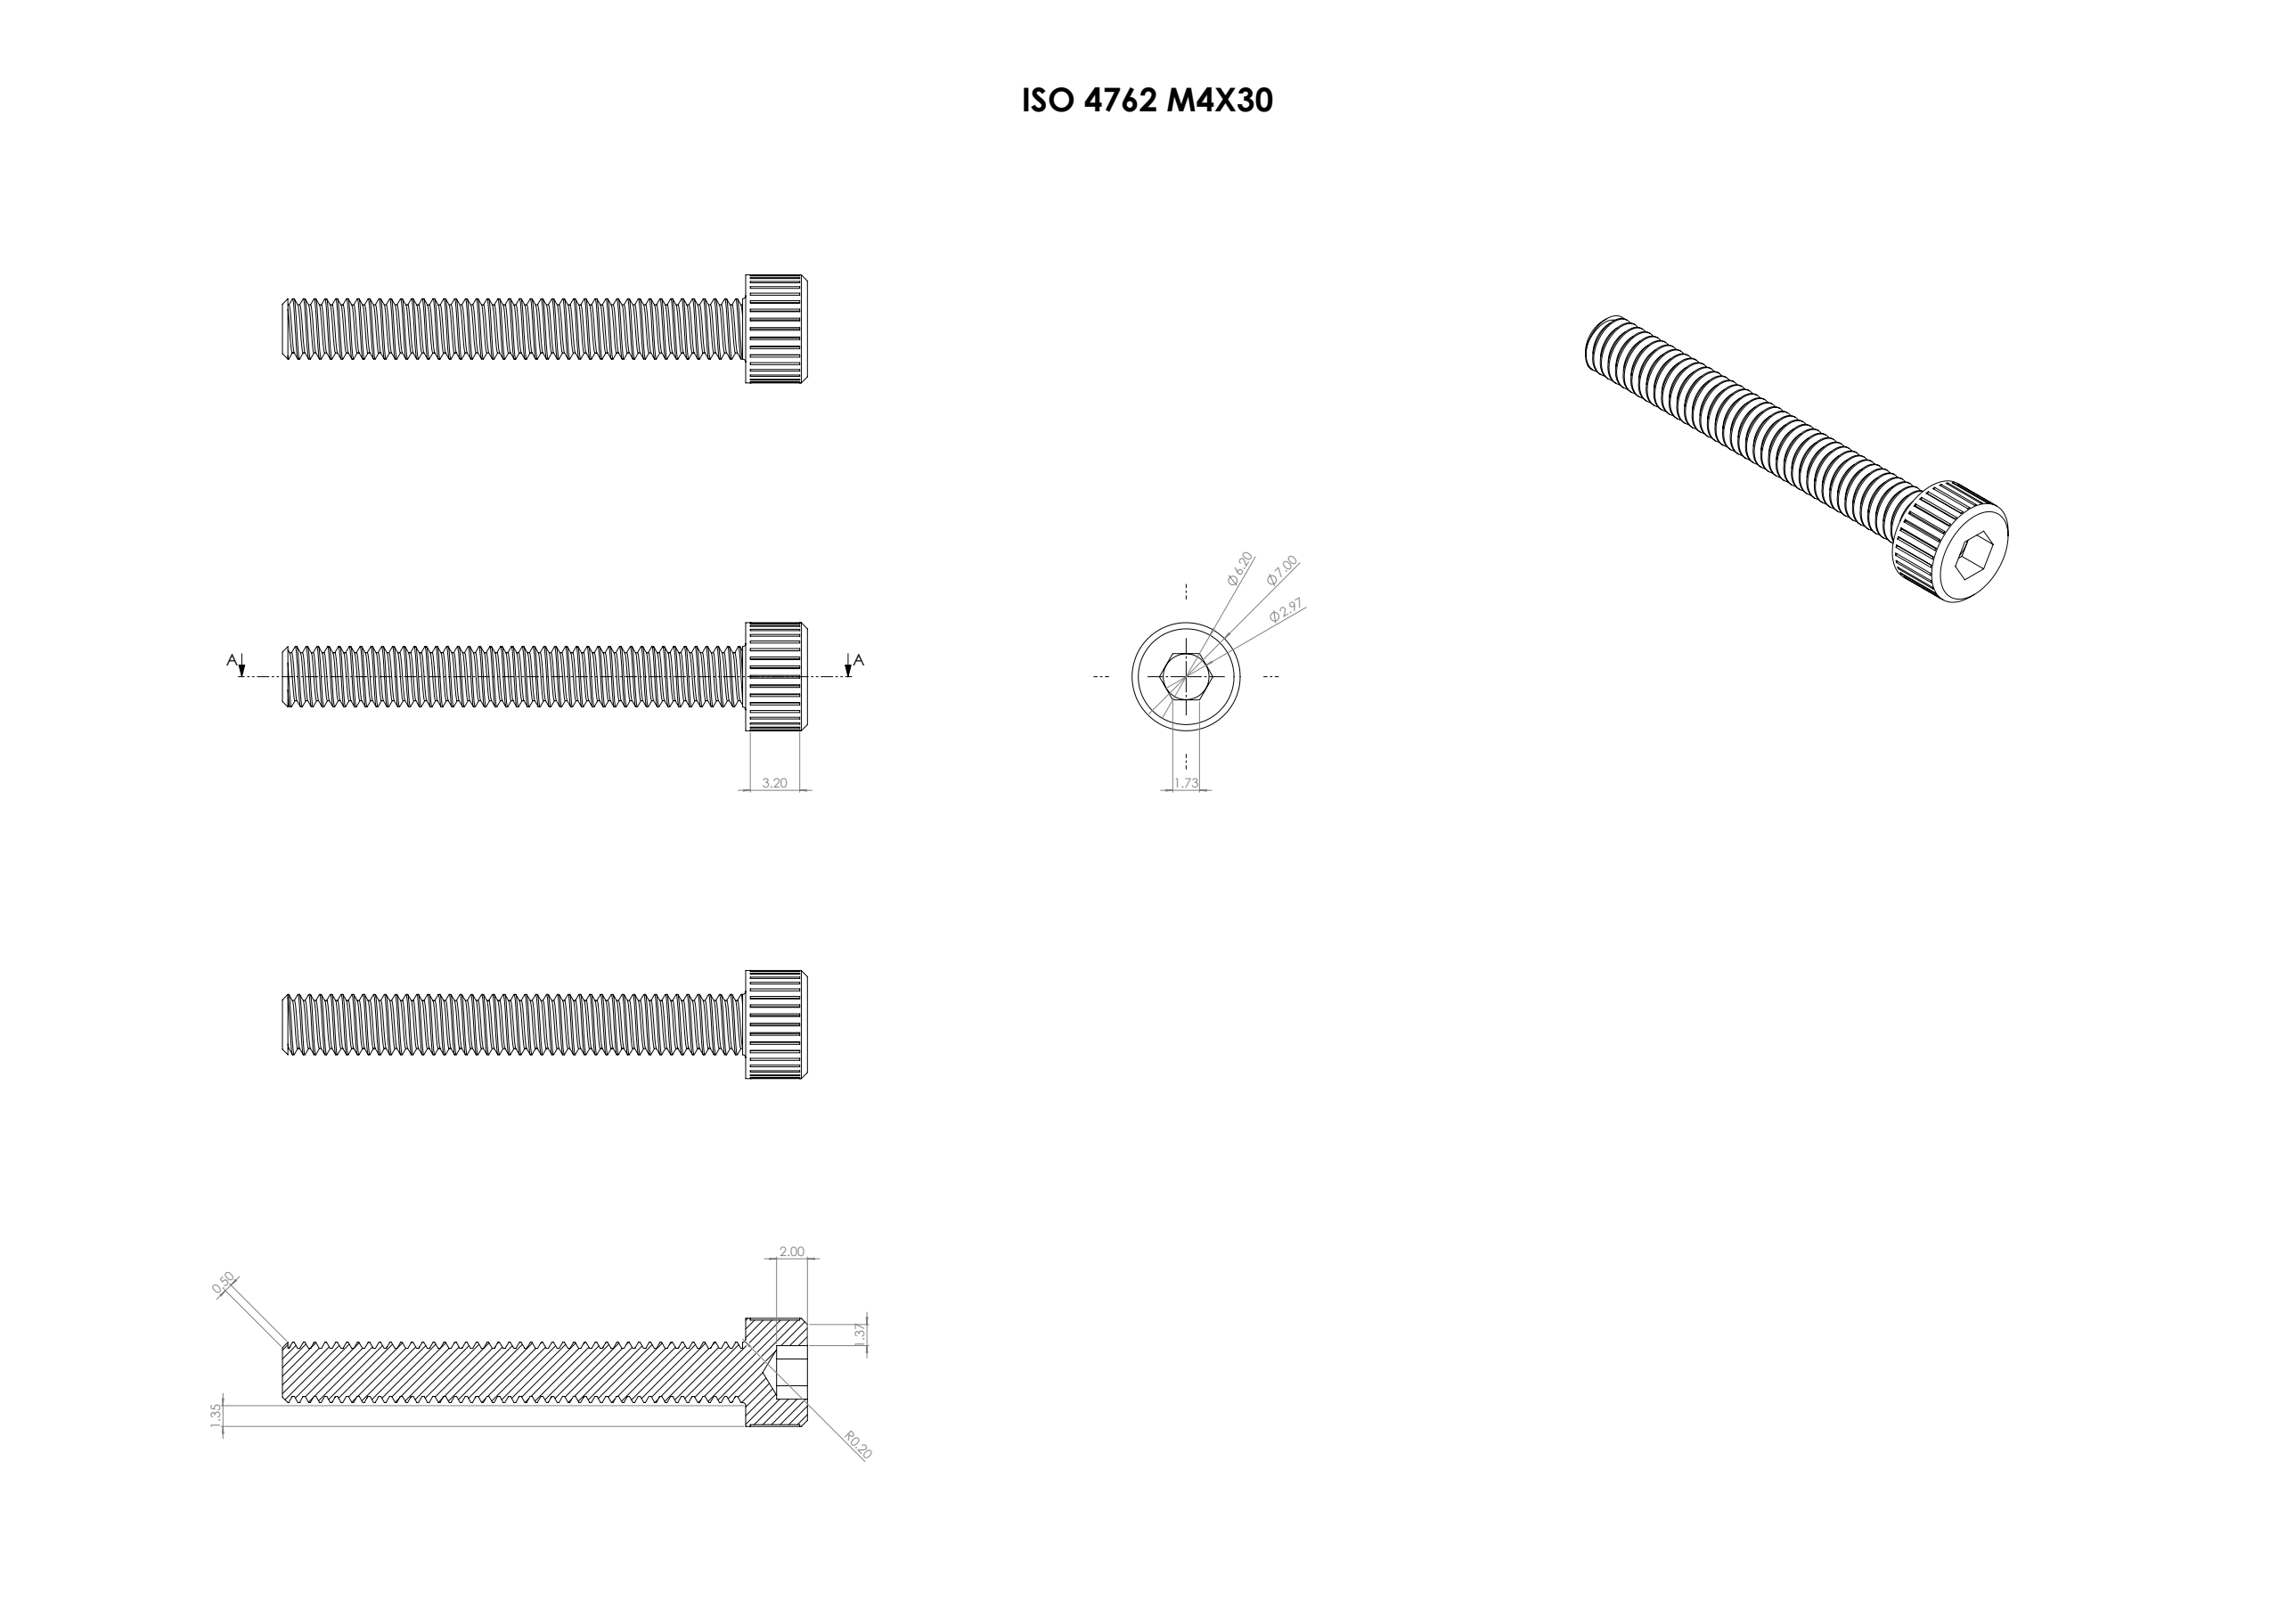
ISO-10303-21;
HEADER;
/* Generated by software containing ST-Developer
 * from STEP Tools, Inc. (www.steptools.com) 
 */

FILE_DESCRIPTION(
/* description */ (''),
/* implementation_level */ '2;1');

FILE_NAME(
/* name */ '14_ISO_4762_M4x30.step',
/* time_stamp */ '2026-10-21T01:56:51-07:00',
/* author */ (''),
/* organization */ (''),
/* preprocessor_version */ 'ST-DEVELOPER v20.2',
/* originating_system */ 'Autodesk Translation Framework v15.15.0.0',
/* authorisation */ '');

FILE_SCHEMA (('AUTOMOTIVE_DESIGN { 1 0 10303 214 3 1 1 }'));
ENDSEC;

DATA;
#10=MECHANICAL_DESIGN_GEOMETRIC_PRESENTATION_REPRESENTATION('',(#281),#82384);
#160=TOROIDAL_SURFACE('',#32201,2.154,0.2);
#243=SHAPE_REPRESENTATION_RELATIONSHIP('SRR','None',#82477,#262);
#262=ADVANCED_BREP_SHAPE_REPRESENTATION('',(#300),#82376);
#281=STYLED_ITEM('',(#82638),#300);
#300=MANIFOLD_SOLID_BREP('Body1',#30672);
#422=B_SPLINE_SURFACE_WITH_KNOTS('',3,3,((#52834,#52835,#52836,#52837,#52838,
#52839,#52840,#52841,#52842,#52843,#52844,#52845,#52846,#52847,#52848,#52849,
#52850,#52851,#52852,#52853,#52854,#52855,#52856,#52857,#52858,#52859,#52860,
#52861,#52862,#52863,#52864,#52865,#52866,#52867,#52868,#52869,#52870,#52871,
#52872,#52873,#52874,#52875,#52876,#52877,#52878,#52879,#52880,#52881,#52882,
#52883,#52884,#52885,#52886,#52887,#52888,#52889,#52890,#52891,#52892,#52893,
#52894,#52895,#52896,#52897,#52898,#52899,#52900,#52901,#52902,#52903,#52904,
#52905,#52906,#52907,#52908,#52909,#52910,#52911,#52912,#52913,#52914,#52915,
#52916,#52917,#52918,#52919,#52920,#52921,#52922,#52923,#52924,#52925,#52926,
#52927,#52928,#52929,#52930,#52931,#52932,#52933,#52934,#52935,#52936,#52937,
#52938,#52939,#52940,#52941,#52942,#52943,#52944,#52945,#52946,#52947,#52948,
#52949,#52950,#52951,#52952,#52953,#52954,#52955,#52956,#52957,#52958,#52959,
#52960,#52961,#52962,#52963,#52964,#52965,#52966,#52967,#52968,#52969,#52970,
#52971,#52972,#52973,#52974,#52975,#52976,#52977,#52978,#52979,#52980,#52981,
#52982,#52983,#52984,#52985,#52986,#52987,#52988,#52989,#52990,#52991,#52992,
#52993,#52994,#52995,#52996,#52997,#52998,#52999,#53000,#53001,#53002,#53003,
#53004,#53005,#53006,#53007,#53008,#53009,#53010,#53011,#53012,#53013,#53014,
#53015,#53016,#53017,#53018,#53019,#53020,#53021,#53022,#53023,#53024,#53025,
#53026,#53027,#53028,#53029,#53030,#53031,#53032,#53033,#53034,#53035,#53036,
#53037,#53038,#53039,#53040,#53041,#53042,#53043,#53044,#53045,#53046,#53047,
#53048,#53049,#53050,#53051,#53052,#53053,#53054,#53055,#53056,#53057,#53058,
#53059,#53060,#53061,#53062,#53063,#53064,#53065,#53066,#53067,#53068,#53069,
#53070,#53071,#53072,#53073,#53074,#53075,#53076,#53077,#53078,#53079,#53080,
#53081,#53082,#53083,#53084,#53085,#53086,#53087,#53088,#53089,#53090,#53091,
#53092,#53093,#53094,#53095,#53096,#53097,#53098,#53099,#53100,#53101,#53102,
#53103),(#53104,#53105,#53106,#53107,#53108,#53109,#53110,#53111,#53112,
#53113,#53114,#53115,#53116,#53117,#53118,#53119,#53120,#53121,#53122,#53123,
#53124,#53125,#53126,#53127,#53128,#53129,#53130,#53131,#53132,#53133,#53134,
#53135,#53136,#53137,#53138,#53139,#53140,#53141,#53142,#53143,#53144,#53145,
#53146,#53147,#53148,#53149,#53150,#53151,#53152,#53153,#53154,#53155,#53156,
#53157,#53158,#53159,#53160,#53161,#53162,#53163,#53164,#53165,#53166,#53167,
#53168,#53169,#53170,#53171,#53172,#53173,#53174,#53175,#53176,#53177,#53178,
#53179,#53180,#53181,#53182,#53183,#53184,#53185,#53186,#53187,#53188,#53189,
#53190,#53191,#53192,#53193,#53194,#53195,#53196,#53197,#53198,#53199,#53200,
#53201,#53202,#53203,#53204,#53205,#53206,#53207,#53208,#53209,#53210,#53211,
#53212,#53213,#53214,#53215,#53216,#53217,#53218,#53219,#53220,#53221,#53222,
#53223,#53224,#53225,#53226,#53227,#53228,#53229,#53230,#53231,#53232,#53233,
#53234,#53235,#53236,#53237,#53238,#53239,#53240,#53241,#53242,#53243,#53244,
#53245,#53246,#53247,#53248,#53249,#53250,#53251,#53252,#53253,#53254,#53255,
#53256,#53257,#53258,#53259,#53260,#53261,#53262,#53263,#53264,#53265,#53266,
#53267,#53268,#53269,#53270,#53271,#53272,#53273,#53274,#53275,#53276,#53277,
#53278,#53279,#53280,#53281,#53282,#53283,#53284,#53285,#53286,#53287,#53288,
#53289,#53290,#53291,#53292,#53293,#53294,#53295,#53296,#53297,#53298,#53299,
#53300,#53301,#53302,#53303,#53304,#53305,#53306,#53307,#53308,#53309,#53310,
#53311,#53312,#53313,#53314,#53315,#53316,#53317,#53318,#53319,#53320,#53321,
#53322,#53323,#53324,#53325,#53326,#53327,#53328,#53329,#53330,#53331,#53332,
#53333,#53334,#53335,#53336,#53337,#53338,#53339,#53340,#53341,#53342,#53343,
#53344,#53345,#53346,#53347,#53348,#53349,#53350,#53351,#53352,#53353,#53354,
#53355,#53356,#53357,#53358,#53359,#53360,#53361,#53362,#53363,#53364,#53365,
#53366,#53367,#53368,#53369,#53370,#53371,#53372,#53373),(#53374,#53375,
#53376,#53377,#53378,#53379,#53380,#53381,#53382,#53383,#53384,#53385,#53386,
#53387,#53388,#53389,#53390,#53391,#53392,#53393,#53394,#53395,#53396,#53397,
#53398,#53399,#53400,#53401,#53402,#53403,#53404,#53405,#53406,#53407,#53408,
#53409,#53410,#53411,#53412,#53413,#53414,#53415,#53416,#53417,#53418,#53419,
#53420,#53421,#53422,#53423,#53424,#53425,#53426,#53427,#53428,#53429,#53430,
#53431,#53432,#53433,#53434,#53435,#53436,#53437,#53438,#53439,#53440,#53441,
#53442,#53443,#53444,#53445,#53446,#53447,#53448,#53449,#53450,#53451,#53452,
#53453,#53454,#53455,#53456,#53457,#53458,#53459,#53460,#53461,#53462,#53463,
#53464,#53465,#53466,#53467,#53468,#53469,#53470,#53471,#53472,#53473,#53474,
#53475,#53476,#53477,#53478,#53479,#53480,#53481,#53482,#53483,#53484,#53485,
#53486,#53487,#53488,#53489,#53490,#53491,#53492,#53493,#53494,#53495,#53496,
#53497,#53498,#53499,#53500,#53501,#53502,#53503,#53504,#53505,#53506,#53507,
#53508,#53509,#53510,#53511,#53512,#53513,#53514,#53515,#53516,#53517,#53518,
#53519,#53520,#53521,#53522,#53523,#53524,#53525,#53526,#53527,#53528,#53529,
#53530,#53531,#53532,#53533,#53534,#53535,#53536,#53537,#53538,#53539,#53540,
#53541,#53542,#53543,#53544,#53545,#53546,#53547,#53548,#53549,#53550,#53551,
#53552,#53553,#53554,#53555,#53556,#53557,#53558,#53559,#53560,#53561,#53562,
#53563,#53564,#53565,#53566,#53567,#53568,#53569,#53570,#53571,#53572,#53573,
#53574,#53575,#53576,#53577,#53578,#53579,#53580,#53581,#53582,#53583,#53584,
#53585,#53586,#53587,#53588,#53589,#53590,#53591,#53592,#53593,#53594,#53595,
#53596,#53597,#53598,#53599,#53600,#53601,#53602,#53603,#53604,#53605,#53606,
#53607,#53608,#53609,#53610,#53611,#53612,#53613,#53614,#53615,#53616,#53617,
#53618,#53619,#53620,#53621,#53622,#53623,#53624,#53625,#53626,#53627,#53628,
#53629,#53630,#53631,#53632,#53633,#53634,#53635,#53636,#53637,#53638,#53639,
#53640,#53641,#53642,#53643),(#53644,#53645,#53646,#53647,#53648,#53649,
#53650,#53651,#53652,#53653,#53654,#53655,#53656,#53657,#53658,#53659,#53660,
#53661,#53662,#53663,#53664,#53665,#53666,#53667,#53668,#53669,#53670,#53671,
#53672,#53673,#53674,#53675,#53676,#53677,#53678,#53679,#53680,#53681,#53682,
#53683,#53684,#53685,#53686,#53687,#53688,#53689,#53690,#53691,#53692,#53693,
#53694,#53695,#53696,#53697,#53698,#53699,#53700,#53701,#53702,#53703,#53704,
#53705,#53706,#53707,#53708,#53709,#53710,#53711,#53712,#53713,#53714,#53715,
#53716,#53717,#53718,#53719,#53720,#53721,#53722,#53723,#53724,#53725,#53726,
#53727,#53728,#53729,#53730,#53731,#53732,#53733,#53734,#53735,#53736,#53737,
#53738,#53739,#53740,#53741,#53742,#53743,#53744,#53745,#53746,#53747,#53748,
#53749,#53750,#53751,#53752,#53753,#53754,#53755,#53756,#53757,#53758,#53759,
#53760,#53761,#53762,#53763,#53764,#53765,#53766,#53767,#53768,#53769,#53770,
#53771,#53772,#53773,#53774,#53775,#53776,#53777,#53778,#53779,#53780,#53781,
#53782,#53783,#53784,#53785,#53786,#53787,#53788,#53789,#53790,#53791,#53792,
#53793,#53794,#53795,#53796,#53797,#53798,#53799,#53800,#53801,#53802,#53803,
#53804,#53805,#53806,#53807,#53808,#53809,#53810,#53811,#53812,#53813,#53814,
#53815,#53816,#53817,#53818,#53819,#53820,#53821,#53822,#53823,#53824,#53825,
#53826,#53827,#53828,#53829,#53830,#53831,#53832,#53833,#53834,#53835,#53836,
#53837,#53838,#53839,#53840,#53841,#53842,#53843,#53844,#53845,#53846,#53847,
#53848,#53849,#53850,#53851,#53852,#53853,#53854,#53855,#53856,#53857,#53858,
#53859,#53860,#53861,#53862,#53863,#53864,#53865,#53866,#53867,#53868,#53869,
#53870,#53871,#53872,#53873,#53874,#53875,#53876,#53877,#53878,#53879,#53880,
#53881,#53882,#53883,#53884,#53885,#53886,#53887,#53888,#53889,#53890,#53891,
#53892,#53893,#53894,#53895,#53896,#53897,#53898,#53899,#53900,#53901,#53902,
#53903,#53904,#53905,#53906,#53907,#53908,#53909,#53910,#53911,#53912,#53913)),
 .UNSPECIFIED.,.F.,.F.,.F.,(4,4),(4,1,1,1,1,1,1,1,1,1,1,1,1,1,1,1,1,1,1,
1,1,1,1,1,1,1,1,1,1,1,1,1,1,1,1,1,1,1,1,1,1,1,1,1,1,1,1,1,1,1,1,1,1,1,1,
1,1,1,1,1,1,1,1,1,1,1,1,1,1,1,1,1,1,1,1,1,1,1,1,1,1,1,1,1,1,1,1,1,1,1,1,
1,1,1,1,1,1,1,1,1,1,1,1,1,1,1,1,1,1,1,1,1,1,1,1,1,1,1,1,1,1,1,1,1,1,1,1,
1,1,1,1,1,1,1,1,1,1,1,1,1,1,1,1,1,1,1,1,1,1,1,1,1,1,1,1,1,1,1,1,1,1,1,1,
1,1,1,1,1,1,1,1,1,1,1,1,1,1,1,1,1,1,1,1,1,1,1,1,1,1,1,1,1,1,1,1,1,1,1,1,
1,1,1,1,1,1,1,1,1,1,1,1,1,1,1,1,1,1,1,1,1,1,1,1,1,1,1,1,1,1,1,1,1,1,1,1,
1,1,1,1,1,1,1,1,1,1,1,1,1,1,1,1,1,1,1,1,1,1,1,1,1,1,1,1,1,1,1,1,4),(0.,
0.0460148164544131),(8.31058692274005,9.30823418142654,10.305881440113,
11.3035286987995,12.301175957486,13.2988232161725,14.296470474859,15.2941177335455,
16.291764992232,17.2894122509185,18.2870595096049,19.2847067682914,20.2823540269779,
21.2800012856644,22.2776485443509,23.2752958030374,24.2729430617239,25.2705903204104,
26.2682375790969,27.2658848377834,28.2635320964698,29.2611793551563,30.2588266138428,
31.2564738725293,32.2541211312158,33.2517683899023,34.2494156485888,35.2470629072753,
36.2447101659618,37.2423574246482,38.2400046833347,39.2376519420212,40.2352992007077,
41.2329464593942,42.2305937180807,43.2282409767672,44.2258882354537,45.2235354941402,
46.2211827528266,47.2188300115131,48.2164772701996,49.2141245288861,50.2117717875726,
51.2094190462591,52.2070663049456,53.2047135636321,54.2023608223186,55.2000080810051,
56.1976553396915,57.195302598378,58.1929498570645,59.190597115751,60.1882443744375,
61.185891633124,62.1835388918105,63.181186150497,64.1788334091835,65.17648066787,
66.1741279265564,67.1717751852429,68.1694224439294,69.1670697026159,70.1647169613024,
71.1623642199889,72.1600114786754,73.1576587373619,74.1553059960484,75.1529532547349,
76.1506005134213,77.1482477721078,78.1458950307943,79.1435422894808,80.1411895481673,
81.1388368068538,82.1364840655403,83.1341313242268,84.1317785829133,85.1294258415997,
86.1270731002862,87.1247203589727,88.1223676176592,89.1200148763457,90.1176621350322,
91.1153093937187,92.1129566524052,93.1106039110917,94.1082511697781,95.1058984284646,
96.1035456871511,97.1011929458376,98.0988402045241,99.0964874632106,100.094134721897,
101.091781980584,102.08942923927,103.087076497957,104.084723756643,105.08237101533,
106.080018274016,107.077665532703,108.075312791389,109.072960050075,110.070607308762,
111.068254567448,112.065901826135,113.063549084821,114.061196343508,115.058843602194,
116.056490860881,117.054138119567,118.051785378254,119.04943263694,120.047079895627,
121.044727154313,122.042374413,123.040021671686,124.037668930373,125.035316189059,
126.032963447746,127.030610706432,128.028257965119,129.025905223805,130.023552482492,
131.021199741178,132.018846999865,133.016494258551,134.014141517238,135.011788775924,
136.009436034611,137.007083293297,138.004730551984,139.00237781067,140.000025069357,
140.997672328043,141.99531958673,142.992966845416,143.990614104103,144.988261362789,
145.985908621476,146.983555880162,147.981203138849,148.978850397535,149.976497656222,
150.974144914908,151.971792173595,152.969439432281,153.967086690968,154.964733949654,
155.96238120834,156.960028467027,157.957675725713,158.9553229844,159.952970243086,
160.950617501773,161.948264760459,162.945912019146,163.943559277832,164.941206536519,
165.938853795205,166.936501053892,167.934148312578,168.931795571265,169.929442829951,
170.927090088638,171.924737347324,172.922384606011,173.920031864697,174.917679123384,
175.91532638207,176.912973640757,177.910620899443,178.90826815813,179.905915416816,
180.903562675503,181.901209934189,182.898857192876,183.896504451562,184.894151710249,
185.891798968935,186.889446227622,187.887093486308,188.884740744995,189.882388003681,
190.880035262368,191.877682521054,192.875329779741,193.872977038427,194.870624297114,
195.8682715558,196.865918814487,197.863566073173,198.86121333186,199.858860590546,
200.856507849232,201.854155107919,202.851802366605,203.849449625292,204.847096883978,
205.844744142665,206.842391401351,207.840038660038,208.837685918724,209.835333177411,
210.832980436097,211.830627694784,212.82827495347,213.825922212157,214.823569470843,
215.82121672953,216.818863988216,217.816511246903,218.814158505589,219.811805764276,
220.809453022962,221.807100281649,222.804747540335,223.802394799022,224.800042057708,
225.797689316395,226.795336575081,227.792983833768,228.790631092454,229.788278351141,
230.785925609827,231.783572868514,232.7812201272,233.778867385887,234.776514644573,
235.77416190326,236.771809161946,237.769456420633,238.767103679319,239.764750938006,
240.762398196692,241.760045455379,242.757692714065,243.755339972752,244.752987231438,
245.750634490125,246.748281748811,247.745929007497,248.743576266184,249.74122352487,
250.738870783557,251.736518042243,252.73416530093,253.731812559616,254.729459818303,
255.727107076989,256.724754335676,257.722401594362,258.720048853049,259.717696111735,
260.715343370422,261.712990629108,262.710637887795,263.708285146481,264.705932405168,
265.703579663854,266.701226922541,267.698874181227,268.696521439914,269.6941686986,
270.691815957287,271.689463215973,272.68711047466,273.684757733346,274.682404992033),
 .UNSPECIFIED.);
#423=B_SPLINE_SURFACE_WITH_KNOTS('',3,3,((#54128,#54129,#54130,#54131,#54132,
#54133,#54134,#54135,#54136,#54137,#54138,#54139,#54140,#54141,#54142,#54143,
#54144,#54145,#54146,#54147,#54148,#54149,#54150,#54151,#54152,#54153,#54154,
#54155,#54156,#54157,#54158,#54159,#54160,#54161,#54162,#54163,#54164,#54165,
#54166,#54167,#54168,#54169,#54170,#54171,#54172,#54173,#54174,#54175,#54176,
#54177,#54178,#54179,#54180,#54181,#54182,#54183,#54184,#54185,#54186,#54187,
#54188,#54189,#54190,#54191,#54192,#54193,#54194,#54195,#54196,#54197,#54198,
#54199,#54200,#54201,#54202,#54203,#54204,#54205,#54206,#54207,#54208,#54209,
#54210,#54211,#54212,#54213,#54214,#54215,#54216,#54217,#54218,#54219,#54220,
#54221,#54222,#54223,#54224,#54225,#54226,#54227,#54228,#54229,#54230,#54231,
#54232,#54233,#54234,#54235,#54236,#54237,#54238,#54239,#54240,#54241,#54242,
#54243,#54244,#54245,#54246,#54247,#54248,#54249,#54250,#54251,#54252,#54253,
#54254,#54255,#54256,#54257,#54258,#54259,#54260,#54261,#54262,#54263,#54264,
#54265,#54266,#54267,#54268,#54269,#54270,#54271,#54272,#54273,#54274,#54275,
#54276,#54277,#54278,#54279,#54280,#54281,#54282,#54283,#54284,#54285,#54286,
#54287,#54288,#54289,#54290,#54291,#54292,#54293,#54294,#54295,#54296,#54297,
#54298,#54299,#54300,#54301,#54302,#54303,#54304,#54305,#54306,#54307,#54308,
#54309,#54310,#54311,#54312,#54313,#54314,#54315,#54316,#54317,#54318,#54319,
#54320,#54321,#54322,#54323,#54324,#54325,#54326,#54327,#54328,#54329,#54330,
#54331,#54332,#54333,#54334,#54335,#54336,#54337,#54338,#54339,#54340,#54341,
#54342,#54343,#54344,#54345,#54346,#54347,#54348,#54349,#54350,#54351,#54352,
#54353,#54354,#54355,#54356,#54357,#54358,#54359,#54360,#54361,#54362,#54363,
#54364,#54365,#54366,#54367,#54368,#54369,#54370,#54371,#54372,#54373,#54374,
#54375,#54376,#54377,#54378,#54379,#54380,#54381,#54382,#54383,#54384,#54385,
#54386,#54387,#54388,#54389,#54390,#54391,#54392,#54393,#54394,#54395,#54396,
#54397),(#54398,#54399,#54400,#54401,#54402,#54403,#54404,#54405,#54406,
#54407,#54408,#54409,#54410,#54411,#54412,#54413,#54414,#54415,#54416,#54417,
#54418,#54419,#54420,#54421,#54422,#54423,#54424,#54425,#54426,#54427,#54428,
#54429,#54430,#54431,#54432,#54433,#54434,#54435,#54436,#54437,#54438,#54439,
#54440,#54441,#54442,#54443,#54444,#54445,#54446,#54447,#54448,#54449,#54450,
#54451,#54452,#54453,#54454,#54455,#54456,#54457,#54458,#54459,#54460,#54461,
#54462,#54463,#54464,#54465,#54466,#54467,#54468,#54469,#54470,#54471,#54472,
#54473,#54474,#54475,#54476,#54477,#54478,#54479,#54480,#54481,#54482,#54483,
#54484,#54485,#54486,#54487,#54488,#54489,#54490,#54491,#54492,#54493,#54494,
#54495,#54496,#54497,#54498,#54499,#54500,#54501,#54502,#54503,#54504,#54505,
#54506,#54507,#54508,#54509,#54510,#54511,#54512,#54513,#54514,#54515,#54516,
#54517,#54518,#54519,#54520,#54521,#54522,#54523,#54524,#54525,#54526,#54527,
#54528,#54529,#54530,#54531,#54532,#54533,#54534,#54535,#54536,#54537,#54538,
#54539,#54540,#54541,#54542,#54543,#54544,#54545,#54546,#54547,#54548,#54549,
#54550,#54551,#54552,#54553,#54554,#54555,#54556,#54557,#54558,#54559,#54560,
#54561,#54562,#54563,#54564,#54565,#54566,#54567,#54568,#54569,#54570,#54571,
#54572,#54573,#54574,#54575,#54576,#54577,#54578,#54579,#54580,#54581,#54582,
#54583,#54584,#54585,#54586,#54587,#54588,#54589,#54590,#54591,#54592,#54593,
#54594,#54595,#54596,#54597,#54598,#54599,#54600,#54601,#54602,#54603,#54604,
#54605,#54606,#54607,#54608,#54609,#54610,#54611,#54612,#54613,#54614,#54615,
#54616,#54617,#54618,#54619,#54620,#54621,#54622,#54623,#54624,#54625,#54626,
#54627,#54628,#54629,#54630,#54631,#54632,#54633,#54634,#54635,#54636,#54637,
#54638,#54639,#54640,#54641,#54642,#54643,#54644,#54645,#54646,#54647,#54648,
#54649,#54650,#54651,#54652,#54653,#54654,#54655,#54656,#54657,#54658,#54659,
#54660,#54661,#54662,#54663,#54664,#54665,#54666,#54667),(#54668,#54669,
#54670,#54671,#54672,#54673,#54674,#54675,#54676,#54677,#54678,#54679,#54680,
#54681,#54682,#54683,#54684,#54685,#54686,#54687,#54688,#54689,#54690,#54691,
#54692,#54693,#54694,#54695,#54696,#54697,#54698,#54699,#54700,#54701,#54702,
#54703,#54704,#54705,#54706,#54707,#54708,#54709,#54710,#54711,#54712,#54713,
#54714,#54715,#54716,#54717,#54718,#54719,#54720,#54721,#54722,#54723,#54724,
#54725,#54726,#54727,#54728,#54729,#54730,#54731,#54732,#54733,#54734,#54735,
#54736,#54737,#54738,#54739,#54740,#54741,#54742,#54743,#54744,#54745,#54746,
#54747,#54748,#54749,#54750,#54751,#54752,#54753,#54754,#54755,#54756,#54757,
#54758,#54759,#54760,#54761,#54762,#54763,#54764,#54765,#54766,#54767,#54768,
#54769,#54770,#54771,#54772,#54773,#54774,#54775,#54776,#54777,#54778,#54779,
#54780,#54781,#54782,#54783,#54784,#54785,#54786,#54787,#54788,#54789,#54790,
#54791,#54792,#54793,#54794,#54795,#54796,#54797,#54798,#54799,#54800,#54801,
#54802,#54803,#54804,#54805,#54806,#54807,#54808,#54809,#54810,#54811,#54812,
#54813,#54814,#54815,#54816,#54817,#54818,#54819,#54820,#54821,#54822,#54823,
#54824,#54825,#54826,#54827,#54828,#54829,#54830,#54831,#54832,#54833,#54834,
#54835,#54836,#54837,#54838,#54839,#54840,#54841,#54842,#54843,#54844,#54845,
#54846,#54847,#54848,#54849,#54850,#54851,#54852,#54853,#54854,#54855,#54856,
#54857,#54858,#54859,#54860,#54861,#54862,#54863,#54864,#54865,#54866,#54867,
#54868,#54869,#54870,#54871,#54872,#54873,#54874,#54875,#54876,#54877,#54878,
#54879,#54880,#54881,#54882,#54883,#54884,#54885,#54886,#54887,#54888,#54889,
#54890,#54891,#54892,#54893,#54894,#54895,#54896,#54897,#54898,#54899,#54900,
#54901,#54902,#54903,#54904,#54905,#54906,#54907,#54908,#54909,#54910,#54911,
#54912,#54913,#54914,#54915,#54916,#54917,#54918,#54919,#54920,#54921,#54922,
#54923,#54924,#54925,#54926,#54927,#54928,#54929,#54930,#54931,#54932,#54933,
#54934,#54935,#54936,#54937),(#54938,#54939,#54940,#54941,#54942,#54943,
#54944,#54945,#54946,#54947,#54948,#54949,#54950,#54951,#54952,#54953,#54954,
#54955,#54956,#54957,#54958,#54959,#54960,#54961,#54962,#54963,#54964,#54965,
#54966,#54967,#54968,#54969,#54970,#54971,#54972,#54973,#54974,#54975,#54976,
#54977,#54978,#54979,#54980,#54981,#54982,#54983,#54984,#54985,#54986,#54987,
#54988,#54989,#54990,#54991,#54992,#54993,#54994,#54995,#54996,#54997,#54998,
#54999,#55000,#55001,#55002,#55003,#55004,#55005,#55006,#55007,#55008,#55009,
#55010,#55011,#55012,#55013,#55014,#55015,#55016,#55017,#55018,#55019,#55020,
#55021,#55022,#55023,#55024,#55025,#55026,#55027,#55028,#55029,#55030,#55031,
#55032,#55033,#55034,#55035,#55036,#55037,#55038,#55039,#55040,#55041,#55042,
#55043,#55044,#55045,#55046,#55047,#55048,#55049,#55050,#55051,#55052,#55053,
#55054,#55055,#55056,#55057,#55058,#55059,#55060,#55061,#55062,#55063,#55064,
#55065,#55066,#55067,#55068,#55069,#55070,#55071,#55072,#55073,#55074,#55075,
#55076,#55077,#55078,#55079,#55080,#55081,#55082,#55083,#55084,#55085,#55086,
#55087,#55088,#55089,#55090,#55091,#55092,#55093,#55094,#55095,#55096,#55097,
#55098,#55099,#55100,#55101,#55102,#55103,#55104,#55105,#55106,#55107,#55108,
#55109,#55110,#55111,#55112,#55113,#55114,#55115,#55116,#55117,#55118,#55119,
#55120,#55121,#55122,#55123,#55124,#55125,#55126,#55127,#55128,#55129,#55130,
#55131,#55132,#55133,#55134,#55135,#55136,#55137,#55138,#55139,#55140,#55141,
#55142,#55143,#55144,#55145,#55146,#55147,#55148,#55149,#55150,#55151,#55152,
#55153,#55154,#55155,#55156,#55157,#55158,#55159,#55160,#55161,#55162,#55163,
#55164,#55165,#55166,#55167,#55168,#55169,#55170,#55171,#55172,#55173,#55174,
#55175,#55176,#55177,#55178,#55179,#55180,#55181,#55182,#55183,#55184,#55185,
#55186,#55187,#55188,#55189,#55190,#55191,#55192,#55193,#55194,#55195,#55196,
#55197,#55198,#55199,#55200,#55201,#55202,#55203,#55204,#55205,#55206,#55207)),
 .UNSPECIFIED.,.F.,.F.,.F.,(4,4),(4,1,1,1,1,1,1,1,1,1,1,1,1,1,1,1,1,1,1,
1,1,1,1,1,1,1,1,1,1,1,1,1,1,1,1,1,1,1,1,1,1,1,1,1,1,1,1,1,1,1,1,1,1,1,1,
1,1,1,1,1,1,1,1,1,1,1,1,1,1,1,1,1,1,1,1,1,1,1,1,1,1,1,1,1,1,1,1,1,1,1,1,
1,1,1,1,1,1,1,1,1,1,1,1,1,1,1,1,1,1,1,1,1,1,1,1,1,1,1,1,1,1,1,1,1,1,1,1,
1,1,1,1,1,1,1,1,1,1,1,1,1,1,1,1,1,1,1,1,1,1,1,1,1,1,1,1,1,1,1,1,1,1,1,1,
1,1,1,1,1,1,1,1,1,1,1,1,1,1,1,1,1,1,1,1,1,1,1,1,1,1,1,1,1,1,1,1,1,1,1,1,
1,1,1,1,1,1,1,1,1,1,1,1,1,1,1,1,1,1,1,1,1,1,1,1,1,1,1,1,1,1,1,1,1,1,1,1,
1,1,1,1,1,1,1,1,1,1,1,1,1,1,1,1,1,1,1,1,1,1,1,1,1,1,1,1,1,1,1,1,4),(0.,
0.0460148164544131),(11.615421519111,12.6130687777975,13.610716036484,14.6083632951705,
15.606010553857,16.6036578125435,17.60130507123,18.5989523299165,19.596599588603,
20.5942468472894,21.5918941059759,22.5895413646624,23.5871886233489,24.5848358820354,
25.5824831407219,26.5801303994084,27.5777776580949,28.5754249167814,29.5730721754678,
30.5707194341543,31.5683666928408,32.5660139515273,33.5636612102138,34.5613084689003,
35.5589557275868,36.5566029862733,37.5542502449598,38.5518975036462,39.5495447623327,
40.5471920210192,41.5448392797057,42.5424865383922,43.5401337970787,44.5377810557652,
45.5354283144517,46.5330755731381,47.5307228318246,48.5283700905111,49.5260173491976,
50.5236646078841,51.5213118665706,52.5189591252571,53.5166063839436,54.5142536426301,
55.5119009013166,56.509548160003,57.5071954186895,58.504842677376,59.5024899360625,
60.500137194749,61.4977844534355,62.495431712122,63.4930789708085,64.490726229495,
65.4883734881815,66.4860207468679,67.4836680055544,68.4813152642409,69.4789625229274,
70.4766097816139,71.4742570403004,72.4719042989869,73.4695515576734,74.4671988163598,
75.4648460750463,76.4624933337328,77.4601405924193,78.4577878511058,79.4554351097923,
80.4530823684788,81.4507296271653,82.4483768858518,83.4460241445382,84.4436714032247,
85.4413186619112,86.4389659205977,87.4366131792842,88.4342604379707,89.4319076966572,
90.4295549553437,91.4272022140302,92.4248494727166,93.4224967314031,94.4201439900896,
95.4177912487761,96.4154385074626,97.4130857661491,98.4107330248356,99.4083802835221,
100.406027542209,101.403674800895,102.401322059582,103.398969318268,104.396616576955,
105.394263835641,106.391911094327,107.389558353014,108.3872056117,109.384852870387,
110.382500129073,111.38014738776,112.377794646446,113.375441905133,114.373089163819,
115.370736422506,116.368383681192,117.366030939879,118.363678198565,119.361325457252,
120.358972715938,121.356619974625,122.354267233311,123.351914491998,124.349561750684,
125.347209009371,126.344856268057,127.342503526744,128.34015078543,129.337798044117,
130.335445302803,131.33309256149,132.330739820176,133.328387078863,134.326034337549,
135.323681596236,136.321328854922,137.318976113609,138.316623372295,139.314270630982,
140.311917889668,141.309565148355,142.307212407041,143.304859665728,144.302506924414,
145.300154183101,146.297801441787,147.295448700474,148.29309595916,149.290743217847,
150.288390476533,151.286037735219,152.283684993906,153.281332252592,154.278979511279,
155.276626769965,156.274274028652,157.271921287338,158.269568546025,159.267215804711,
160.264863063398,161.262510322084,162.260157580771,163.257804839457,164.255452098144,
165.25309935683,166.250746615517,167.248393874203,168.24604113289,169.243688391576,
170.241335650263,171.238982908949,172.236630167636,173.234277426322,174.231924685009,
175.229571943695,176.227219202382,177.224866461068,178.222513719755,179.220160978441,
180.217808237128,181.215455495814,182.213102754501,183.210750013187,184.208397271874,
185.20604453056,186.203691789247,187.201339047933,188.19898630662,189.196633565306,
190.194280823993,191.191928082679,192.189575341366,193.187222600052,194.184869858739,
195.182517117425,196.180164376111,197.177811634798,198.175458893484,199.173106152171,
200.170753410857,201.168400669544,202.16604792823,203.163695186917,204.161342445603,
205.15898970429,206.156636962976,207.154284221663,208.151931480349,209.149578739036,
210.147225997722,211.144873256409,212.142520515095,213.140167773782,214.137815032468,
215.135462291155,216.133109549841,217.130756808528,218.128404067214,219.126051325901,
220.123698584587,221.121345843274,222.11899310196,223.116640360647,224.114287619333,
225.11193487802,226.109582136706,227.107229395393,228.104876654079,229.102523912766,
230.100171171452,231.097818430139,232.095465688825,233.093112947512,234.090760206198,
235.088407464885,236.086054723571,237.083701982258,238.081349240944,239.078996499631,
240.076643758317,241.074291017004,242.07193827569,243.069585534376,244.067232793063,
245.064880051749,246.062527310436,247.060174569122,248.057821827809,249.055469086495,
250.053116345182,251.050763603868,252.048410862555,253.046058121241,254.043705379928,
255.041352638614,256.038999897301,257.036647155987,258.034294414674,259.03194167336,
260.029588932047,261.027236190733,262.02488344942,263.022530708106,264.020177966793,
265.017825225479,266.015472484166,267.013119742852,268.010767001539,269.008414260225,
270.006061518912,271.003708777598,272.001356036285,272.999003294971,273.996650553658,
274.994297812344,275.991945071031,276.989592329717,277.987239588404),
 .UNSPECIFIED.);
#578=CYLINDRICAL_SURFACE('',#32108,1.954);
#579=CYLINDRICAL_SURFACE('',#32110,1.954);
#580=CYLINDRICAL_SURFACE('',#32111,1.954);
#581=CYLINDRICAL_SURFACE('',#32112,1.954);
#582=CYLINDRICAL_SURFACE('',#32113,1.954);
#583=CYLINDRICAL_SURFACE('',#32114,1.954);
#584=CYLINDRICAL_SURFACE('',#32115,1.954);
#585=CYLINDRICAL_SURFACE('',#32116,1.954);
#586=CYLINDRICAL_SURFACE('',#32117,1.954);
#587=CYLINDRICAL_SURFACE('',#32118,1.954);
#588=CYLINDRICAL_SURFACE('',#32119,1.954);
#589=CYLINDRICAL_SURFACE('',#32120,1.954);
#590=CYLINDRICAL_SURFACE('',#32121,1.954);
#591=CYLINDRICAL_SURFACE('',#32122,1.954);
#592=CYLINDRICAL_SURFACE('',#32123,1.954);
#593=CYLINDRICAL_SURFACE('',#32124,1.954);
#594=CYLINDRICAL_SURFACE('',#32125,1.954);
#595=CYLINDRICAL_SURFACE('',#32126,1.954);
#596=CYLINDRICAL_SURFACE('',#32127,1.954);
#597=CYLINDRICAL_SURFACE('',#32128,1.954);
#598=CYLINDRICAL_SURFACE('',#32129,1.954);
#599=CYLINDRICAL_SURFACE('',#32130,1.954);
#600=CYLINDRICAL_SURFACE('',#32131,1.954);
#601=CYLINDRICAL_SURFACE('',#32132,1.954);
#602=CYLINDRICAL_SURFACE('',#32133,1.954);
#603=CYLINDRICAL_SURFACE('',#32134,1.954);
#604=CYLINDRICAL_SURFACE('',#32135,1.954);
#605=CYLINDRICAL_SURFACE('',#32136,1.954);
#606=CYLINDRICAL_SURFACE('',#32137,1.954);
#607=CYLINDRICAL_SURFACE('',#32138,1.954);
#608=CYLINDRICAL_SURFACE('',#32139,1.954);
#609=CYLINDRICAL_SURFACE('',#32140,1.954);
#610=CYLINDRICAL_SURFACE('',#32141,1.954);
#611=CYLINDRICAL_SURFACE('',#32142,1.954);
#612=CYLINDRICAL_SURFACE('',#32143,1.954);
#613=CYLINDRICAL_SURFACE('',#32144,1.954);
#614=CYLINDRICAL_SURFACE('',#32145,1.954);
#615=CYLINDRICAL_SURFACE('',#32146,1.954);
#616=CYLINDRICAL_SURFACE('',#32147,1.954);
#617=CYLINDRICAL_SURFACE('',#32148,1.954);
#618=CYLINDRICAL_SURFACE('',#32149,1.954);
#619=CYLINDRICAL_SURFACE('',#32150,1.954);
#620=CYLINDRICAL_SURFACE('',#32151,1.5555);
#621=CYLINDRICAL_SURFACE('',#32153,1.5555);
#622=CYLINDRICAL_SURFACE('',#32154,1.5555);
#623=CYLINDRICAL_SURFACE('',#32155,1.5555);
#624=CYLINDRICAL_SURFACE('',#32156,1.5555);
#625=CYLINDRICAL_SURFACE('',#32157,1.5555);
#626=CYLINDRICAL_SURFACE('',#32158,1.5555);
#627=CYLINDRICAL_SURFACE('',#32159,1.5555);
#628=CYLINDRICAL_SURFACE('',#32160,1.5555);
#629=CYLINDRICAL_SURFACE('',#32161,1.5555);
#630=CYLINDRICAL_SURFACE('',#32162,1.5555);
#631=CYLINDRICAL_SURFACE('',#32163,1.5555);
#632=CYLINDRICAL_SURFACE('',#32164,1.5555);
#633=CYLINDRICAL_SURFACE('',#32165,1.5555);
#634=CYLINDRICAL_SURFACE('',#32166,1.5555);
#635=CYLINDRICAL_SURFACE('',#32167,1.5555);
#636=CYLINDRICAL_SURFACE('',#32168,1.5555);
#637=CYLINDRICAL_SURFACE('',#32169,1.5555);
#638=CYLINDRICAL_SURFACE('',#32170,1.5555);
#639=CYLINDRICAL_SURFACE('',#32171,1.5555);
#640=CYLINDRICAL_SURFACE('',#32172,1.5555);
#641=CYLINDRICAL_SURFACE('',#32173,1.5555);
#642=CYLINDRICAL_SURFACE('',#32174,1.5555);
#643=CYLINDRICAL_SURFACE('',#32175,1.5555);
#644=CYLINDRICAL_SURFACE('',#32176,1.5555);
#645=CYLINDRICAL_SURFACE('',#32177,1.5555);
#646=CYLINDRICAL_SURFACE('',#32178,1.5555);
#647=CYLINDRICAL_SURFACE('',#32179,1.5555);
#648=CYLINDRICAL_SURFACE('',#32180,1.5555);
#649=CYLINDRICAL_SURFACE('',#32181,1.5555);
#650=CYLINDRICAL_SURFACE('',#32182,1.5555);
#651=CYLINDRICAL_SURFACE('',#32183,1.5555);
#652=CYLINDRICAL_SURFACE('',#32184,1.5555);
#653=CYLINDRICAL_SURFACE('',#32185,1.5555);
#654=CYLINDRICAL_SURFACE('',#32186,1.5555);
#655=CYLINDRICAL_SURFACE('',#32187,1.5555);
#656=CYLINDRICAL_SURFACE('',#32188,1.5555);
#657=CYLINDRICAL_SURFACE('',#32189,1.5555);
#658=CYLINDRICAL_SURFACE('',#32190,1.5555);
#659=CYLINDRICAL_SURFACE('',#32191,1.5555);
#660=CYLINDRICAL_SURFACE('',#32192,1.5555);
#661=CYLINDRICAL_SURFACE('',#32193,1.5555);
#662=CYLINDRICAL_SURFACE('',#32200,1.5555);
#663=CYLINDRICAL_SURFACE('',#32206,1.954);
#664=CYLINDRICAL_SURFACE('',#32439,3.5);
#1542=CIRCLE('',#32109,1.954);
#1543=CIRCLE('',#32152,1.5555);
#1544=CIRCLE('',#32195,1.954);
#1545=CIRCLE('',#32197,1.954);
#1546=CIRCLE('',#32198,1.954);
#1547=CIRCLE('',#32199,1.5555);
#1548=CIRCLE('',#32202,1.954);
#1549=CIRCLE('',#32203,0.2);
#1550=CIRCLE('',#32204,2.154);
#1551=CIRCLE('',#32205,1.954);
#1552=CIRCLE('',#32208,3.5);
#1553=CIRCLE('',#32211,3.5);
#1554=CIRCLE('',#32214,3.5);
#1555=CIRCLE('',#32217,3.5);
#1556=CIRCLE('',#32220,3.5);
#1557=CIRCLE('',#32223,3.5);
#1558=CIRCLE('',#32226,3.5);
#1559=CIRCLE('',#32229,3.5);
#1560=CIRCLE('',#32232,3.5);
#1561=CIRCLE('',#32235,3.5);
#1562=CIRCLE('',#32238,3.5);
#1563=CIRCLE('',#32241,3.5);
#1564=CIRCLE('',#32244,3.5);
#1565=CIRCLE('',#32247,3.5);
#1566=CIRCLE('',#32250,3.5);
#1567=CIRCLE('',#32253,3.5);
#1568=CIRCLE('',#32256,3.5);
#1569=CIRCLE('',#32259,3.5);
#1570=CIRCLE('',#32262,3.5);
#1571=CIRCLE('',#32265,3.5);
#1572=CIRCLE('',#32268,3.5);
#1573=CIRCLE('',#32271,3.5);
#1574=CIRCLE('',#32274,3.5);
#1575=CIRCLE('',#32277,3.5);
#1576=CIRCLE('',#32280,3.5);
#1577=CIRCLE('',#32283,3.5);
#1578=CIRCLE('',#32286,3.5);
#1579=CIRCLE('',#32289,3.5);
#1580=CIRCLE('',#32292,3.5);
#1581=CIRCLE('',#32295,3.5);
#1582=CIRCLE('',#32298,3.5);
#1583=CIRCLE('',#32301,3.5);
#1584=CIRCLE('',#32304,3.5);
#1585=CIRCLE('',#32307,3.5);
#1586=CIRCLE('',#32310,3.5);
#1587=CIRCLE('',#32313,3.5);
#1588=CIRCLE('',#32314,3.5);
#1589=CIRCLE('',#32317,3.5);
#1590=CIRCLE('',#32318,3.5);
#1591=CIRCLE('',#32321,3.5);
#1592=CIRCLE('',#32324,3.5);
#1593=CIRCLE('',#32327,3.5);
#1594=CIRCLE('',#32330,3.5);
#1595=CIRCLE('',#32333,3.5);
#1596=CIRCLE('',#32336,3.5);
#1597=CIRCLE('',#32339,3.5);
#1598=CIRCLE('',#32342,3.5);
#1599=CIRCLE('',#32345,3.5);
#1600=CIRCLE('',#32348,3.5);
#1601=CIRCLE('',#32351,3.5);
#1602=CIRCLE('',#32354,3.5);
#1603=CIRCLE('',#32357,3.5);
#1604=CIRCLE('',#32360,3.5);
#1605=CIRCLE('',#32363,3.5);
#1606=CIRCLE('',#32366,3.5);
#1607=CIRCLE('',#32369,3.5);
#1608=CIRCLE('',#32372,3.5);
#1609=CIRCLE('',#32375,3.5);
#1610=CIRCLE('',#32378,3.5);
#1611=CIRCLE('',#32381,3.5);
#1612=CIRCLE('',#32384,3.5);
#1613=CIRCLE('',#32387,3.5);
#1614=CIRCLE('',#32390,3.5);
#1615=CIRCLE('',#32393,3.5);
#1616=CIRCLE('',#32396,3.5);
#1617=CIRCLE('',#32399,3.5);
#1618=CIRCLE('',#32402,3.5);
#1619=CIRCLE('',#32405,3.5);
#1620=CIRCLE('',#32408,3.5);
#1621=CIRCLE('',#32411,3.5);
#1622=CIRCLE('',#32414,3.5);
#1623=CIRCLE('',#32417,3.5);
#1624=CIRCLE('',#32420,3.5);
#1625=CIRCLE('',#32423,3.5);
#1626=CIRCLE('',#32426,3.5);
#1627=CIRCLE('',#32428,1.483539833954);
#1628=CIRCLE('',#32437,1.6);
#1629=CIRCLE('',#32440,3.5);
#1630=CIRCLE('',#32442,3.1);
#2039=CONICAL_SURFACE('',#32427,0.75,1.02486043295185);
#2040=CONICAL_SURFACE('',#32438,1.8,0.785398163397448);
#2041=CONICAL_SURFACE('',#32441,3.3,0.785398163397448);
#2375=B_SPLINE_CURVE_WITH_KNOTS('',3,(#49575,#49576,#49577,#49578,#49579,
#49580,#49581,#49582,#49583,#49584),.UNSPECIFIED.,.F.,.F.,(4,3,3,4),(-4.09254174883831,
-3.99058903474596,-2.99294177605947,-2.06514013327809),.UNSPECIFIED.);
#2376=B_SPLINE_CURVE_WITH_KNOTS('',3,(#49587,#49588,#49589,#49590,#49591,
#49592,#49593),.UNSPECIFIED.,.F.,.F.,(4,3,4),(0.,0.997647258686503,1.11419103803015),
 .UNSPECIFIED.);
#2377=B_SPLINE_CURVE_WITH_KNOTS('',3,(#49598,#49599,#49600,#49601,#49602,
#49603,#49604,#49605,#49606,#49607,#49608,#49609,#49610,#49611,#49612,#49613,
#49614,#49615,#49616,#49617,#49618,#49619),.UNSPECIFIED.,.F.,.F.,(4,3,3,
3,3,3,3,4),(-10.3757270560179,-9.97647258686489,-8.9788253281784,-7.98117806949191,
-6.98353081080542,-5.98588355211893,-4.98823629343245,-4.09254174883831),
 .UNSPECIFIED.);
#2378=B_SPLINE_CURVE_WITH_KNOTS('',3,(#49620,#49621,#49622,#49623,#49624,
#49625,#49626,#49627,#49628,#49629,#49630,#49631,#49632,#49633,#49634,#49635,
#49636,#49637,#49638,#49639,#49640,#49641),.UNSPECIFIED.,.F.,.F.,(4,3,3,
3,3,3,3,4),(1.11419103803015,1.99529451737299,2.99294177605948,3.99058903474597,
4.98823629343246,5.98588355211895,6.98353081080544,7.39737634520972),
 .UNSPECIFIED.);
#2379=B_SPLINE_CURVE_WITH_KNOTS('',3,(#49646,#49647,#49648,#49649,#49650,
#49651,#49652,#49653,#49654,#49655,#49656,#49657,#49658,#49659,#49660,#49661,
#49662,#49663,#49664,#49665,#49666,#49667),.UNSPECIFIED.,.F.,.F.,(4,3,3,
3,3,3,3,4),(-16.6589123631975,-15.9623561389838,-14.9647088802973,-13.9670616216108,
-12.9694143629244,-11.9717671042379,-10.9741198455514,-10.3757270560179),
 .UNSPECIFIED.);
#2380=B_SPLINE_CURVE_WITH_KNOTS('',3,(#49668,#49669,#49670,#49671,#49672,
#49673,#49674,#49675,#49676,#49677,#49678,#49679,#49680,#49681,#49682,#49683,
#49684,#49685,#49686,#49687,#49688,#49689),.UNSPECIFIED.,.F.,.F.,(4,3,3,
3,3,3,3,4),(7.39737634520972,7.98117806949192,8.97882532817841,9.97647258686489,
10.9741198455514,11.9717671042379,12.9694143629243,13.6805616523893),
 .UNSPECIFIED.);
#2381=B_SPLINE_CURVE_WITH_KNOTS('',3,(#49694,#49695,#49696,#49697,#49698,
#49699,#49700,#49701,#49702,#49703,#49704,#49705,#49706,#49707,#49708,#49709,
#49710,#49711,#49712,#49713,#49714,#49715),.UNSPECIFIED.,.F.,.F.,(4,3,3,
3,3,3,3,4),(-22.9420976703771,-21.9482396911028,-20.9505924324163,-19.9529451737298,
-18.9552979150433,-17.9576506563568,-16.9600033976703,-16.6589123631975),
 .UNSPECIFIED.);
#2382=B_SPLINE_CURVE_WITH_KNOTS('',3,(#49716,#49717,#49718,#49719,#49720,
#49721,#49722,#49723,#49724,#49725,#49726,#49727,#49728,#49729,#49730,#49731,
#49732,#49733,#49734,#49735,#49736,#49737,#49738,#49739,#49740),
 .UNSPECIFIED.,.F.,.F.,(4,3,3,3,3,3,3,3,4),(13.6805616523893,13.9670616216108,
14.9647088802973,15.9623561389838,16.9600033976703,17.9576506563568,18.9552979150433,
19.9529451737298,19.9637469595689),.UNSPECIFIED.);
#2383=B_SPLINE_CURVE_WITH_KNOTS('',3,(#49745,#49746,#49747,#49748,#49749,
#49750,#49751,#49752,#49753,#49754,#49755,#49756,#49757,#49758,#49759,#49760,
#49761,#49762,#49763,#49764,#49765,#49766,#49767,#49768,#49769),
 .UNSPECIFIED.,.F.,.F.,(4,3,3,3,3,3,3,3,4),(-29.2252829775566,-28.9317705019082,
-27.9341232432217,-26.9364759845352,-25.9388287258487,-24.9411814671622,
-23.9435342084757,-22.9458869497892,-22.9420976703771),.UNSPECIFIED.);
#2384=B_SPLINE_CURVE_WITH_KNOTS('',3,(#49770,#49771,#49772,#49773,#49774,
#49775,#49776,#49777,#49778,#49779,#49780,#49781,#49782,#49783,#49784,#49785,
#49786,#49787,#49788,#49789,#49790,#49791),.UNSPECIFIED.,.F.,.F.,(4,3,3,
3,3,3,3,4),(19.9637469595689,20.9505924324163,21.9482396911028,22.9458869497892,
23.9435342084757,24.9411814671622,25.9388287258487,26.2469322667485),
 .UNSPECIFIED.);
#2385=B_SPLINE_CURVE_WITH_KNOTS('',3,(#49796,#49797,#49798,#49799,#49800,
#49801,#49802,#49803,#49804,#49805,#49806,#49807,#49808,#49809,#49810,#49811,
#49812,#49813,#49814,#49815,#49816,#49817),.UNSPECIFIED.,.F.,.F.,(4,3,3,
3,3,3,3,4),(-35.5084682847363,-34.9176540540271,-33.9200067953406,-32.9223595366541,
-31.9247122779677,-30.9270650192812,-29.9294177605947,-29.2252829775566),
 .UNSPECIFIED.);
#2386=B_SPLINE_CURVE_WITH_KNOTS('',3,(#49818,#49819,#49820,#49821,#49822,
#49823,#49824,#49825,#49826,#49827,#49828,#49829,#49830,#49831,#49832,#49833,
#49834,#49835,#49836,#49837,#49838,#49839),.UNSPECIFIED.,.F.,.F.,(4,3,3,
3,3,3,3,4),(26.2469322667485,26.9364759845352,27.9341232432217,28.9317705019082,
29.9294177605947,30.9270650192812,31.9247122779677,32.5301175739281),
 .UNSPECIFIED.);
#2387=B_SPLINE_CURVE_WITH_KNOTS('',3,(#49844,#49845,#49846,#49847,#49848,
#49849,#49850,#49851,#49852,#49853,#49854,#49855,#49856,#49857,#49858,#49859,
#49860,#49861,#49862,#49863,#49864,#49865),.UNSPECIFIED.,.F.,.F.,(4,3,3,
3,3,3,3,4),(-41.7916535919158,-40.903537606146,-39.9058903474596,-38.9082430887731,
-37.9105958300866,-36.9129485714001,-35.9153013127136,-35.5084682847363),
 .UNSPECIFIED.);
#2388=B_SPLINE_CURVE_WITH_KNOTS('',3,(#49866,#49867,#49868,#49869,#49870,
#49871,#49872,#49873,#49874,#49875,#49876,#49877,#49878,#49879,#49880,#49881,
#49882,#49883,#49884,#49885,#49886,#49887),.UNSPECIFIED.,.F.,.F.,(4,3,3,
3,3,3,3,4),(32.5301175739281,32.9223595366541,33.9200067953406,34.9176540540271,
35.9153013127136,36.9129485714001,37.9105958300866,38.8133028811077),
 .UNSPECIFIED.);
#2389=B_SPLINE_CURVE_WITH_KNOTS('',3,(#49892,#49893,#49894,#49895,#49896,
#49897,#49898,#49899,#49900,#49901,#49902,#49903,#49904,#49905,#49906,#49907,
#49908,#49909,#49910,#49911,#49912,#49913,#49914,#49915,#49916),
 .UNSPECIFIED.,.F.,.F.,(4,3,3,3,3,3,3,3,4),(-48.0748388990954,-47.8870684169515,
-46.889421158265,-45.8917738995785,-44.894126640892,-43.8964793822055,-42.898832123519,
-41.9011848648325,-41.7916535919158),.UNSPECIFIED.);
#2390=B_SPLINE_CURVE_WITH_KNOTS('',3,(#49917,#49918,#49919,#49920,#49921,
#49922,#49923,#49924,#49925,#49926,#49927,#49928,#49929,#49930,#49931,#49932,
#49933,#49934,#49935,#49936,#49937,#49938,#49939,#49940,#49941),
 .UNSPECIFIED.,.F.,.F.,(4,3,3,3,3,3,3,3,4),(38.8133028811077,38.9082430887731,
39.9058903474596,40.9035376061461,41.9011848648326,42.898832123519,43.8964793822055,
44.894126640892,45.0964881882873),.UNSPECIFIED.);
#2391=B_SPLINE_CURVE_WITH_KNOTS('',3,(#49946,#49947,#49948,#49949,#49950,
#49951,#49952,#49953,#49954,#49955,#49956,#49957,#49958,#49959,#49960,#49961,
#49962,#49963,#49964,#49965,#49966,#49967),.UNSPECIFIED.,.F.,.F.,(4,3,3,
3,3,3,3,4),(-54.358024206275,-53.8729519690704,-52.8753047103839,-51.8776574516974,
-50.8800101930109,-49.8823629343244,-48.884715675638,-48.0748388990954),
 .UNSPECIFIED.);
#2392=B_SPLINE_CURVE_WITH_KNOTS('',3,(#49968,#49969,#49970,#49971,#49972,
#49973,#49974,#49975,#49976,#49977,#49978,#49979,#49980,#49981,#49982,#49983,
#49984,#49985,#49986,#49987,#49988,#49989),.UNSPECIFIED.,.F.,.F.,(4,3,3,
3,3,3,3,4),(45.0964881882873,45.8917738995785,46.889421158265,47.8870684169515,
48.884715675638,49.8823629343245,50.880010193011,51.3796734954669),
 .UNSPECIFIED.);
#2393=B_SPLINE_CURVE_WITH_KNOTS('',3,(#49994,#49995,#49996,#49997,#49998,
#49999,#50000,#50001,#50002,#50003,#50004,#50005,#50006,#50007,#50008,#50009,
#50010,#50011,#50012,#50013,#50014,#50015),.UNSPECIFIED.,.F.,.F.,(4,3,3,
3,3,3,3,4),(-60.6412095134546,-59.8588355211893,-58.8611882625028,-57.8635410038164,
-56.8658937451299,-55.8682464864434,-54.8705992277569,-54.358024206275),
 .UNSPECIFIED.);
#2394=B_SPLINE_CURVE_WITH_KNOTS('',3,(#50016,#50017,#50018,#50019,#50020,
#50021,#50022,#50023,#50024,#50025,#50026,#50027,#50028,#50029,#50030,#50031,
#50032,#50033,#50034,#50035,#50036,#50037),.UNSPECIFIED.,.F.,.F.,(4,3,3,
3,3,3,3,4),(51.3796734954669,51.8776574516975,52.8753047103839,53.8729519690704,
54.8705992277569,55.8682464864434,56.8658937451299,57.6628588026465),
 .UNSPECIFIED.);
#2395=B_SPLINE_CURVE_WITH_KNOTS('',3,(#50042,#50043,#50044,#50045,#50046,
#50047,#50048,#50049,#50050,#50051,#50052,#50053,#50054,#50055,#50056,#50057,
#50058,#50059,#50060,#50061,#50062,#50063,#50064,#50065,#50066),
 .UNSPECIFIED.,.F.,.F.,(4,3,3,3,3,3,3,3,4),(-66.9243948206342,-66.8423663319947,
-65.8447190733083,-64.8470718146218,-63.8494245559353,-62.8517772972488,
-61.8541300385623,-60.8564827798758,-60.6412095134546),.UNSPECIFIED.);
#2396=B_SPLINE_CURVE_WITH_KNOTS('',3,(#50067,#50068,#50069,#50070,#50071,
#50072,#50073,#50074,#50075,#50076,#50077,#50078,#50079,#50080,#50081,#50082,
#50083,#50084,#50085,#50086,#50087,#50088,#50089,#50090,#50091),
 .UNSPECIFIED.,.F.,.F.,(4,3,3,3,3,3,3,3,4),(57.6628588026465,57.8635410038164,
58.8611882625029,59.8588355211894,60.8564827798759,61.8541300385624,62.8517772972489,
63.8494245559354,63.946044109826),.UNSPECIFIED.);
#2397=B_SPLINE_CURVE_WITH_KNOTS('',3,(#50096,#50097,#50098,#50099,#50100,
#50101,#50102,#50103,#50104,#50105,#50106,#50107,#50108,#50109,#50110,#50111,
#50112,#50113,#50114,#50115,#50116,#50117),.UNSPECIFIED.,.F.,.F.,(4,3,3,
3,3,3,3,4),(-73.2075801278138,-72.8282498841137,-71.8306026254272,-70.8329553667407,
-69.8353081080542,-68.8376608493677,-67.8400135906812,-66.9243948206342),
 .UNSPECIFIED.);
#2398=B_SPLINE_CURVE_WITH_KNOTS('',3,(#50118,#50119,#50120,#50121,#50122,
#50123,#50124,#50125,#50126,#50127,#50128,#50129,#50130,#50131,#50132,#50133,
#50134,#50135,#50136,#50137,#50138,#50139),.UNSPECIFIED.,.F.,.F.,(4,3,3,
3,3,3,3,4),(63.946044109826,64.8470718146218,65.8447190733083,66.8423663319948,
67.8400135906813,68.8376608493678,69.8353081080543,70.2292294170057),
 .UNSPECIFIED.);
#2399=B_SPLINE_CURVE_WITH_KNOTS('',3,(#50144,#50145,#50146,#50147,#50148,
#50149,#50150,#50151,#50152,#50153,#50154,#50155,#50156,#50157,#50158,#50159,
#50160,#50161,#50162,#50163,#50164,#50165),.UNSPECIFIED.,.F.,.F.,(4,3,3,
3,3,3,3,4),(-79.4907654349934,-78.8141334362326,-77.8164861775462,-76.8188389188597,
-75.8211916601732,-74.8235444014867,-73.8258971428002,-73.2075801278138),
 .UNSPECIFIED.);
#2400=B_SPLINE_CURVE_WITH_KNOTS('',3,(#50166,#50167,#50168,#50169,#50170,
#50171,#50172,#50173,#50174,#50175,#50176,#50177,#50178,#50179,#50180,#50181,
#50182,#50183,#50184,#50185,#50186,#50187),.UNSPECIFIED.,.F.,.F.,(4,3,3,
3,3,3,3,4),(70.2292294170057,70.8329553667407,71.8306026254272,72.8282498841137,
73.8258971428002,74.8235444014867,75.8211916601732,76.5124147241852),
 .UNSPECIFIED.);
#2401=B_SPLINE_CURVE_WITH_KNOTS('',3,(#50192,#50193,#50194,#50195,#50196,
#50197,#50198,#50199,#50200,#50201,#50202,#50203,#50204,#50205,#50206,#50207,
#50208,#50209,#50210,#50211,#50212,#50213),.UNSPECIFIED.,.F.,.F.,(4,3,3,
3,3,3,3,4),(-85.773950742173,-84.8000169883516,-83.8023697296651,-82.8047224709786,
-81.8070752122921,-80.8094279536056,-79.8117806949191,-79.4907654349934),
 .UNSPECIFIED.);
#2402=B_SPLINE_CURVE_WITH_KNOTS('',3,(#50214,#50215,#50216,#50217,#50218,
#50219,#50220,#50221,#50222,#50223,#50224,#50225,#50226,#50227,#50228,#50229,
#50230,#50231,#50232,#50233,#50234,#50235),.UNSPECIFIED.,.F.,.F.,(4,3,3,
3,3,3,3,4),(76.5124147241852,76.8188389188597,77.8164861775462,78.8141334362327,
79.8117806949192,80.8094279536056,81.8070752122921,82.7956000313648),
 .UNSPECIFIED.);
#2403=B_SPLINE_CURVE_WITH_KNOTS('',3,(#50240,#50241,#50242,#50243,#50244,
#50245,#50246,#50247,#50248,#50249,#50250,#50251,#50252,#50253,#50254,#50255,
#50256,#50257,#50258,#50259,#50260,#50261,#50262,#50263,#50264),
 .UNSPECIFIED.,.F.,.F.,(4,3,3,3,3,3,3,3,4),(-92.0571360493526,-91.783547799157,
-90.7859005404705,-89.788253281784,-88.7906060230975,-87.792958764411,-86.7953115057246,
-85.7976642470381,-85.773950742173),.UNSPECIFIED.);
#2404=B_SPLINE_CURVE_WITH_KNOTS('',3,(#50265,#50266,#50267,#50268,#50269,
#50270,#50271,#50272,#50273,#50274,#50275,#50276,#50277,#50278,#50279,#50280,
#50281,#50282,#50283,#50284,#50285,#50286,#50287,#50288,#50289),
 .UNSPECIFIED.,.F.,.F.,(4,3,3,3,3,3,3,3,4),(82.7956000313648,82.8047224709786,
83.8023697296651,84.8000169883516,85.7976642470381,86.7953115057246,87.7929587644111,
88.7906060230976,89.0787853385444),.UNSPECIFIED.);
#2405=B_SPLINE_CURVE_WITH_KNOTS('',3,(#50294,#50295,#50296,#50297,#50298,
#50299,#50300,#50301,#50302,#50303,#50304,#50305,#50306,#50307,#50308,#50309,
#50310,#50311,#50312,#50313,#50314,#50315),.UNSPECIFIED.,.F.,.F.,(4,3,3,
3,3,3,3,4),(-98.3403213565322,-97.7694313512759,-96.7717840925894,-95.774136833903,
-94.7764895752164,-93.77884231653,-92.7811950578435,-92.0571360493526),
 .UNSPECIFIED.);
#2406=B_SPLINE_CURVE_WITH_KNOTS('',3,(#50316,#50317,#50318,#50319,#50320,
#50321,#50322,#50323,#50324,#50325,#50326,#50327,#50328,#50329,#50330,#50331,
#50332,#50333,#50334,#50335,#50336,#50337),.UNSPECIFIED.,.F.,.F.,(4,3,3,
3,3,3,3,4),(89.0787853385444,89.7882532817841,90.7859005404705,91.783547799157,
92.7811950578435,93.77884231653,94.7764895752165,95.361970645724),
 .UNSPECIFIED.);
#2407=B_SPLINE_CURVE_WITH_KNOTS('',3,(#50342,#50343,#50344,#50345,#50346,
#50347,#50348,#50349,#50350,#50351,#50352,#50353,#50354,#50355,#50356,#50357,
#50358,#50359,#50360,#50361,#50362,#50363),.UNSPECIFIED.,.F.,.F.,(4,3,3,
3,3,3,3,4),(-104.623506663712,-103.755314903395,-102.757667644708,-101.760020386022,
-100.762373127335,-99.7647258686489,-98.7670786099624,-98.3403213565322),
 .UNSPECIFIED.);
#2408=B_SPLINE_CURVE_WITH_KNOTS('',3,(#50364,#50365,#50366,#50367,#50368,
#50369,#50370,#50371,#50372,#50373,#50374,#50375,#50376,#50377,#50378,#50379,
#50380,#50381,#50382,#50383,#50384,#50385),.UNSPECIFIED.,.F.,.F.,(4,3,3,
3,3,3,3,4),(95.361970645724,95.774136833903,96.7717840925895,97.769431351276,
98.7670786099625,99.7647258686489,100.762373127335,101.645155952904),
 .UNSPECIFIED.);
#2409=B_SPLINE_CURVE_WITH_KNOTS('',3,(#50390,#50391,#50392,#50393,#50394,
#50395,#50396,#50397,#50398,#50399,#50400,#50401,#50402,#50403,#50404,#50405,
#50406,#50407,#50408,#50409,#50410,#50411,#50412,#50413,#50414),
 .UNSPECIFIED.,.F.,.F.,(4,3,3,3,3,3,3,3,4),(-110.906691970891,-110.7388457142,
-109.741198455514,-108.743551196827,-107.745903938141,-106.748256679454,
-105.750609420768,-104.752962162081,-104.623506663712),.UNSPECIFIED.);
#2410=B_SPLINE_CURVE_WITH_KNOTS('',3,(#50415,#50416,#50417,#50418,#50419,
#50420,#50421,#50422,#50423,#50424,#50425,#50426,#50427,#50428,#50429,#50430,
#50431,#50432,#50433,#50434,#50435,#50436,#50437,#50438,#50439),
 .UNSPECIFIED.,.F.,.F.,(4,3,3,3,3,3,3,3,4),(101.645155952904,101.760020386022,
102.757667644708,103.755314903395,104.752962162081,105.750609420768,106.748256679454,
107.745903938141,107.928341260083),.UNSPECIFIED.);
#2411=B_SPLINE_CURVE_WITH_KNOTS('',3,(#50444,#50445,#50446,#50447,#50448,
#50449,#50450,#50451,#50452,#50453,#50454,#50455,#50456,#50457,#50458,#50459,
#50460,#50461,#50462,#50463,#50464,#50465),.UNSPECIFIED.,.F.,.F.,(4,3,3,
3,3,3,3,4),(-117.189877278071,-116.724729266319,-115.727082007633,-114.729434748946,
-113.73178749026,-112.734140231573,-111.736492972887,-110.906691970891),
 .UNSPECIFIED.);
#2412=B_SPLINE_CURVE_WITH_KNOTS('',3,(#50466,#50467,#50468,#50469,#50470,
#50471,#50472,#50473,#50474,#50475,#50476,#50477,#50478,#50479,#50480,#50481,
#50482,#50483,#50484,#50485,#50486,#50487),.UNSPECIFIED.,.F.,.F.,(4,3,3,
3,3,3,3,4),(107.928341260083,108.743551196827,109.741198455514,110.7388457142,
111.736492972887,112.734140231573,113.73178749026,114.211526567263),
 .UNSPECIFIED.);
#2413=B_SPLINE_CURVE_WITH_KNOTS('',3,(#50492,#50493,#50494,#50495,#50496,
#50497,#50498,#50499,#50500,#50501,#50502,#50503,#50504,#50505,#50506,#50507,
#50508,#50509,#50510,#50511,#50512,#50513),.UNSPECIFIED.,.F.,.F.,(4,3,3,
3,3,3,3,4),(-123.473062585251,-122.710612818438,-121.712965559752,-120.715318301065,
-119.717671042379,-118.720023783692,-117.722376525006,-117.189877278071),
 .UNSPECIFIED.);
#2414=B_SPLINE_CURVE_WITH_KNOTS('',3,(#50514,#50515,#50516,#50517,#50518,
#50519,#50520,#50521,#50522,#50523,#50524,#50525,#50526,#50527,#50528,#50529,
#50530,#50531,#50532,#50533,#50534,#50535),.UNSPECIFIED.,.F.,.F.,(4,3,3,
3,3,3,3,4),(114.211526567263,114.729434748946,115.727082007633,116.724729266319,
117.722376525006,118.720023783692,119.717671042379,120.494711874442),
 .UNSPECIFIED.);
#2415=B_SPLINE_CURVE_WITH_KNOTS('',3,(#50540,#50541,#50542,#50543,#50544,
#50545,#50546,#50547,#50548,#50549,#50550,#50551,#50552,#50553,#50554,#50555,
#50556,#50557,#50558,#50559,#50560,#50561,#50562,#50563,#50564),
 .UNSPECIFIED.,.F.,.F.,(4,3,3,3,3,3,3,3,4),(-129.75624789243,-129.694143629244,
-128.696496370557,-127.698849111871,-126.701201853184,-125.703554594498,
-124.705907335811,-123.708260077125,-123.473062585251),.UNSPECIFIED.);
#2416=B_SPLINE_CURVE_WITH_KNOTS('',3,(#50565,#50566,#50567,#50568,#50569,
#50570,#50571,#50572,#50573,#50574,#50575,#50576,#50577,#50578,#50579,#50580,
#50581,#50582,#50583,#50584,#50585,#50586,#50587,#50588,#50589),
 .UNSPECIFIED.,.F.,.F.,(4,3,3,3,3,3,3,3,4),(120.494711874442,120.715318301065,
121.712965559752,122.710612818438,123.708260077125,124.705907335811,125.703554594498,
126.701201853184,126.777897181622),.UNSPECIFIED.);
#2417=B_SPLINE_CURVE_WITH_KNOTS('',3,(#50594,#50595,#50596,#50597,#50598,
#50599,#50600,#50601,#50602,#50603,#50604,#50605,#50606,#50607,#50608,#50609,
#50610,#50611,#50612,#50613,#50614,#50615),.UNSPECIFIED.,.F.,.F.,(4,3,3,
3,3,3,3,4),(-136.03943319961,-135.680027181363,-134.682379922676,-133.68473266399,
-132.687085405303,-131.689438146617,-130.69179088793,-129.75624789243),
 .UNSPECIFIED.);
#2418=B_SPLINE_CURVE_WITH_KNOTS('',3,(#50616,#50617,#50618,#50619,#50620,
#50621,#50622,#50623,#50624,#50625,#50626,#50627,#50628,#50629,#50630,#50631,
#50632,#50633,#50634,#50635,#50636,#50637),.UNSPECIFIED.,.F.,.F.,(4,3,3,
3,3,3,3,4),(126.777897181622,127.698849111871,128.696496370557,129.694143629244,
130.69179088793,131.689438146617,132.687085405303,133.061082488802),
 .UNSPECIFIED.);
#2419=B_SPLINE_CURVE_WITH_KNOTS('',3,(#50642,#50643,#50644,#50645,#50646,
#50647,#50648,#50649,#50650,#50651,#50652,#50653,#50654,#50655,#50656,#50657,
#50658,#50659,#50660,#50661,#50662,#50663),.UNSPECIFIED.,.F.,.F.,(4,3,3,
3,3,3,3,4),(-142.322618506789,-141.665910733481,-140.668263474795,-139.670616216108,
-138.672968957422,-137.675321698735,-136.677674440049,-136.03943319961),
 .UNSPECIFIED.);
#2420=B_SPLINE_CURVE_WITH_KNOTS('',3,(#50664,#50665,#50666,#50667,#50668,
#50669,#50670,#50671,#50672,#50673,#50674,#50675,#50676,#50677,#50678,#50679,
#50680,#50681,#50682,#50683,#50684,#50685),.UNSPECIFIED.,.F.,.F.,(4,3,3,
3,3,3,3,4),(133.061082488802,133.68473266399,134.682379922676,135.680027181363,
136.677674440049,137.675321698736,138.672968957422,139.344267795981),
 .UNSPECIFIED.);
#2421=B_SPLINE_CURVE_WITH_KNOTS('',3,(#50690,#50691,#50692,#50693,#50694,
#50695,#50696,#50697,#50698,#50699,#50700,#50701,#50702,#50703,#50704,#50705,
#50706,#50707,#50708,#50709,#50710,#50711),.UNSPECIFIED.,.F.,.F.,(4,3,3,
3,3,3,3,4),(-148.605803813969,-147.6517942856,-146.654147026914,-145.656499768227,
-144.658852509541,-143.661205250854,-142.663557992168,-142.322618506789),
 .UNSPECIFIED.);
#2422=B_SPLINE_CURVE_WITH_KNOTS('',3,(#50712,#50713,#50714,#50715,#50716,
#50717,#50718,#50719,#50720,#50721,#50722,#50723,#50724,#50725,#50726,#50727,
#50728,#50729,#50730,#50731,#50732,#50733),.UNSPECIFIED.,.F.,.F.,(4,3,3,
3,3,3,3,4),(139.344267795981,139.670616216109,140.668263474795,141.665910733481,
142.663557992168,143.661205250854,144.658852509541,145.627453103161),
 .UNSPECIFIED.);
#2423=B_SPLINE_CURVE_WITH_KNOTS('',3,(#50738,#50739,#50740,#50741,#50742,
#50743,#50744,#50745,#50746,#50747,#50748,#50749,#50750,#50751,#50752,#50753,
#50754,#50755,#50756,#50757,#50758,#50759,#50760,#50761,#50762),
 .UNSPECIFIED.,.F.,.F.,(4,3,3,3,3,3,3,3,4),(-154.888989121148,-154.635325096406,
-153.637677837719,-152.640030579033,-151.642383320346,-150.64473606166,
-149.647088802973,-148.649441544287,-148.605803813969),.UNSPECIFIED.);
#2424=B_SPLINE_CURVE_WITH_KNOTS('',3,(#50763,#50764,#50765,#50766,#50767,
#50768,#50769,#50770,#50771,#50772,#50773,#50774,#50775,#50776,#50777,#50778,
#50779,#50780,#50781,#50782,#50783,#50784,#50785,#50786,#50787),
 .UNSPECIFIED.,.F.,.F.,(4,3,3,3,3,3,3,3,4),(145.627453103161,145.656499768227,
146.654147026914,147.6517942856,148.649441544287,149.647088802973,150.64473606166,
151.642383320346,151.91063841034),.UNSPECIFIED.);
#2425=B_SPLINE_CURVE_WITH_KNOTS('',3,(#50792,#50793,#50794,#50795,#50796,
#50797,#50798,#50799,#50800,#50801,#50802,#50803,#50804,#50805,#50806,#50807,
#50808,#50809,#50810,#50811,#50812,#50813),.UNSPECIFIED.,.F.,.F.,(4,3,3,
3,3,3,3,4),(-161.172174428328,-160.621208648525,-159.623561389838,-158.625914131152,
-157.628266872465,-156.630619613779,-155.632972355092,-154.888989121148),
 .UNSPECIFIED.);
#2426=B_SPLINE_CURVE_WITH_KNOTS('',3,(#50814,#50815,#50816,#50817,#50818,
#50819,#50820,#50821,#50822,#50823,#50824,#50825,#50826,#50827,#50828,#50829,
#50830,#50831,#50832,#50833,#50834,#50835),.UNSPECIFIED.,.F.,.F.,(4,3,3,
3,3,3,3,4),(151.91063841034,152.640030579033,153.637677837719,154.635325096406,
155.632972355092,156.630619613779,157.628266872465,158.19382371752),
 .UNSPECIFIED.);
#2427=B_SPLINE_CURVE_WITH_KNOTS('',3,(#50840,#50841,#50842,#50843,#50844,
#50845,#50846,#50847,#50848,#50849,#50850,#50851,#50852,#50853,#50854,#50855,
#50856,#50857,#50858,#50859,#50860,#50861),.UNSPECIFIED.,.F.,.F.,(4,3,3,
3,3,3,3,4),(-167.455359735508,-166.607092200644,-165.609444941957,-164.611797683271,
-163.614150424584,-162.616503165898,-161.618855907211,-161.172174428328),
 .UNSPECIFIED.);
#2428=B_SPLINE_CURVE_WITH_KNOTS('',3,(#50862,#50863,#50864,#50865,#50866,
#50867,#50868,#50869,#50870,#50871,#50872,#50873,#50874,#50875,#50876,#50877,
#50878,#50879,#50880,#50881,#50882,#50883),.UNSPECIFIED.,.F.,.F.,(4,3,3,
3,3,3,3,4),(158.19382371752,158.625914131152,159.623561389838,160.621208648525,
161.618855907211,162.616503165898,163.614150424584,164.477009024699),
 .UNSPECIFIED.);
#2429=B_SPLINE_CURVE_WITH_KNOTS('',3,(#50888,#50889,#50890,#50891,#50892,
#50893,#50894,#50895,#50896,#50897,#50898,#50899,#50900,#50901,#50902,#50903,
#50904,#50905,#50906,#50907,#50908,#50909,#50910,#50911,#50912),
 .UNSPECIFIED.,.F.,.F.,(4,3,3,3,3,3,3,3,4),(-173.738545042687,-173.590623011449,
-172.592975752763,-171.595328494076,-170.59768123539,-169.600033976703,
-168.602386718017,-167.60473945933,-167.455359735508),.UNSPECIFIED.);
#2430=B_SPLINE_CURVE_WITH_KNOTS('',3,(#50913,#50914,#50915,#50916,#50917,
#50918,#50919,#50920,#50921,#50922,#50923,#50924,#50925,#50926,#50927,#50928,
#50929,#50930,#50931,#50932,#50933,#50934,#50935,#50936,#50937),
 .UNSPECIFIED.,.F.,.F.,(4,3,3,3,3,3,3,3,4),(164.477009024699,164.611797683271,
165.609444941957,166.607092200644,167.60473945933,168.602386718017,169.600033976703,
170.59768123539,170.760194331879),.UNSPECIFIED.);
#2431=B_SPLINE_CURVE_WITH_KNOTS('',3,(#50942,#50943,#50944,#50945,#50946,
#50947,#50948,#50949,#50950,#50951,#50952,#50953,#50954,#50955,#50956,#50957,
#50958,#50959,#50960,#50961,#50962,#50963),.UNSPECIFIED.,.F.,.F.,(4,3,3,
3,3,3,3,4),(-180.021730349867,-179.576506563568,-178.578859304882,-177.581212046195,
-176.583564787509,-175.585917528822,-174.588270270136,-173.738545042687),
 .UNSPECIFIED.);
#2432=B_SPLINE_CURVE_WITH_KNOTS('',3,(#50964,#50965,#50966,#50967,#50968,
#50969,#50970,#50971,#50972,#50973,#50974,#50975,#50976,#50977,#50978,#50979,
#50980,#50981,#50982,#50983,#50984,#50985),.UNSPECIFIED.,.F.,.F.,(4,3,3,
3,3,3,3,4),(170.760194331879,171.595328494076,172.592975752763,173.590623011449,
174.588270270136,175.585917528822,176.583564787509,177.043379639058),
 .UNSPECIFIED.);
#2433=B_SPLINE_CURVE_WITH_KNOTS('',3,(#50990,#50991,#50992,#50993,#50994,
#50995,#50996,#50997,#50998,#50999,#51000,#51001,#51002,#51003,#51004,#51005,
#51006,#51007,#51008,#51009,#51010,#51011),.UNSPECIFIED.,.F.,.F.,(4,3,3,
3,3,3,3,4),(-186.304915657046,-185.562390115687,-184.564742857,-183.567095598314,
-182.569448339627,-181.571801080941,-180.574153822254,-180.021730349867),
 .UNSPECIFIED.);
#2434=B_SPLINE_CURVE_WITH_KNOTS('',3,(#51012,#51013,#51014,#51015,#51016,
#51017,#51018,#51019,#51020,#51021,#51022,#51023,#51024,#51025,#51026,#51027,
#51028,#51029,#51030,#51031,#51032,#51033),.UNSPECIFIED.,.F.,.F.,(4,3,3,
3,3,3,3,4),(177.043379639058,177.581212046195,178.578859304882,179.576506563568,
180.574153822255,181.571801080941,182.569448339628,183.326564946238),
 .UNSPECIFIED.);
#2435=B_SPLINE_CURVE_WITH_KNOTS('',3,(#51038,#51039,#51040,#51041,#51042,
#51043,#51044,#51045,#51046,#51047,#51048,#51049,#51050,#51051,#51052,#51053,
#51054,#51055,#51056,#51057,#51058,#51059,#51060,#51061,#51062),
 .UNSPECIFIED.,.F.,.F.,(4,3,3,3,3,3,3,3,4),(-192.588100964226,-192.545920926492,
-191.548273667806,-190.550626409119,-189.552979150433,-188.555331891746,
-187.55768463306,-186.560037374373,-186.304915657046),.UNSPECIFIED.);
#2436=B_SPLINE_CURVE_WITH_KNOTS('',3,(#51063,#51064,#51065,#51066,#51067,
#51068,#51069,#51070,#51071,#51072,#51073,#51074,#51075,#51076,#51077,#51078,
#51079,#51080,#51081,#51082,#51083,#51084,#51085,#51086,#51087),
 .UNSPECIFIED.,.F.,.F.,(4,3,3,3,3,3,3,3,4),(183.326564946238,183.567095598314,
184.564742857001,185.562390115687,186.560037374374,187.55768463306,188.555331891746,
189.552979150433,189.609750253418),.UNSPECIFIED.);
#2437=B_SPLINE_CURVE_WITH_KNOTS('',3,(#51092,#51093,#51094,#51095,#51096,
#51097,#51098,#51099,#51100,#51101,#51102,#51103,#51104,#51105,#51106,#51107,
#51108,#51109,#51110,#51111,#51112,#51113),.UNSPECIFIED.,.F.,.F.,(4,3,3,
3,3,3,3,4),(-198.871286271405,-198.531804478611,-197.534157219925,-196.536509961238,
-195.538862702552,-194.541215443865,-193.543568185179,-192.588100964226),
 .UNSPECIFIED.);
#2438=B_SPLINE_CURVE_WITH_KNOTS('',3,(#51114,#51115,#51116,#51117,#51118,
#51119,#51120,#51121,#51122,#51123,#51124,#51125,#51126,#51127,#51128,#51129,
#51130,#51131,#51132,#51133,#51134,#51135),.UNSPECIFIED.,.F.,.F.,(4,3,3,
3,3,3,3,4),(189.609750253418,190.55062640912,191.548273667806,192.545920926492,
193.543568185179,194.541215443865,195.538862702552,195.892935560597),
 .UNSPECIFIED.);
#2439=B_SPLINE_CURVE_WITH_KNOTS('',3,(#51140,#51141,#51142,#51143,#51144,
#51145,#51146,#51147,#51148,#51149,#51150,#51151,#51152,#51153,#51154,#51155,
#51156,#51157,#51158,#51159,#51160,#51161),.UNSPECIFIED.,.F.,.F.,(4,3,3,
3,3,3,3,4),(-205.154471578585,-204.51768803073,-203.520040772044,-202.522393513357,
-201.524746254671,-200.527098995984,-199.529451737298,-198.871286271405),
 .UNSPECIFIED.);
#2440=B_SPLINE_CURVE_WITH_KNOTS('',3,(#51162,#51163,#51164,#51165,#51166,
#51167,#51168,#51169,#51170,#51171,#51172,#51173,#51174,#51175,#51176,#51177,
#51178,#51179,#51180,#51181,#51182,#51183),.UNSPECIFIED.,.F.,.F.,(4,3,3,
3,3,3,3,4),(195.892935560597,196.536509961238,197.534157219925,198.531804478611,
199.529451737298,200.527098995984,201.524746254671,202.176120867777),
 .UNSPECIFIED.);
#2441=B_SPLINE_CURVE_WITH_KNOTS('',3,(#51188,#51189,#51190,#51191,#51192,
#51193,#51194,#51195,#51196,#51197,#51198,#51199,#51200,#51201,#51202,#51203,
#51204,#51205,#51206,#51207,#51208,#51209),.UNSPECIFIED.,.F.,.F.,(4,3,3,
3,3,3,3,4),(-211.437656885764,-210.503571582849,-209.505924324163,-208.508277065476,
-207.51062980679,-206.512982548103,-205.515335289417,-205.154471578585),
 .UNSPECIFIED.);
#2442=B_SPLINE_CURVE_WITH_KNOTS('',3,(#51210,#51211,#51212,#51213,#51214,
#51215,#51216,#51217,#51218,#51219,#51220,#51221,#51222,#51223,#51224,#51225,
#51226,#51227,#51228,#51229,#51230,#51231),.UNSPECIFIED.,.F.,.F.,(4,3,3,
3,3,3,3,4),(202.176120867777,202.522393513357,203.520040772044,204.51768803073,
205.515335289417,206.512982548103,207.51062980679,208.459306174956),
 .UNSPECIFIED.);
#2443=B_SPLINE_CURVE_WITH_KNOTS('',3,(#51236,#51237,#51238,#51239,#51240,
#51241,#51242,#51243,#51244,#51245,#51246,#51247,#51248,#51249,#51250,#51251,
#51252,#51253,#51254,#51255,#51256,#51257,#51258,#51259,#51260),
 .UNSPECIFIED.,.F.,.F.,(4,3,3,3,3,3,3,3,4),(-217.720842192944,-217.487102393655,
-216.489455134968,-215.491807876282,-214.494160617595,-213.496513358909,
-212.498866100222,-211.501218841536,-211.437656885764),.UNSPECIFIED.);
#2444=B_SPLINE_CURVE_WITH_KNOTS('',3,(#51261,#51262,#51263,#51264,#51265,
#51266,#51267,#51268,#51269,#51270,#51271,#51272,#51273,#51274,#51275,#51276,
#51277,#51278,#51279,#51280,#51281,#51282,#51283,#51284,#51285),
 .UNSPECIFIED.,.F.,.F.,(4,3,3,3,3,3,3,3,4),(208.459306174956,208.508277065476,
209.505924324163,210.503571582849,211.501218841536,212.498866100222,213.496513358909,
214.494160617595,214.742491482136),.UNSPECIFIED.);
#2445=B_SPLINE_CURVE_WITH_KNOTS('',3,(#51290,#51291,#51292,#51293,#51294,
#51295,#51296,#51297,#51298,#51299,#51300,#51301,#51302,#51303,#51304,#51305,
#51306,#51307,#51308,#51309,#51310,#51311),.UNSPECIFIED.,.F.,.F.,(4,3,3,
3,3,3,3,4),(-224.004027500124,-223.472985945774,-222.475338687087,-221.477691428401,
-220.480044169714,-219.482396911028,-218.484749652341,-217.720842192944),
 .UNSPECIFIED.);
#2446=B_SPLINE_CURVE_WITH_KNOTS('',3,(#51312,#51313,#51314,#51315,#51316,
#51317,#51318,#51319,#51320,#51321,#51322,#51323,#51324,#51325,#51326,#51327,
#51328,#51329,#51330,#51331,#51332,#51333),.UNSPECIFIED.,.F.,.F.,(4,3,3,
3,3,3,3,4),(214.742491482136,215.491807876282,216.489455134968,217.487102393655,
218.484749652341,219.482396911028,220.480044169714,221.025676789315),
 .UNSPECIFIED.);
#2447=B_SPLINE_CURVE_WITH_KNOTS('',3,(#51338,#51339,#51340,#51341,#51342,
#51343,#51344,#51345,#51346,#51347,#51348,#51349,#51350,#51351,#51352,#51353,
#51354,#51355,#51356,#51357,#51358,#51359),.UNSPECIFIED.,.F.,.F.,(4,3,3,
3,3,3,3,4),(-230.287212807303,-229.458869497892,-228.461222239206,-227.463574980519,
-226.465927721833,-225.468280463147,-224.47063320446,-224.004027500124),
 .UNSPECIFIED.);
#2448=B_SPLINE_CURVE_WITH_KNOTS('',3,(#51360,#51361,#51362,#51363,#51364,
#51365,#51366,#51367,#51368,#51369,#51370,#51371,#51372,#51373,#51374,#51375,
#51376,#51377,#51378,#51379,#51380,#51381),.UNSPECIFIED.,.F.,.F.,(4,3,3,
3,3,3,3,4),(221.025676789315,221.477691428401,222.475338687087,223.472985945774,
224.47063320446,225.468280463147,226.465927721833,227.308862096495),
 .UNSPECIFIED.);
#2449=B_SPLINE_CURVE_WITH_KNOTS('',3,(#51386,#51387,#51388,#51389,#51390,
#51391,#51392,#51393,#51394,#51395,#51396,#51397,#51398,#51399,#51400,#51401,
#51402,#51403,#51404,#51405,#51406,#51407,#51408,#51409,#51410),
 .UNSPECIFIED.,.F.,.F.,(4,3,3,3,3,3,3,3,4),(-236.570398114483,-236.442400308698,
-235.444753050011,-234.447105791325,-233.449458532638,-232.451811273952,
-231.454164015265,-230.456516756579,-230.287212807303),.UNSPECIFIED.);
#2450=B_SPLINE_CURVE_WITH_KNOTS('',3,(#51411,#51412,#51413,#51414,#51415,
#51416,#51417,#51418,#51419,#51420,#51421,#51422,#51423,#51424,#51425,#51426,
#51427,#51428,#51429,#51430,#51431,#51432,#51433,#51434,#51435),
 .UNSPECIFIED.,.F.,.F.,(4,3,3,3,3,3,3,3,4),(227.308862096495,227.46357498052,
228.461222239206,229.458869497893,230.456516756579,231.454164015266,232.451811273952,
233.449458532639,233.592047403675),.UNSPECIFIED.);
#2451=B_SPLINE_CURVE_WITH_KNOTS('',3,(#51440,#51441,#51442,#51443,#51444,
#51445,#51446,#51447,#51448,#51449,#51450,#51451,#51452,#51453,#51454,#51455,
#51456,#51457,#51458,#51459,#51460,#51461),.UNSPECIFIED.,.F.,.F.,(4,3,3,
3,3,3,3,4),(-242.853583421662,-242.428283860817,-241.43063660213,-240.432989343444,
-239.435342084757,-238.437694826071,-237.440047567384,-236.570398114483),
 .UNSPECIFIED.);
#2452=B_SPLINE_CURVE_WITH_KNOTS('',3,(#51462,#51463,#51464,#51465,#51466,
#51467,#51468,#51469,#51470,#51471,#51472,#51473,#51474,#51475,#51476,#51477,
#51478,#51479,#51480,#51481,#51482,#51483),.UNSPECIFIED.,.F.,.F.,(4,3,3,
3,3,3,3,4),(233.592047403675,234.447105791325,235.444753050011,236.442400308698,
237.440047567384,238.437694826071,239.435342084757,239.875232710854),
 .UNSPECIFIED.);
#2453=B_SPLINE_CURVE_WITH_KNOTS('',3,(#51488,#51489,#51490,#51491,#51492,
#51493,#51494,#51495,#51496,#51497,#51498,#51499,#51500,#51501,#51502,#51503,
#51504,#51505,#51506,#51507,#51508,#51509),.UNSPECIFIED.,.F.,.F.,(4,3,3,
3,3,3,3,4),(-249.136768728842,-248.414167412936,-247.416520154249,-246.418872895563,
-245.421225636876,-244.42357837819,-243.425931119503,-242.853583421662),
 .UNSPECIFIED.);
#2454=B_SPLINE_CURVE_WITH_KNOTS('',3,(#51510,#51511,#51512,#51513,#51514,
#51515,#51516,#51517,#51518,#51519,#51520,#51521,#51522,#51523,#51524,#51525,
#51526,#51527,#51528,#51529,#51530,#51531),.UNSPECIFIED.,.F.,.F.,(4,3,3,
3,3,3,3,4),(239.875232710854,240.432989343444,241.43063660213,242.428283860817,
243.425931119503,244.42357837819,245.421225636876,246.158418018034),
 .UNSPECIFIED.);
#2455=B_SPLINE_CURVE_WITH_KNOTS('',3,(#51536,#51537,#51538,#51539,#51540,
#51541,#51542,#51543,#51544,#51545,#51546,#51547,#51548,#51549,#51550,#51551,
#51552,#51553,#51554,#51555,#51556,#51557,#51558,#51559,#51560),
 .UNSPECIFIED.,.F.,.F.,(4,3,3,3,3,3,3,3,4),(-255.419954036021,-255.397698223741,
-254.400050965055,-253.402403706368,-252.404756447682,-251.407109188995,
-250.409461930309,-249.411814671622,-249.136768728842),.UNSPECIFIED.);
#2456=B_SPLINE_CURVE_WITH_KNOTS('',3,(#51561,#51562,#51563,#51564,#51565,
#51566,#51567,#51568,#51569,#51570,#51571,#51572,#51573,#51574,#51575,#51576,
#51577,#51578,#51579,#51580,#51581,#51582,#51583,#51584,#51585),
 .UNSPECIFIED.,.F.,.F.,(4,3,3,3,3,3,3,3,4),(246.158418018034,246.418872895563,
247.416520154249,248.414167412936,249.411814671622,250.409461930309,251.407109188995,
252.404756447682,252.441603325213),.UNSPECIFIED.);
#2457=B_SPLINE_CURVE_WITH_KNOTS('',3,(#51590,#51591,#51592,#51593,#51594,
#51595,#51596,#51597,#51598,#51599,#51600,#51601,#51602,#51603,#51604,#51605,
#51606,#51607,#51608,#51609,#51610,#51611),.UNSPECIFIED.,.F.,.F.,(4,3,3,
3,3,3,3,4),(-261.703139343201,-261.38358177586,-260.385934517174,-259.388287258487,
-258.390639999801,-257.392992741114,-256.395345482428,-255.419954036021),
 .UNSPECIFIED.);
#2458=B_SPLINE_CURVE_WITH_KNOTS('',3,(#51612,#51613,#51614,#51615,#51616,
#51617,#51618,#51619,#51620,#51621,#51622,#51623,#51624,#51625,#51626,#51627,
#51628,#51629,#51630,#51631,#51632,#51633),.UNSPECIFIED.,.F.,.F.,(4,3,3,
3,3,3,3,4),(252.441603325213,253.402403706368,254.400050965055,255.397698223741,
256.395345482428,257.392992741114,258.390639999801,258.724788632393),
 .UNSPECIFIED.);
#2459=B_SPLINE_CURVE_WITH_KNOTS('',3,(#51639,#51640,#51641,#51642,#51643,
#51644),.UNSPECIFIED.,.F.,.F.,(4,1,1,4),(273.318560862312,273.996650553658,
274.994297812344,275.922099455125),.UNSPECIFIED.);
#2460=B_SPLINE_CURVE_WITH_KNOTS('',3,(#51647,#51648,#51649,#51650,#51651),
 .UNSPECIFIED.,.F.,.F.,(4,1,4),(273.318560862312,273.684757733346,274.682404992033),
 .UNSPECIFIED.);
#2461=B_SPLINE_CURVE_WITH_KNOTS('',3,(#51656,#51657,#51658,#51659,#51660,
#51661,#51662,#51663,#51664,#51665),.UNSPECIFIED.,.F.,.F.,(4,1,1,1,1,1,
1,4),(267.035375555132,268.010767001539,269.008414260225,270.006061518912,
271.003708777598,272.001356036285,272.999003294971,273.318560862312),
 .UNSPECIFIED.);
#2462=B_SPLINE_CURVE_WITH_KNOTS('',3,(#51666,#51667,#51668,#51669,#51670,
#51671,#51672,#51673,#51674,#51675),.UNSPECIFIED.,.F.,.F.,(4,1,1,1,1,1,
1,4),(267.035375555132,267.698874181227,268.696521439914,269.6941686986,
270.691815957287,271.689463215973,272.68711047466,273.318560862312),
 .UNSPECIFIED.);
#2463=B_SPLINE_CURVE_WITH_KNOTS('',3,(#51680,#51681,#51682,#51683,#51684,
#51685,#51686,#51687,#51688,#51689,#51690),.UNSPECIFIED.,.F.,.F.,(4,1,1,
1,1,1,1,1,4),(260.752190247953,261.027236190733,262.02488344942,263.022530708106,
264.020177966793,265.017825225479,266.015472484166,267.013119742852,267.035375555132),
 .UNSPECIFIED.);
#2464=B_SPLINE_CURVE_WITH_KNOTS('',3,(#51691,#51692,#51693,#51694,#51695,
#51696,#51697,#51698,#51699,#51700),.UNSPECIFIED.,.F.,.F.,(4,1,1,1,1,1,
1,4),(260.752190247953,261.712990629108,262.710637887795,263.708285146481,
264.705932405168,265.703579663854,266.701226922541,267.035375555132),
 .UNSPECIFIED.);
#2465=B_SPLINE_CURVE_WITH_KNOTS('',3,(#51705,#51706,#51707,#51708,#51709,
#51710,#51711,#51712,#51713,#51714),.UNSPECIFIED.,.F.,.F.,(4,1,1,1,1,1,
1,4),(254.469004940773,255.041352638614,256.038999897301,257.036647155987,
258.034294414674,259.03194167336,260.029588932047,260.752190247953),
 .UNSPECIFIED.);
#2466=B_SPLINE_CURVE_WITH_KNOTS('',3,(#51715,#51716,#51717,#51718,#51719,
#51720,#51721,#51722,#51723,#51724,#51725),.UNSPECIFIED.,.F.,.F.,(4,1,1,
1,1,1,1,1,4),(254.469004940773,254.729459818303,255.727107076989,256.724754335676,
257.722401594362,258.720048853049,259.717696111735,260.715343370422,260.752190247953),
 .UNSPECIFIED.);
#2467=B_SPLINE_CURVE_WITH_KNOTS('',3,(#51730,#51731,#51732,#51733,#51734,
#51735,#51736,#51737,#51738,#51739),.UNSPECIFIED.,.F.,.F.,(4,1,1,1,1,1,
1,4),(248.185819633594,249.055469086495,250.053116345182,251.050763603868,
252.048410862555,253.046058121241,254.043705379928,254.469004940773),
 .UNSPECIFIED.);
#2468=B_SPLINE_CURVE_WITH_KNOTS('',3,(#51740,#51741,#51742,#51743,#51744,
#51745,#51746,#51747,#51748,#51749),.UNSPECIFIED.,.F.,.F.,(4,1,1,1,1,1,
1,4),(248.185819633594,248.743576266184,249.74122352487,250.738870783557,
251.736518042243,252.73416530093,253.731812559616,254.469004940773),
 .UNSPECIFIED.);
#2469=B_SPLINE_CURVE_WITH_KNOTS('',3,(#51754,#51755,#51756,#51757,#51758,
#51759,#51760,#51761,#51762,#51763,#51764),.UNSPECIFIED.,.F.,.F.,(4,1,1,
1,1,1,1,1,4),(241.902634326414,242.07193827569,243.069585534376,244.067232793063,
245.064880051749,246.062527310436,247.060174569122,248.057821827809,248.185819633594),
 .UNSPECIFIED.);
#2470=B_SPLINE_CURVE_WITH_KNOTS('',3,(#51765,#51766,#51767,#51768,#51769,
#51770,#51771,#51772,#51773,#51774),.UNSPECIFIED.,.F.,.F.,(4,1,1,1,1,1,
1,4),(241.902634326414,242.757692714065,243.755339972752,244.752987231438,
245.750634490125,246.748281748811,247.745929007497,248.185819633594),
 .UNSPECIFIED.);
#2471=B_SPLINE_CURVE_WITH_KNOTS('',3,(#51779,#51780,#51781,#51782,#51783,
#51784,#51785,#51786,#51787,#51788),.UNSPECIFIED.,.F.,.F.,(4,1,1,1,1,1,
1,4),(235.619449019234,236.086054723571,237.083701982258,238.081349240944,
239.078996499631,240.076643758317,241.074291017004,241.902634326414),
 .UNSPECIFIED.);
#2472=B_SPLINE_CURVE_WITH_KNOTS('',3,(#51789,#51790,#51791,#51792,#51793,
#51794,#51795,#51796,#51797,#51798,#51799),.UNSPECIFIED.,.F.,.F.,(4,1,1,
1,1,1,1,1,4),(235.619449019235,235.77416190326,236.771809161946,237.769456420633,
238.767103679319,239.764750938006,240.762398196692,241.760045455379,241.902634326414),
 .UNSPECIFIED.);
#2473=B_SPLINE_CURVE_WITH_KNOTS('',3,(#51804,#51805,#51806,#51807,#51808,
#51809,#51810,#51811,#51812,#51813),.UNSPECIFIED.,.F.,.F.,(4,1,1,1,1,1,
1,4),(229.336263712055,230.100171171452,231.097818430139,232.095465688825,
233.093112947512,234.090760206198,235.088407464885,235.619449019234),
 .UNSPECIFIED.);
#2474=B_SPLINE_CURVE_WITH_KNOTS('',3,(#51814,#51815,#51816,#51817,#51818,
#51819,#51820,#51821,#51822,#51823),.UNSPECIFIED.,.F.,.F.,(4,1,1,1,1,1,
1,4),(229.336263712055,229.788278351141,230.785925609827,231.783572868514,
232.7812201272,233.778867385887,234.776514644573,235.619449019235),
 .UNSPECIFIED.);
#2475=B_SPLINE_CURVE_WITH_KNOTS('',3,(#51828,#51829,#51830,#51831,#51832,
#51833,#51834,#51835,#51836,#51837,#51838),.UNSPECIFIED.,.F.,.F.,(4,1,1,
1,1,1,1,1,4),(223.053078404875,223.116640360647,224.114287619333,225.11193487802,
226.109582136706,227.107229395393,228.104876654079,229.102523912766,229.336263712055),
 .UNSPECIFIED.);
#2476=B_SPLINE_CURVE_WITH_KNOTS('',3,(#51839,#51840,#51841,#51842,#51843,
#51844,#51845,#51846,#51847,#51848),.UNSPECIFIED.,.F.,.F.,(4,1,1,1,1,1,
1,4),(223.053078404875,223.802394799022,224.800042057708,225.797689316395,
226.795336575081,227.792983833768,228.790631092454,229.336263712055),
 .UNSPECIFIED.);
#2477=B_SPLINE_CURVE_WITH_KNOTS('',3,(#51853,#51854,#51855,#51856,#51857,
#51858,#51859,#51860,#51861,#51862),.UNSPECIFIED.,.F.,.F.,(4,1,1,1,1,1,
1,4),(216.769893097696,217.130756808528,218.128404067214,219.126051325901,
220.123698584587,221.121345843274,222.11899310196,223.053078404875),
 .UNSPECIFIED.);
#2478=B_SPLINE_CURVE_WITH_KNOTS('',3,(#51863,#51864,#51865,#51866,#51867,
#51868,#51869,#51870,#51871,#51872,#51873),.UNSPECIFIED.,.F.,.F.,(4,1,1,
1,1,1,1,1,4),(216.769893097696,216.818863988216,217.816511246903,218.814158505589,
219.811805764276,220.809453022962,221.807100281649,222.804747540335,223.053078404875),
 .UNSPECIFIED.);
#2479=B_SPLINE_CURVE_WITH_KNOTS('',3,(#51878,#51879,#51880,#51881,#51882,
#51883,#51884,#51885,#51886,#51887),.UNSPECIFIED.,.F.,.F.,(4,1,1,1,1,1,
1,4),(210.486707790516,211.144873256409,212.142520515095,213.140167773782,
214.137815032468,215.135462291155,216.133109549841,216.769893097696),
 .UNSPECIFIED.);
#2480=B_SPLINE_CURVE_WITH_KNOTS('',3,(#51888,#51889,#51890,#51891,#51892,
#51893,#51894,#51895,#51896,#51897),.UNSPECIFIED.,.F.,.F.,(4,1,1,1,1,1,
1,4),(210.486707790516,210.832980436097,211.830627694784,212.82827495347,
213.825922212157,214.823569470843,215.82121672953,216.769893097696),
 .UNSPECIFIED.);
#2481=B_SPLINE_CURVE_WITH_KNOTS('',3,(#51902,#51903,#51904,#51905,#51906,
#51907,#51908,#51909,#51910,#51911),.UNSPECIFIED.,.F.,.F.,(4,1,1,1,1,1,
1,4),(204.203522483337,205.15898970429,206.156636962976,207.154284221663,
208.151931480349,209.149578739036,210.147225997722,210.486707790516),
 .UNSPECIFIED.);
#2482=B_SPLINE_CURVE_WITH_KNOTS('',3,(#51912,#51913,#51914,#51915,#51916,
#51917,#51918,#51919,#51920,#51921),.UNSPECIFIED.,.F.,.F.,(4,1,1,1,1,1,
1,4),(204.203522483337,204.847096883978,205.844744142665,206.842391401351,
207.840038660038,208.837685918724,209.835333177411,210.486707790516),
 .UNSPECIFIED.);
#2483=B_SPLINE_CURVE_WITH_KNOTS('',3,(#51926,#51927,#51928,#51929,#51930,
#51931,#51932,#51933,#51934,#51935,#51936),.UNSPECIFIED.,.F.,.F.,(4,1,1,
1,1,1,1,1,4),(197.920337176157,198.175458893484,199.173106152171,200.170753410857,
201.168400669544,202.16604792823,203.163695186917,204.161342445603,204.203522483337),
 .UNSPECIFIED.);
#2484=B_SPLINE_CURVE_WITH_KNOTS('',3,(#51937,#51938,#51939,#51940,#51941,
#51942,#51943,#51944,#51945,#51946),.UNSPECIFIED.,.F.,.F.,(4,1,1,1,1,1,
1,4),(197.920337176157,198.86121333186,199.858860590546,200.856507849232,
201.854155107919,202.851802366605,203.849449625292,204.203522483337),
 .UNSPECIFIED.);
#2485=B_SPLINE_CURVE_WITH_KNOTS('',3,(#51951,#51952,#51953,#51954,#51955,
#51956,#51957,#51958,#51959,#51960),.UNSPECIFIED.,.F.,.F.,(4,1,1,1,1,1,
1,4),(191.637151868977,192.189575341366,193.187222600052,194.184869858739,
195.182517117425,196.180164376111,197.177811634798,197.920337176157),
 .UNSPECIFIED.);
#2486=B_SPLINE_CURVE_WITH_KNOTS('',3,(#51961,#51962,#51963,#51964,#51965,
#51966,#51967,#51968,#51969,#51970,#51971),.UNSPECIFIED.,.F.,.F.,(4,1,1,
1,1,1,1,1,4),(191.637151868978,191.877682521054,192.875329779741,193.872977038427,
194.870624297114,195.8682715558,196.865918814487,197.863566073173,197.920337176157),
 .UNSPECIFIED.);
#2487=B_SPLINE_CURVE_WITH_KNOTS('',3,(#51976,#51977,#51978,#51979,#51980,
#51981,#51982,#51983,#51984,#51985),.UNSPECIFIED.,.F.,.F.,(4,1,1,1,1,1,
1,4),(185.353966561798,186.203691789247,187.201339047933,188.19898630662,
189.196633565306,190.194280823993,191.191928082679,191.637151868977),
 .UNSPECIFIED.);
#2488=B_SPLINE_CURVE_WITH_KNOTS('',3,(#51986,#51987,#51988,#51989,#51990,
#51991,#51992,#51993,#51994,#51995),.UNSPECIFIED.,.F.,.F.,(4,1,1,1,1,1,
1,4),(185.353966561798,185.891798968935,186.889446227622,187.887093486308,
188.884740744995,189.882388003681,190.880035262368,191.637151868978),
 .UNSPECIFIED.);
#2489=B_SPLINE_CURVE_WITH_KNOTS('',3,(#52000,#52001,#52002,#52003,#52004,
#52005,#52006,#52007,#52008,#52009,#52010),.UNSPECIFIED.,.F.,.F.,(4,1,1,
1,1,1,1,1,4),(179.070781254618,179.220160978441,180.217808237128,181.215455495814,
182.213102754501,183.210750013187,184.208397271874,185.20604453056,185.353966561798),
 .UNSPECIFIED.);
#2490=B_SPLINE_CURVE_WITH_KNOTS('',3,(#52011,#52012,#52013,#52014,#52015,
#52016,#52017,#52018,#52019,#52020),.UNSPECIFIED.,.F.,.F.,(4,1,1,1,1,1,
1,4),(179.070781254619,179.905915416816,180.903562675503,181.901209934189,
182.898857192876,183.896504451562,184.894151710249,185.353966561798),
 .UNSPECIFIED.);
#2491=B_SPLINE_CURVE_WITH_KNOTS('',3,(#52025,#52026,#52027,#52028,#52029,
#52030,#52031,#52032,#52033,#52034),.UNSPECIFIED.,.F.,.F.,(4,1,1,1,1,1,
1,4),(172.787595947439,173.234277426322,174.231924685009,175.229571943695,
176.227219202382,177.224866461068,178.222513719755,179.070781254618),
 .UNSPECIFIED.);
#2492=B_SPLINE_CURVE_WITH_KNOTS('',3,(#52035,#52036,#52037,#52038,#52039,
#52040,#52041,#52042,#52043,#52044,#52045),.UNSPECIFIED.,.F.,.F.,(4,1,1,
1,1,1,1,1,4),(172.787595947439,172.922384606011,173.920031864697,174.917679123384,
175.91532638207,176.912973640757,177.910620899443,178.90826815813,179.070781254619),
 .UNSPECIFIED.);
#2493=B_SPLINE_CURVE_WITH_KNOTS('',3,(#52050,#52051,#52052,#52053,#52054,
#52055,#52056,#52057,#52058,#52059),.UNSPECIFIED.,.F.,.F.,(4,1,1,1,1,1,
1,4),(166.504410640259,167.248393874203,168.24604113289,169.243688391576,
170.241335650263,171.238982908949,172.236630167636,172.787595947439),
 .UNSPECIFIED.);
#2494=B_SPLINE_CURVE_WITH_KNOTS('',3,(#52060,#52061,#52062,#52063,#52064,
#52065,#52066,#52067,#52068,#52069),.UNSPECIFIED.,.F.,.F.,(4,1,1,1,1,1,
1,4),(166.504410640259,166.936501053892,167.934148312578,168.931795571265,
169.929442829951,170.927090088638,171.924737347324,172.787595947439),
 .UNSPECIFIED.);
#2495=B_SPLINE_CURVE_WITH_KNOTS('',3,(#52074,#52075,#52076,#52077,#52078,
#52079,#52080,#52081,#52082,#52083,#52084),.UNSPECIFIED.,.F.,.F.,(4,1,1,
1,1,1,1,1,4),(160.22122533308,160.264863063398,161.262510322084,162.260157580771,
163.257804839457,164.255452098144,165.25309935683,166.250746615517,166.504410640259),
 .UNSPECIFIED.);
#2496=B_SPLINE_CURVE_WITH_KNOTS('',3,(#52085,#52086,#52087,#52088,#52089,
#52090,#52091,#52092,#52093,#52094),.UNSPECIFIED.,.F.,.F.,(4,1,1,1,1,1,
1,4),(160.22122533308,160.950617501773,161.948264760459,162.945912019146,
163.943559277832,164.941206536519,165.938853795205,166.504410640259),
 .UNSPECIFIED.);
#2497=B_SPLINE_CURVE_WITH_KNOTS('',3,(#52099,#52100,#52101,#52102,#52103,
#52104,#52105,#52106,#52107,#52108),.UNSPECIFIED.,.F.,.F.,(4,1,1,1,1,1,
1,4),(153.9380400259,154.278979511279,155.276626769965,156.274274028652,
157.271921287338,158.269568546025,159.267215804711,160.22122533308),
 .UNSPECIFIED.);
#2498=B_SPLINE_CURVE_WITH_KNOTS('',3,(#52109,#52110,#52111,#52112,#52113,
#52114,#52115,#52116,#52117,#52118,#52119),.UNSPECIFIED.,.F.,.F.,(4,1,1,
1,1,1,1,1,4),(153.9380400259,153.967086690968,154.964733949654,155.96238120834,
156.960028467027,157.957675725713,158.9553229844,159.952970243086,160.22122533308),
 .UNSPECIFIED.);
#2499=B_SPLINE_CURVE_WITH_KNOTS('',3,(#52124,#52125,#52126,#52127,#52128,
#52129,#52130,#52131,#52132,#52133),.UNSPECIFIED.,.F.,.F.,(4,1,1,1,1,1,
1,4),(147.654854718721,148.29309595916,149.290743217847,150.288390476533,
151.286037735219,152.283684993906,153.281332252592,153.9380400259),
 .UNSPECIFIED.);
#2500=B_SPLINE_CURVE_WITH_KNOTS('',3,(#52134,#52135,#52136,#52137,#52138,
#52139,#52140,#52141,#52142,#52143),.UNSPECIFIED.,.F.,.F.,(4,1,1,1,1,1,
1,4),(147.654854718721,147.981203138849,148.978850397535,149.976497656222,
150.974144914908,151.971792173595,152.969439432281,153.9380400259),
 .UNSPECIFIED.);
#2501=B_SPLINE_CURVE_WITH_KNOTS('',3,(#52148,#52149,#52150,#52151,#52152,
#52153,#52154,#52155,#52156,#52157),.UNSPECIFIED.,.F.,.F.,(4,1,1,1,1,1,
1,4),(141.371669411541,142.307212407041,143.304859665728,144.302506924414,
145.300154183101,146.297801441787,147.295448700474,147.654854718721),
 .UNSPECIFIED.);
#2502=B_SPLINE_CURVE_WITH_KNOTS('',3,(#52158,#52159,#52160,#52161,#52162,
#52163,#52164,#52165,#52166,#52167),.UNSPECIFIED.,.F.,.F.,(4,1,1,1,1,1,
1,4),(141.371669411541,141.99531958673,142.992966845416,143.990614104103,
144.988261362789,145.985908621476,146.983555880162,147.654854718721),
 .UNSPECIFIED.);
#2503=B_SPLINE_CURVE_WITH_KNOTS('',3,(#52172,#52173,#52174,#52175,#52176,
#52177,#52178,#52179,#52180,#52181,#52182),.UNSPECIFIED.,.F.,.F.,(4,1,1,
1,1,1,1,1,4),(135.088484104361,135.323681596236,136.321328854922,137.318976113609,
138.316623372295,139.314270630982,140.311917889668,141.309565148355,141.371669411541),
 .UNSPECIFIED.);
#2504=B_SPLINE_CURVE_WITH_KNOTS('',3,(#52183,#52184,#52185,#52186,#52187,
#52188,#52189,#52190,#52191,#52192),.UNSPECIFIED.,.F.,.F.,(4,1,1,1,1,1,
1,4),(135.088484104362,136.009436034611,137.007083293297,138.004730551984,
139.00237781067,140.000025069357,140.997672328043,141.371669411541),
 .UNSPECIFIED.);
#2505=B_SPLINE_CURVE_WITH_KNOTS('',3,(#52197,#52198,#52199,#52200,#52201,
#52202,#52203,#52204,#52205,#52206),.UNSPECIFIED.,.F.,.F.,(4,1,1,1,1,1,
1,4),(128.805298797182,129.337798044117,130.335445302803,131.33309256149,
132.330739820176,133.328387078863,134.326034337549,135.088484104361),
 .UNSPECIFIED.);
#2506=B_SPLINE_CURVE_WITH_KNOTS('',3,(#52207,#52208,#52209,#52210,#52211,
#52212,#52213,#52214,#52215,#52216,#52217),.UNSPECIFIED.,.F.,.F.,(4,1,1,
1,1,1,1,1,4),(128.805298797182,129.025905223805,130.023552482492,131.021199741178,
132.018846999865,133.016494258551,134.014141517238,135.011788775924,135.088484104362),
 .UNSPECIFIED.);
#2507=B_SPLINE_CURVE_WITH_KNOTS('',3,(#52222,#52223,#52224,#52225,#52226,
#52227,#52228,#52229,#52230,#52231),.UNSPECIFIED.,.F.,.F.,(4,1,1,1,1,1,
1,4),(122.522113490002,123.351914491998,124.349561750684,125.347209009371,
126.344856268057,127.342503526744,128.34015078543,128.805298797182),
 .UNSPECIFIED.);
#2508=B_SPLINE_CURVE_WITH_KNOTS('',3,(#52232,#52233,#52234,#52235,#52236,
#52237,#52238,#52239,#52240,#52241),.UNSPECIFIED.,.F.,.F.,(4,1,1,1,1,1,
1,4),(122.522113490002,123.040021671686,124.037668930373,125.035316189059,
126.032963447746,127.030610706432,128.028257965119,128.805298797182),
 .UNSPECIFIED.);
#2509=B_SPLINE_CURVE_WITH_KNOTS('',3,(#52246,#52247,#52248,#52249,#52250,
#52251,#52252,#52253,#52254,#52255,#52256),.UNSPECIFIED.,.F.,.F.,(4,1,1,
1,1,1,1,1,4),(116.238928182823,116.368383681192,117.366030939879,118.363678198565,
119.361325457252,120.358972715938,121.356619974625,122.354267233311,122.522113490002),
 .UNSPECIFIED.);
#2510=B_SPLINE_CURVE_WITH_KNOTS('',3,(#52257,#52258,#52259,#52260,#52261,
#52262,#52263,#52264,#52265,#52266),.UNSPECIFIED.,.F.,.F.,(4,1,1,1,1,1,
1,4),(116.238928182823,117.054138119567,118.051785378254,119.04943263694,
120.047079895627,121.044727154313,122.042374413,122.522113490002),
 .UNSPECIFIED.);
#2511=B_SPLINE_CURVE_WITH_KNOTS('',3,(#52271,#52272,#52273,#52274,#52275,
#52276,#52277,#52278,#52279,#52280),.UNSPECIFIED.,.F.,.F.,(4,1,1,1,1,1,
1,4),(109.955742875643,110.382500129073,111.38014738776,112.377794646446,
113.375441905133,114.373089163819,115.370736422506,116.238928182823),
 .UNSPECIFIED.);
#2512=B_SPLINE_CURVE_WITH_KNOTS('',3,(#52281,#52282,#52283,#52284,#52285,
#52286,#52287,#52288,#52289,#52290,#52291),.UNSPECIFIED.,.F.,.F.,(4,1,1,
1,1,1,1,1,4),(109.955742875643,110.070607308762,111.068254567448,112.065901826135,
113.063549084821,114.061196343508,115.058843602194,116.056490860881,116.238928182823),
 .UNSPECIFIED.);
#2513=B_SPLINE_CURVE_WITH_KNOTS('',3,(#52296,#52297,#52298,#52299,#52300,
#52301,#52302,#52303,#52304,#52305),.UNSPECIFIED.,.F.,.F.,(4,1,1,1,1,1,
1,4),(103.672557568464,104.396616576955,105.394263835641,106.391911094327,
107.389558353014,108.3872056117,109.384852870387,109.955742875643),
 .UNSPECIFIED.);
#2514=B_SPLINE_CURVE_WITH_KNOTS('',3,(#52306,#52307,#52308,#52309,#52310,
#52311,#52312,#52313,#52314,#52315),.UNSPECIFIED.,.F.,.F.,(4,1,1,1,1,1,
1,4),(103.672557568464,104.084723756643,105.08237101533,106.080018274016,
107.077665532703,108.075312791389,109.072960050075,109.955742875643),
 .UNSPECIFIED.);
#2515=B_SPLINE_CURVE_WITH_KNOTS('',3,(#52320,#52321,#52322,#52323,#52324,
#52325,#52326,#52327,#52328,#52329,#52330),.UNSPECIFIED.,.F.,.F.,(4,1,1,
1,1,1,1,1,4),(97.3893722612839,97.4130857661491,98.4107330248356,99.4083802835221,
100.406027542209,101.403674800895,102.401322059582,103.398969318268,103.672557568464),
 .UNSPECIFIED.);
#2516=B_SPLINE_CURVE_WITH_KNOTS('',3,(#52331,#52332,#52333,#52334,#52335,
#52336,#52337,#52338,#52339,#52340),.UNSPECIFIED.,.F.,.F.,(4,1,1,1,1,1,
1,4),(97.389372261284,98.0988402045241,99.0964874632106,100.094134721897,
101.091781980584,102.08942923927,103.087076497957,103.672557568464),
 .UNSPECIFIED.);
#2517=B_SPLINE_CURVE_WITH_KNOTS('',3,(#52345,#52346,#52347,#52348,#52349,
#52350,#52351,#52352,#52353,#52354),.UNSPECIFIED.,.F.,.F.,(4,1,1,1,1,1,
1,4),(91.1061869541043,91.4272022140302,92.4248494727166,93.4224967314031,
94.4201439900896,95.4177912487761,96.4154385074626,97.3893722612839),
 .UNSPECIFIED.);
#2518=B_SPLINE_CURVE_WITH_KNOTS('',3,(#52355,#52356,#52357,#52358,#52359,
#52360,#52361,#52362,#52363,#52364,#52365),.UNSPECIFIED.,.F.,.F.,(4,1,1,
1,1,1,1,1,4),(91.1061869541044,91.1153093937187,92.1129566524052,93.1106039110917,
94.1082511697781,95.1058984284646,96.1035456871511,97.1011929458376,97.389372261284),
 .UNSPECIFIED.);
#2519=B_SPLINE_CURVE_WITH_KNOTS('',3,(#52370,#52371,#52372,#52373,#52374,
#52375,#52376,#52377,#52378,#52379),.UNSPECIFIED.,.F.,.F.,(4,1,1,1,1,1,
1,4),(84.8230016469247,85.4413186619112,86.4389659205977,87.4366131792842,
88.4342604379707,89.4319076966572,90.4295549553437,91.1061869541043),
 .UNSPECIFIED.);
#2520=B_SPLINE_CURVE_WITH_KNOTS('',3,(#52380,#52381,#52382,#52383,#52384,
#52385,#52386,#52387,#52388,#52389),.UNSPECIFIED.,.F.,.F.,(4,1,1,1,1,1,
1,4),(84.8230016469249,85.1294258415997,86.1270731002862,87.1247203589727,
88.1223676176592,89.1200148763457,90.1176621350322,91.1061869541044),
 .UNSPECIFIED.);
#2521=B_SPLINE_CURVE_WITH_KNOTS('',3,(#52394,#52395,#52396,#52397,#52398,
#52399,#52400,#52401,#52402,#52403),.UNSPECIFIED.,.F.,.F.,(4,1,1,1,1,1,
1,4),(78.5398163397451,79.4554351097923,80.4530823684788,81.4507296271653,
82.4483768858518,83.4460241445382,84.4436714032247,84.8230016469247),
 .UNSPECIFIED.);
#2522=B_SPLINE_CURVE_WITH_KNOTS('',3,(#52404,#52405,#52406,#52407,#52408,
#52409,#52410,#52411,#52412,#52413),.UNSPECIFIED.,.F.,.F.,(4,1,1,1,1,1,
1,4),(78.5398163397452,79.1435422894808,80.1411895481673,81.1388368068538,
82.1364840655403,83.1341313242268,84.1317785829133,84.8230016469249),
 .UNSPECIFIED.);
#2523=B_SPLINE_CURVE_WITH_KNOTS('',3,(#52418,#52419,#52420,#52421,#52422,
#52423,#52424,#52425,#52426,#52427,#52428),.UNSPECIFIED.,.F.,.F.,(4,1,1,
1,1,1,1,1,4),(72.2566310325655,72.4719042989869,73.4695515576734,74.4671988163598,
75.4648460750463,76.4624933337328,77.4601405924193,78.4577878511058,78.5398163397451),
 .UNSPECIFIED.);
#2524=B_SPLINE_CURVE_WITH_KNOTS('',3,(#52429,#52430,#52431,#52432,#52433,
#52434,#52435,#52436,#52437,#52438),.UNSPECIFIED.,.F.,.F.,(4,1,1,1,1,1,
1,4),(72.2566310325657,73.1576587373619,74.1553059960484,75.1529532547349,
76.1506005134213,77.1482477721078,78.1458950307943,78.5398163397452),
 .UNSPECIFIED.);
#2525=B_SPLINE_CURVE_WITH_KNOTS('',3,(#52443,#52444,#52445,#52446,#52447,
#52448,#52449,#52450,#52451,#52452),.UNSPECIFIED.,.F.,.F.,(4,1,1,1,1,1,
1,4),(65.9734457253859,66.4860207468679,67.4836680055544,68.4813152642409,
69.4789625229274,70.4766097816139,71.4742570403004,72.2566310325655),
 .UNSPECIFIED.);
#2526=B_SPLINE_CURVE_WITH_KNOTS('',3,(#52453,#52454,#52455,#52456,#52457,
#52458,#52459,#52460,#52461,#52462,#52463),.UNSPECIFIED.,.F.,.F.,(4,1,1,
1,1,1,1,1,4),(65.973445725386,66.1741279265564,67.1717751852429,68.1694224439294,
69.1670697026159,70.1647169613024,71.1623642199889,72.1600114786754,72.2566310325657),
 .UNSPECIFIED.);
#2527=B_SPLINE_CURVE_WITH_KNOTS('',3,(#52468,#52469,#52470,#52471,#52472,
#52473,#52474,#52475,#52476,#52477),.UNSPECIFIED.,.F.,.F.,(4,1,1,1,1,1,
1,4),(59.6902604182064,60.500137194749,61.4977844534355,62.495431712122,
63.4930789708085,64.490726229495,65.4883734881815,65.9734457253859),
 .UNSPECIFIED.);
#2528=B_SPLINE_CURVE_WITH_KNOTS('',3,(#52478,#52479,#52480,#52481,#52482,
#52483,#52484,#52485,#52486,#52487),.UNSPECIFIED.,.F.,.F.,(4,1,1,1,1,1,
1,4),(59.6902604182065,60.1882443744375,61.185891633124,62.1835388918105,
63.181186150497,64.1788334091835,65.17648066787,65.973445725386),
 .UNSPECIFIED.);
#2529=B_SPLINE_CURVE_WITH_KNOTS('',3,(#52492,#52493,#52494,#52495,#52496,
#52497,#52498,#52499,#52500,#52501,#52502),.UNSPECIFIED.,.F.,.F.,(4,1,1,
1,1,1,1,1,4),(53.4070751110267,53.5166063839436,54.5142536426301,55.5119009013166,
56.509548160003,57.5071954186895,58.504842677376,59.5024899360625,59.6902604182064),
 .UNSPECIFIED.);
#2530=B_SPLINE_CURVE_WITH_KNOTS('',3,(#52503,#52504,#52505,#52506,#52507,
#52508,#52509,#52510,#52511,#52512),.UNSPECIFIED.,.F.,.F.,(4,1,1,1,1,1,
1,4),(53.4070751110269,54.2023608223186,55.2000080810051,56.1976553396915,
57.195302598378,58.1929498570645,59.190597115751,59.6902604182065),
 .UNSPECIFIED.);
#2531=B_SPLINE_CURVE_WITH_KNOTS('',3,(#52517,#52518,#52519,#52520,#52521,
#52522,#52523,#52524,#52525,#52526),.UNSPECIFIED.,.F.,.F.,(4,1,1,1,1,1,
1,4),(47.1238898038472,47.5307228318246,48.5283700905111,49.5260173491976,
50.5236646078841,51.5213118665706,52.5189591252571,53.4070751110267),
 .UNSPECIFIED.);
#2532=B_SPLINE_CURVE_WITH_KNOTS('',3,(#52527,#52528,#52529,#52530,#52531,
#52532,#52533,#52534,#52535,#52536,#52537),.UNSPECIFIED.,.F.,.F.,(4,1,1,
1,1,1,1,1,4),(47.1238898038473,47.2188300115131,48.2164772701996,49.2141245288861,
50.2117717875726,51.2094190462591,52.2070663049456,53.2047135636321,53.4070751110269),
 .UNSPECIFIED.);
#2533=B_SPLINE_CURVE_WITH_KNOTS('',3,(#52542,#52543,#52544,#52545,#52546,
#52547,#52548,#52549,#52550,#52551),.UNSPECIFIED.,.F.,.F.,(4,1,1,1,1,1,
1,4),(40.8407044966676,41.5448392797057,42.5424865383922,43.5401337970787,
44.5377810557652,45.5354283144517,46.5330755731381,47.1238898038472),
 .UNSPECIFIED.);
#2534=B_SPLINE_CURVE_WITH_KNOTS('',3,(#52552,#52553,#52554,#52555,#52556,
#52557,#52558,#52559,#52560,#52561),.UNSPECIFIED.,.F.,.F.,(4,1,1,1,1,1,
1,4),(40.8407044966677,41.2329464593942,42.2305937180807,43.2282409767672,
44.2258882354537,45.2235354941402,46.2211827528266,47.1238898038473),
 .UNSPECIFIED.);
#2535=B_SPLINE_CURVE_WITH_KNOTS('',3,(#52566,#52567,#52568,#52569,#52570,
#52571,#52572,#52573,#52574,#52575,#52576),.UNSPECIFIED.,.F.,.F.,(4,1,1,
1,1,1,1,1,4),(34.557519189488,34.5613084689003,35.5589557275868,36.5566029862733,
37.5542502449598,38.5518975036462,39.5495447623327,40.5471920210192,40.8407044966676),
 .UNSPECIFIED.);
#2536=B_SPLINE_CURVE_WITH_KNOTS('',3,(#52577,#52578,#52579,#52580,#52581,
#52582,#52583,#52584,#52585,#52586),.UNSPECIFIED.,.F.,.F.,(4,1,1,1,1,1,
1,4),(34.5575191894881,35.2470629072753,36.2447101659618,37.2423574246482,
38.2400046833347,39.2376519420212,40.2352992007077,40.8407044966677),
 .UNSPECIFIED.);
#2537=B_SPLINE_CURVE_WITH_KNOTS('',3,(#52591,#52592,#52593,#52594,#52595,
#52596,#52597,#52598,#52599,#52600),.UNSPECIFIED.,.F.,.F.,(4,1,1,1,1,1,
1,4),(28.2743338823084,28.5754249167814,29.5730721754678,30.5707194341543,
31.5683666928408,32.5660139515273,33.5636612102138,34.557519189488),
 .UNSPECIFIED.);
#2538=B_SPLINE_CURVE_WITH_KNOTS('',3,(#52601,#52602,#52603,#52604,#52605,
#52606,#52607,#52608,#52609,#52610),.UNSPECIFIED.,.F.,.F.,(4,1,1,1,1,1,
1,4),(28.2743338823085,29.2611793551563,30.2588266138428,31.2564738725293,
32.2541211312158,33.2517683899023,34.2494156485888,34.5575191894881),
 .UNSPECIFIED.);
#2539=B_SPLINE_CURVE_WITH_KNOTS('',3,(#52615,#52616,#52617,#52618,#52619,
#52620,#52621,#52622,#52623,#52624),.UNSPECIFIED.,.F.,.F.,(4,1,1,1,1,1,
1,4),(21.9911485751288,22.5895413646624,23.5871886233489,24.5848358820354,
25.5824831407219,26.5801303994084,27.5777776580949,28.2743338823084),
 .UNSPECIFIED.);
#2540=B_SPLINE_CURVE_WITH_KNOTS('',3,(#52625,#52626,#52627,#52628,#52629,
#52630,#52631,#52632,#52633,#52634,#52635),.UNSPECIFIED.,.F.,.F.,(4,1,1,
1,1,1,1,1,4),(21.9911485751289,22.2776485443509,23.2752958030374,24.2729430617239,
25.2705903204104,26.2682375790969,27.2658848377834,28.2635320964698,28.2743338823085),
 .UNSPECIFIED.);
#2541=B_SPLINE_CURVE_WITH_KNOTS('',3,(#52640,#52641,#52642,#52643,#52644,
#52645,#52646,#52647,#52648,#52649),.UNSPECIFIED.,.F.,.F.,(4,1,1,1,1,1,
1,4),(15.7079632679492,16.6036578125435,17.60130507123,18.5989523299165,
19.596599588603,20.5942468472894,21.5918941059759,21.9911485751288),
 .UNSPECIFIED.);
#2542=B_SPLINE_CURVE_WITH_KNOTS('',3,(#52650,#52651,#52652,#52653,#52654,
#52655,#52656,#52657,#52658,#52659),.UNSPECIFIED.,.F.,.F.,(4,1,1,1,1,1,
1,4),(15.7079632679493,16.291764992232,17.2894122509185,18.2870595096049,
19.2847067682914,20.2823540269779,21.2800012856644,21.9911485751289),
 .UNSPECIFIED.);
#2543=B_SPLINE_CURVE_WITH_KNOTS('',3,(#52662,#52663,#52664,#52665,#52666,
#52667,#52668,#52669,#52670,#52671,#52672,#52673,#52674,#52675,#52676,#52677,
#52678,#52679,#52680,#52681,#52682,#52683,#52684,#52685,#52686,#52687,#52688,
#52689,#52690,#52691,#52692,#52693,#52694,#52695,#52696,#52697,#52698,#52699,
#52700,#52701,#52702,#52703,#52704,#52705,#52706,#52707,#52708,#52709,#52710,
#52711,#52712,#52713,#52714,#52715,#52716,#52717,#52718,#52719,#52720,#52721,
#52722,#52723,#52724,#52725,#52726,#52727,#52728,#52729,#52730,#52731,#52732,
#52733,#52734,#52735,#52736,#52737,#52738,#52739,#52740,#52741,#52742,#52743,
#52744,#52745,#52746),.UNSPECIFIED.,.F.,.F.,(4,3,3,3,3,3,3,3,3,3,3,3,3,
3,3,3,3,3,3,3,3,3,3,3,3,3,3,3,4),(-0.366397579005864,-0.355346843401997,
-0.337374205212124,-0.327023766356039,-0.321660460620163,-0.302852850386516,
-0.288389399635472,-0.281253803741762,-0.277593082466284,-0.258152985974441,
-0.238335747277564,-0.225538121552714,-0.218338269767891,-0.214826360536685,
-0.194396506267918,-0.187145244378166,-0.167439047158832,-0.156805333697672,
-0.149254241972043,-0.145835187513462,-0.125406703312949,-0.104529747281994,
-0.0834620766624818,-0.0752632118999826,-0.0721348992869,-0.0504908701427557,
-0.0287975712486206,-0.00756831909181192,0.),.UNSPECIFIED.);
#2544=B_SPLINE_CURVE_WITH_KNOTS('',3,(#52749,#52750,#52751,#52752,#52753,
#52754,#52755,#52756,#52757,#52758,#52759,#52760,#52761,#52762,#52763,#52764,
#52765,#52766,#52767,#52768,#52769,#52770,#52771,#52772,#52773,#52774,#52775,
#52776,#52777,#52778,#52779,#52780,#52781,#52782,#52783,#52784,#52785,#52786,
#52787,#52788,#52789,#52790,#52791,#52792,#52793,#52794,#52795,#52796,#52797,
#52798,#52799,#52800,#52801,#52802,#52803,#52804,#52805,#52806,#52807,#52808,
#52809,#52810,#52811,#52812,#52813,#52814,#52815,#52816,#52817,#52818,#52819,
#52820,#52821,#52822,#52823,#52824,#52825,#52826,#52827,#52828,#52829,#52830,
#52831,#52832,#52833),.UNSPECIFIED.,.F.,.F.,(4,3,3,3,3,3,3,3,3,3,3,3,3,
3,3,3,3,3,3,3,3,3,3,3,3,3,3,3,4),(-0.364629307890682,-0.351006911521526,
-0.329419062578797,-0.319153222372462,-0.313799294766335,-0.309381194149429,
-0.28805875991114,-0.272829974986374,-0.264051709713518,-0.260308217235067,
-0.239577131076176,-0.219357140458664,-0.206074975472251,-0.194939029035285,
-0.191413094196265,-0.171827379537648,-0.166228480513009,-0.145449920448883,
-0.126802705425088,-0.123658925074466,-0.104206162927893,-0.0848250947771817,
-0.0658374354857542,-0.0621954187504667,-0.0590783926424019,-0.0404862701271266,
-0.0222276738045438,-0.00455247856545703,0.),.UNSPECIFIED.);
#2545=B_SPLINE_CURVE_WITH_KNOTS('',3,(#53914,#53915,#53916,#53917,#53918,
#53919,#53920,#53921,#53922,#53923,#53924,#53925,#53926,#53927,#53928,#53929,
#53930,#53931,#53932),.UNSPECIFIED.,.F.,.F.,(4,3,3,3,3,3,4),(258.724788632393,
259.388287258487,260.385934517174,261.38358177586,262.381229034547,263.378876293233,
264.306677936014),.UNSPECIFIED.);
#2546=B_SPLINE_CURVE_WITH_KNOTS('',3,(#53934,#53935,#53936,#53937,#53938,
#53939,#53940,#53941,#53942,#53943,#53944,#53945,#53946,#53947,#53948,#53949,
#53950,#53951,#53952,#53953,#53954,#53955,#53956,#53957,#53958,#53959,#53960,
#53961,#53962,#53963,#53964,#53965,#53966,#53967,#53968,#53969,#53970,#53971,
#53972,#53973,#53974,#53975,#53976,#53977,#53978,#53979,#53980,#53981,#53982,
#53983,#53984,#53985,#53986,#53987,#53988,#53989,#53990,#53991,#53992,#53993,
#53994,#53995,#53996,#53997,#53998,#53999,#54000,#54001,#54002,#54003,#54004,
#54005,#54006,#54007,#54008,#54009,#54010,#54011,#54012,#54013,#54014,#54015,
#54016,#54017,#54018),.UNSPECIFIED.,.F.,.F.,(4,3,3,3,3,3,3,3,3,3,3,3,3,
3,3,3,3,3,3,3,3,3,3,3,3,3,3,3,4),(-0.366397579005823,-0.355346843401945,
-0.337374208775006,-0.327023772701273,-0.321660460826443,-0.302852852909943,
-0.288389401843468,-0.281253813336682,-0.277593084937738,-0.258152990277808,
-0.238335751411466,-0.225538124653135,-0.218338277322973,-0.214826365031749,
-0.19439651065702,-0.187145244378141,-0.167439048322423,-0.156805335511694,
-0.149254246961296,-0.145835189834807,-0.125406707076156,-0.104529752607351,
-0.0834620823221285,-0.0752632122609285,-0.0721348995369247,-0.0504908714072708,
-0.0287975717539159,-0.00756831536751696,0.),.UNSPECIFIED.);
#2547=B_SPLINE_CURVE_WITH_KNOTS('',3,(#54019,#54020,#54021,#54022,#54023,
#54024,#54025,#54026,#54027),.UNSPECIFIED.,.F.,.F.,(4,1,1,1,1,1,4),(10.3757270560183,
11.3035286987995,12.301175957486,13.2988232161725,14.296470474859,15.2941177335455,
15.7079632679493),.UNSPECIFIED.);
#2548=B_SPLINE_CURVE_WITH_KNOTS('',3,(#54033,#54034,#54035,#54036,#54037,
#54038,#54039,#54040,#54041,#54042,#54043,#54044,#54045,#54046,#54047,#54048,
#54049,#54050,#54051,#54052,#54053,#54054,#54055,#54056,#54057,#54058,#54059,
#54060,#54061,#54062,#54063,#54064,#54065,#54066,#54067,#54068,#54069,#54070,
#54071,#54072,#54073,#54074,#54075,#54076,#54077,#54078,#54079,#54080,#54081,
#54082,#54083,#54084,#54085,#54086,#54087,#54088,#54089,#54090,#54091,#54092,
#54093,#54094,#54095,#54096,#54097,#54098,#54099,#54100,#54101,#54102,#54103,
#54104,#54105,#54106,#54107,#54108,#54109,#54110,#54111,#54112,#54113,#54114,
#54115,#54116,#54117),.UNSPECIFIED.,.F.,.F.,(4,3,3,3,3,3,3,3,3,3,3,3,3,
3,3,3,3,3,3,3,3,3,3,3,3,3,3,3,4),(-0.364629307890672,-0.351006911521527,
-0.329419062483496,-0.319153221480068,-0.313799274448012,-0.309381188300517,
-0.288058753940656,-0.272829969762204,-0.264051699307754,-0.260308214521764,
-0.23957712793709,-0.219357134376034,-0.206074970910285,-0.194939021602606,
-0.191413092807867,-0.171827375216207,-0.166228480513036,-0.145449920448906,
-0.12680270395916,-0.123658922471174,-0.104206159570983,-0.0848250934702219,
-0.0658374384621282,-0.0621954412209474,-0.0590784413626975,-0.040486321224885,
-0.022227728381574,-0.00455253779193712,0.),.UNSPECIFIED.);
#2549=B_SPLINE_CURVE_WITH_KNOTS('',3,(#54120,#54121,#54122,#54123,#54124,
#54125,#54126,#54127),.UNSPECIFIED.,.F.,.F.,(4,1,1,1,1,4),(11.615421519111,
12.6130687777975,13.610716036484,14.6083632951705,15.606010553857,15.7079632679492),
 .UNSPECIFIED.);
#2550=B_SPLINE_CURVE_WITH_KNOTS('',3,(#55208,#55209,#55210,#55211,#55212,
#55213,#55214,#55215,#55216,#55217,#55218,#55219,#55220,#55221,#55222,#55223),
 .UNSPECIFIED.,.F.,.F.,(4,3,3,3,3,4),(-266.371818069293,-265.374170810606,
-264.37652355192,-263.378876293233,-262.381229034547,-261.703139343201),
 .UNSPECIFIED.);
#3488=FACE_BOUND('',#6442,.T.);
#3489=FACE_BOUND('',#6595,.T.);
#3490=FACE_BOUND('',#6599,.T.);
#3491=FACE_BOUND('',#6600,.T.);
#3492=FACE_BOUND('',#6601,.T.);
#3493=FACE_BOUND('',#6602,.T.);
#3494=FACE_BOUND('',#6603,.T.);
#3495=FACE_BOUND('',#6604,.T.);
#3496=FACE_BOUND('',#6605,.T.);
#3497=FACE_BOUND('',#6606,.T.);
#3498=FACE_BOUND('',#6607,.T.);
#3499=FACE_BOUND('',#6608,.T.);
#3500=FACE_BOUND('',#6609,.T.);
#3501=FACE_BOUND('',#6610,.T.);
#3502=FACE_BOUND('',#6611,.T.);
#3503=FACE_BOUND('',#6612,.T.);
#3504=FACE_BOUND('',#6613,.T.);
#3505=FACE_BOUND('',#6614,.T.);
#3506=FACE_BOUND('',#6615,.T.);
#3507=FACE_BOUND('',#6616,.T.);
#3508=FACE_BOUND('',#6617,.T.);
#3509=FACE_BOUND('',#6618,.T.);
#3510=FACE_BOUND('',#6619,.T.);
#3511=FACE_BOUND('',#6620,.T.);
#3512=FACE_BOUND('',#6621,.T.);
#3513=FACE_BOUND('',#6622,.T.);
#3514=FACE_BOUND('',#6623,.T.);
#3515=FACE_BOUND('',#6624,.T.);
#3516=FACE_BOUND('',#6625,.T.);
#3517=FACE_BOUND('',#6626,.T.);
#3518=FACE_BOUND('',#6627,.T.);
#3519=FACE_BOUND('',#6628,.T.);
#3520=FACE_BOUND('',#6629,.T.);
#3521=FACE_BOUND('',#6630,.T.);
#3522=FACE_BOUND('',#6631,.T.);
#3523=FACE_BOUND('',#6632,.T.);
#3524=FACE_BOUND('',#6633,.T.);
#3525=FACE_BOUND('',#6636,.T.);
#4390=FACE_OUTER_BOUND('',#6350,.T.);
#4391=FACE_OUTER_BOUND('',#6351,.T.);
#4392=FACE_OUTER_BOUND('',#6352,.T.);
#4393=FACE_OUTER_BOUND('',#6353,.T.);
#4394=FACE_OUTER_BOUND('',#6354,.T.);
#4395=FACE_OUTER_BOUND('',#6355,.T.);
#4396=FACE_OUTER_BOUND('',#6356,.T.);
#4397=FACE_OUTER_BOUND('',#6357,.T.);
#4398=FACE_OUTER_BOUND('',#6358,.T.);
#4399=FACE_OUTER_BOUND('',#6359,.T.);
#4400=FACE_OUTER_BOUND('',#6360,.T.);
#4401=FACE_OUTER_BOUND('',#6361,.T.);
#4402=FACE_OUTER_BOUND('',#6362,.T.);
#4403=FACE_OUTER_BOUND('',#6363,.T.);
#4404=FACE_OUTER_BOUND('',#6364,.T.);
#4405=FACE_OUTER_BOUND('',#6365,.T.);
#4406=FACE_OUTER_BOUND('',#6366,.T.);
#4407=FACE_OUTER_BOUND('',#6367,.T.);
#4408=FACE_OUTER_BOUND('',#6368,.T.);
#4409=FACE_OUTER_BOUND('',#6369,.T.);
#4410=FACE_OUTER_BOUND('',#6370,.T.);
#4411=FACE_OUTER_BOUND('',#6371,.T.);
#4412=FACE_OUTER_BOUND('',#6372,.T.);
#4413=FACE_OUTER_BOUND('',#6373,.T.);
#4414=FACE_OUTER_BOUND('',#6374,.T.);
#4415=FACE_OUTER_BOUND('',#6375,.T.);
#4416=FACE_OUTER_BOUND('',#6376,.T.);
#4417=FACE_OUTER_BOUND('',#6377,.T.);
#4418=FACE_OUTER_BOUND('',#6378,.T.);
#4419=FACE_OUTER_BOUND('',#6379,.T.);
#4420=FACE_OUTER_BOUND('',#6380,.T.);
#4421=FACE_OUTER_BOUND('',#6381,.T.);
#4422=FACE_OUTER_BOUND('',#6382,.T.);
#4423=FACE_OUTER_BOUND('',#6383,.T.);
#4424=FACE_OUTER_BOUND('',#6384,.T.);
#4425=FACE_OUTER_BOUND('',#6385,.T.);
#4426=FACE_OUTER_BOUND('',#6386,.T.);
#4427=FACE_OUTER_BOUND('',#6387,.T.);
#4428=FACE_OUTER_BOUND('',#6388,.T.);
#4429=FACE_OUTER_BOUND('',#6389,.T.);
#4430=FACE_OUTER_BOUND('',#6390,.T.);
#4431=FACE_OUTER_BOUND('',#6391,.T.);
#4432=FACE_OUTER_BOUND('',#6392,.T.);
#4433=FACE_OUTER_BOUND('',#6393,.T.);
#4434=FACE_OUTER_BOUND('',#6394,.T.);
#4435=FACE_OUTER_BOUND('',#6395,.T.);
#4436=FACE_OUTER_BOUND('',#6396,.T.);
#4437=FACE_OUTER_BOUND('',#6397,.T.);
#4438=FACE_OUTER_BOUND('',#6398,.T.);
#4439=FACE_OUTER_BOUND('',#6399,.T.);
#4440=FACE_OUTER_BOUND('',#6400,.T.);
#4441=FACE_OUTER_BOUND('',#6401,.T.);
#4442=FACE_OUTER_BOUND('',#6402,.T.);
#4443=FACE_OUTER_BOUND('',#6403,.T.);
#4444=FACE_OUTER_BOUND('',#6404,.T.);
#4445=FACE_OUTER_BOUND('',#6405,.T.);
#4446=FACE_OUTER_BOUND('',#6406,.T.);
#4447=FACE_OUTER_BOUND('',#6407,.T.);
#4448=FACE_OUTER_BOUND('',#6408,.T.);
#4449=FACE_OUTER_BOUND('',#6409,.T.);
#4450=FACE_OUTER_BOUND('',#6410,.T.);
#4451=FACE_OUTER_BOUND('',#6411,.T.);
#4452=FACE_OUTER_BOUND('',#6412,.T.);
#4453=FACE_OUTER_BOUND('',#6413,.T.);
#4454=FACE_OUTER_BOUND('',#6414,.T.);
#4455=FACE_OUTER_BOUND('',#6415,.T.);
#4456=FACE_OUTER_BOUND('',#6416,.T.);
#4457=FACE_OUTER_BOUND('',#6417,.T.);
#4458=FACE_OUTER_BOUND('',#6418,.T.);
#4459=FACE_OUTER_BOUND('',#6419,.T.);
#4460=FACE_OUTER_BOUND('',#6420,.T.);
#4461=FACE_OUTER_BOUND('',#6421,.T.);
#4462=FACE_OUTER_BOUND('',#6422,.T.);
#4463=FACE_OUTER_BOUND('',#6423,.T.);
#4464=FACE_OUTER_BOUND('',#6424,.T.);
#4465=FACE_OUTER_BOUND('',#6425,.T.);
#4466=FACE_OUTER_BOUND('',#6426,.T.);
#4467=FACE_OUTER_BOUND('',#6427,.T.);
#4468=FACE_OUTER_BOUND('',#6428,.T.);
#4469=FACE_OUTER_BOUND('',#6429,.T.);
#4470=FACE_OUTER_BOUND('',#6430,.T.);
#4471=FACE_OUTER_BOUND('',#6431,.T.);
#4472=FACE_OUTER_BOUND('',#6432,.T.);
#4473=FACE_OUTER_BOUND('',#6433,.T.);
#4474=FACE_OUTER_BOUND('',#6434,.T.);
#4475=FACE_OUTER_BOUND('',#6435,.T.);
#4476=FACE_OUTER_BOUND('',#6436,.T.);
#4477=FACE_OUTER_BOUND('',#6437,.T.);
#4478=FACE_OUTER_BOUND('',#6438,.T.);
#4479=FACE_OUTER_BOUND('',#6439,.T.);
#4480=FACE_OUTER_BOUND('',#6440,.T.);
#4481=FACE_OUTER_BOUND('',#6441,.T.);
#4482=FACE_OUTER_BOUND('',#6443,.T.);
#4483=FACE_OUTER_BOUND('',#6444,.T.);
#4484=FACE_OUTER_BOUND('',#6445,.T.);
#4485=FACE_OUTER_BOUND('',#6446,.T.);
#4486=FACE_OUTER_BOUND('',#6447,.T.);
#4487=FACE_OUTER_BOUND('',#6448,.T.);
#4488=FACE_OUTER_BOUND('',#6449,.T.);
#4489=FACE_OUTER_BOUND('',#6450,.T.);
#4490=FACE_OUTER_BOUND('',#6451,.T.);
#4491=FACE_OUTER_BOUND('',#6452,.T.);
#4492=FACE_OUTER_BOUND('',#6453,.T.);
#4493=FACE_OUTER_BOUND('',#6454,.T.);
#4494=FACE_OUTER_BOUND('',#6455,.T.);
#4495=FACE_OUTER_BOUND('',#6456,.T.);
#4496=FACE_OUTER_BOUND('',#6457,.T.);
#4497=FACE_OUTER_BOUND('',#6458,.T.);
#4498=FACE_OUTER_BOUND('',#6459,.T.);
#4499=FACE_OUTER_BOUND('',#6460,.T.);
#4500=FACE_OUTER_BOUND('',#6461,.T.);
#4501=FACE_OUTER_BOUND('',#6462,.T.);
#4502=FACE_OUTER_BOUND('',#6463,.T.);
#4503=FACE_OUTER_BOUND('',#6464,.T.);
#4504=FACE_OUTER_BOUND('',#6465,.T.);
#4505=FACE_OUTER_BOUND('',#6466,.T.);
#4506=FACE_OUTER_BOUND('',#6467,.T.);
#4507=FACE_OUTER_BOUND('',#6468,.T.);
#4508=FACE_OUTER_BOUND('',#6469,.T.);
#4509=FACE_OUTER_BOUND('',#6470,.T.);
#4510=FACE_OUTER_BOUND('',#6471,.T.);
#4511=FACE_OUTER_BOUND('',#6472,.T.);
#4512=FACE_OUTER_BOUND('',#6473,.T.);
#4513=FACE_OUTER_BOUND('',#6474,.T.);
#4514=FACE_OUTER_BOUND('',#6475,.T.);
#4515=FACE_OUTER_BOUND('',#6476,.T.);
#4516=FACE_OUTER_BOUND('',#6477,.T.);
#4517=FACE_OUTER_BOUND('',#6478,.T.);
#4518=FACE_OUTER_BOUND('',#6479,.T.);
#4519=FACE_OUTER_BOUND('',#6480,.T.);
#4520=FACE_OUTER_BOUND('',#6481,.T.);
#4521=FACE_OUTER_BOUND('',#6482,.T.);
#4522=FACE_OUTER_BOUND('',#6483,.T.);
#4523=FACE_OUTER_BOUND('',#6484,.T.);
#4524=FACE_OUTER_BOUND('',#6485,.T.);
#4525=FACE_OUTER_BOUND('',#6486,.T.);
#4526=FACE_OUTER_BOUND('',#6487,.T.);
#4527=FACE_OUTER_BOUND('',#6488,.T.);
#4528=FACE_OUTER_BOUND('',#6489,.T.);
#4529=FACE_OUTER_BOUND('',#6490,.T.);
#4530=FACE_OUTER_BOUND('',#6491,.T.);
#4531=FACE_OUTER_BOUND('',#6492,.T.);
#4532=FACE_OUTER_BOUND('',#6493,.T.);
#4533=FACE_OUTER_BOUND('',#6494,.T.);
#4534=FACE_OUTER_BOUND('',#6495,.T.);
#4535=FACE_OUTER_BOUND('',#6496,.T.);
#4536=FACE_OUTER_BOUND('',#6497,.T.);
#4537=FACE_OUTER_BOUND('',#6498,.T.);
#4538=FACE_OUTER_BOUND('',#6499,.T.);
#4539=FACE_OUTER_BOUND('',#6500,.T.);
#4540=FACE_OUTER_BOUND('',#6501,.T.);
#4541=FACE_OUTER_BOUND('',#6502,.T.);
#4542=FACE_OUTER_BOUND('',#6503,.T.);
#4543=FACE_OUTER_BOUND('',#6504,.T.);
#4544=FACE_OUTER_BOUND('',#6505,.T.);
#4545=FACE_OUTER_BOUND('',#6506,.T.);
#4546=FACE_OUTER_BOUND('',#6507,.T.);
#4547=FACE_OUTER_BOUND('',#6508,.T.);
#4548=FACE_OUTER_BOUND('',#6509,.T.);
#4549=FACE_OUTER_BOUND('',#6510,.T.);
#4550=FACE_OUTER_BOUND('',#6511,.T.);
#4551=FACE_OUTER_BOUND('',#6512,.T.);
#4552=FACE_OUTER_BOUND('',#6513,.T.);
#4553=FACE_OUTER_BOUND('',#6514,.T.);
#4554=FACE_OUTER_BOUND('',#6515,.T.);
#4555=FACE_OUTER_BOUND('',#6516,.T.);
#4556=FACE_OUTER_BOUND('',#6517,.T.);
#4557=FACE_OUTER_BOUND('',#6518,.T.);
#4558=FACE_OUTER_BOUND('',#6519,.T.);
#4559=FACE_OUTER_BOUND('',#6520,.T.);
#4560=FACE_OUTER_BOUND('',#6521,.T.);
#4561=FACE_OUTER_BOUND('',#6522,.T.);
#4562=FACE_OUTER_BOUND('',#6523,.T.);
#4563=FACE_OUTER_BOUND('',#6524,.T.);
#4564=FACE_OUTER_BOUND('',#6525,.T.);
#4565=FACE_OUTER_BOUND('',#6526,.T.);
#4566=FACE_OUTER_BOUND('',#6527,.T.);
#4567=FACE_OUTER_BOUND('',#6528,.T.);
#4568=FACE_OUTER_BOUND('',#6529,.T.);
#4569=FACE_OUTER_BOUND('',#6530,.T.);
#4570=FACE_OUTER_BOUND('',#6531,.T.);
#4571=FACE_OUTER_BOUND('',#6532,.T.);
#4572=FACE_OUTER_BOUND('',#6533,.T.);
#4573=FACE_OUTER_BOUND('',#6534,.T.);
#4574=FACE_OUTER_BOUND('',#6535,.T.);
#4575=FACE_OUTER_BOUND('',#6536,.T.);
#4576=FACE_OUTER_BOUND('',#6537,.T.);
#4577=FACE_OUTER_BOUND('',#6538,.T.);
#4578=FACE_OUTER_BOUND('',#6539,.T.);
#4579=FACE_OUTER_BOUND('',#6540,.T.);
#4580=FACE_OUTER_BOUND('',#6541,.T.);
#4581=FACE_OUTER_BOUND('',#6542,.T.);
#4582=FACE_OUTER_BOUND('',#6543,.T.);
#4583=FACE_OUTER_BOUND('',#6544,.T.);
#4584=FACE_OUTER_BOUND('',#6545,.T.);
#4585=FACE_OUTER_BOUND('',#6546,.T.);
#4586=FACE_OUTER_BOUND('',#6547,.T.);
#4587=FACE_OUTER_BOUND('',#6548,.T.);
#4588=FACE_OUTER_BOUND('',#6549,.T.);
#4589=FACE_OUTER_BOUND('',#6550,.T.);
#4590=FACE_OUTER_BOUND('',#6551,.T.);
#4591=FACE_OUTER_BOUND('',#6552,.T.);
#4592=FACE_OUTER_BOUND('',#6553,.T.);
#4593=FACE_OUTER_BOUND('',#6554,.T.);
#4594=FACE_OUTER_BOUND('',#6555,.T.);
#4595=FACE_OUTER_BOUND('',#6556,.T.);
#4596=FACE_OUTER_BOUND('',#6557,.T.);
#4597=FACE_OUTER_BOUND('',#6558,.T.);
#4598=FACE_OUTER_BOUND('',#6559,.T.);
#4599=FACE_OUTER_BOUND('',#6560,.T.);
#4600=FACE_OUTER_BOUND('',#6561,.T.);
#4601=FACE_OUTER_BOUND('',#6562,.T.);
#4602=FACE_OUTER_BOUND('',#6563,.T.);
#4603=FACE_OUTER_BOUND('',#6564,.T.);
#4604=FACE_OUTER_BOUND('',#6565,.T.);
#4605=FACE_OUTER_BOUND('',#6566,.T.);
#4606=FACE_OUTER_BOUND('',#6567,.T.);
#4607=FACE_OUTER_BOUND('',#6568,.T.);
#4608=FACE_OUTER_BOUND('',#6569,.T.);
#4609=FACE_OUTER_BOUND('',#6570,.T.);
#4610=FACE_OUTER_BOUND('',#6571,.T.);
#4611=FACE_OUTER_BOUND('',#6572,.T.);
#4612=FACE_OUTER_BOUND('',#6573,.T.);
#4613=FACE_OUTER_BOUND('',#6574,.T.);
#4614=FACE_OUTER_BOUND('',#6575,.T.);
#4615=FACE_OUTER_BOUND('',#6576,.T.);
#4616=FACE_OUTER_BOUND('',#6577,.T.);
#4617=FACE_OUTER_BOUND('',#6578,.T.);
#4618=FACE_OUTER_BOUND('',#6579,.T.);
#4619=FACE_OUTER_BOUND('',#6580,.T.);
#4620=FACE_OUTER_BOUND('',#6581,.T.);
#4621=FACE_OUTER_BOUND('',#6582,.T.);
#4622=FACE_OUTER_BOUND('',#6583,.T.);
#4623=FACE_OUTER_BOUND('',#6584,.T.);
#4624=FACE_OUTER_BOUND('',#6585,.T.);
#4625=FACE_OUTER_BOUND('',#6586,.T.);
#4626=FACE_OUTER_BOUND('',#6587,.T.);
#4627=FACE_OUTER_BOUND('',#6588,.T.);
#4628=FACE_OUTER_BOUND('',#6589,.T.);
#4629=FACE_OUTER_BOUND('',#6590,.T.);
#4630=FACE_OUTER_BOUND('',#6591,.T.);
#4631=FACE_OUTER_BOUND('',#6592,.T.);
#4632=FACE_OUTER_BOUND('',#6593,.T.);
#4633=FACE_OUTER_BOUND('',#6594,.T.);
#4634=FACE_OUTER_BOUND('',#6596,.T.);
#4635=FACE_OUTER_BOUND('',#6597,.T.);
#4636=FACE_OUTER_BOUND('',#6598,.T.);
#4637=FACE_OUTER_BOUND('',#6634,.T.);
#4638=FACE_OUTER_BOUND('',#6635,.T.);
#6350=EDGE_LOOP('',(#23083,#23084,#23085,#23086));
#6351=EDGE_LOOP('',(#23087,#23088,#23089,#23090));
#6352=EDGE_LOOP('',(#23091,#23092,#23093,#23094));
#6353=EDGE_LOOP('',(#23095,#23096,#23097,#23098));
#6354=EDGE_LOOP('',(#23099,#23100,#23101,#23102));
#6355=EDGE_LOOP('',(#23103,#23104,#23105,#23106));
#6356=EDGE_LOOP('',(#23107,#23108,#23109,#23110));
#6357=EDGE_LOOP('',(#23111,#23112,#23113,#23114));
#6358=EDGE_LOOP('',(#23115,#23116,#23117,#23118));
#6359=EDGE_LOOP('',(#23119,#23120,#23121,#23122));
#6360=EDGE_LOOP('',(#23123,#23124,#23125,#23126));
#6361=EDGE_LOOP('',(#23127,#23128,#23129,#23130));
#6362=EDGE_LOOP('',(#23131,#23132,#23133,#23134));
#6363=EDGE_LOOP('',(#23135,#23136,#23137,#23138));
#6364=EDGE_LOOP('',(#23139,#23140,#23141,#23142));
#6365=EDGE_LOOP('',(#23143,#23144,#23145,#23146));
#6366=EDGE_LOOP('',(#23147,#23148,#23149,#23150));
#6367=EDGE_LOOP('',(#23151,#23152,#23153,#23154));
#6368=EDGE_LOOP('',(#23155,#23156,#23157,#23158));
#6369=EDGE_LOOP('',(#23159,#23160,#23161,#23162));
#6370=EDGE_LOOP('',(#23163,#23164,#23165,#23166));
#6371=EDGE_LOOP('',(#23167,#23168,#23169,#23170));
#6372=EDGE_LOOP('',(#23171,#23172,#23173,#23174));
#6373=EDGE_LOOP('',(#23175,#23176,#23177,#23178));
#6374=EDGE_LOOP('',(#23179,#23180,#23181,#23182));
#6375=EDGE_LOOP('',(#23183,#23184,#23185,#23186));
#6376=EDGE_LOOP('',(#23187,#23188,#23189,#23190));
#6377=EDGE_LOOP('',(#23191,#23192,#23193,#23194));
#6378=EDGE_LOOP('',(#23195,#23196,#23197,#23198));
#6379=EDGE_LOOP('',(#23199,#23200,#23201,#23202));
#6380=EDGE_LOOP('',(#23203,#23204,#23205,#23206));
#6381=EDGE_LOOP('',(#23207,#23208,#23209,#23210));
#6382=EDGE_LOOP('',(#23211,#23212,#23213,#23214));
#6383=EDGE_LOOP('',(#23215,#23216,#23217,#23218));
#6384=EDGE_LOOP('',(#23219,#23220,#23221,#23222));
#6385=EDGE_LOOP('',(#23223,#23224,#23225,#23226));
#6386=EDGE_LOOP('',(#23227,#23228,#23229,#23230));
#6387=EDGE_LOOP('',(#23231,#23232,#23233,#23234));
#6388=EDGE_LOOP('',(#23235,#23236,#23237,#23238));
#6389=EDGE_LOOP('',(#23239,#23240,#23241,#23242));
#6390=EDGE_LOOP('',(#23243,#23244,#23245,#23246));
#6391=EDGE_LOOP('',(#23247,#23248,#23249,#23250));
#6392=EDGE_LOOP('',(#23251,#23252,#23253,#23254));
#6393=EDGE_LOOP('',(#23255,#23256,#23257,#23258));
#6394=EDGE_LOOP('',(#23259,#23260,#23261,#23262));
#6395=EDGE_LOOP('',(#23263,#23264,#23265,#23266));
#6396=EDGE_LOOP('',(#23267,#23268,#23269,#23270));
#6397=EDGE_LOOP('',(#23271,#23272,#23273,#23274));
#6398=EDGE_LOOP('',(#23275,#23276,#23277,#23278));
#6399=EDGE_LOOP('',(#23279,#23280,#23281,#23282));
#6400=EDGE_LOOP('',(#23283,#23284,#23285,#23286));
#6401=EDGE_LOOP('',(#23287,#23288,#23289,#23290));
#6402=EDGE_LOOP('',(#23291,#23292,#23293,#23294));
#6403=EDGE_LOOP('',(#23295,#23296,#23297,#23298));
#6404=EDGE_LOOP('',(#23299,#23300,#23301,#23302));
#6405=EDGE_LOOP('',(#23303,#23304,#23305,#23306));
#6406=EDGE_LOOP('',(#23307,#23308,#23309,#23310));
#6407=EDGE_LOOP('',(#23311,#23312,#23313,#23314));
#6408=EDGE_LOOP('',(#23315,#23316,#23317,#23318));
#6409=EDGE_LOOP('',(#23319,#23320,#23321,#23322));
#6410=EDGE_LOOP('',(#23323,#23324,#23325,#23326));
#6411=EDGE_LOOP('',(#23327,#23328,#23329,#23330));
#6412=EDGE_LOOP('',(#23331,#23332,#23333,#23334));
#6413=EDGE_LOOP('',(#23335,#23336,#23337,#23338));
#6414=EDGE_LOOP('',(#23339,#23340,#23341,#23342));
#6415=EDGE_LOOP('',(#23343,#23344,#23345,#23346));
#6416=EDGE_LOOP('',(#23347,#23348,#23349,#23350));
#6417=EDGE_LOOP('',(#23351,#23352,#23353,#23354));
#6418=EDGE_LOOP('',(#23355,#23356,#23357,#23358));
#6419=EDGE_LOOP('',(#23359,#23360,#23361,#23362));
#6420=EDGE_LOOP('',(#23363,#23364,#23365,#23366));
#6421=EDGE_LOOP('',(#23367,#23368,#23369,#23370));
#6422=EDGE_LOOP('',(#23371,#23372,#23373,#23374));
#6423=EDGE_LOOP('',(#23375,#23376,#23377,#23378));
#6424=EDGE_LOOP('',(#23379,#23380,#23381,#23382));
#6425=EDGE_LOOP('',(#23383,#23384,#23385,#23386));
#6426=EDGE_LOOP('',(#23387,#23388,#23389,#23390));
#6427=EDGE_LOOP('',(#23391,#23392,#23393,#23394));
#6428=EDGE_LOOP('',(#23395,#23396,#23397,#23398));
#6429=EDGE_LOOP('',(#23399,#23400,#23401,#23402));
#6430=EDGE_LOOP('',(#23403,#23404,#23405,#23406));
#6431=EDGE_LOOP('',(#23407,#23408,#23409,#23410));
#6432=EDGE_LOOP('',(#23411,#23412,#23413,#23414));
#6433=EDGE_LOOP('',(#23415,#23416,#23417,#23418));
#6434=EDGE_LOOP('',(#23419,#23420,#23421,#23422));
#6435=EDGE_LOOP('',(#23423,#23424,#23425,#23426,#23427,#23428,#23429,#23430,
#23431,#23432,#23433,#23434,#23435,#23436,#23437,#23438,#23439,#23440,#23441,
#23442,#23443,#23444,#23445,#23446,#23447,#23448,#23449,#23450,#23451,#23452,
#23453,#23454,#23455,#23456,#23457,#23458,#23459,#23460,#23461,#23462,#23463,
#23464,#23465,#23466,#23467,#23468,#23469,#23470,#23471,#23472,#23473,#23474,
#23475,#23476,#23477,#23478,#23479,#23480,#23481,#23482,#23483,#23484,#23485,
#23486,#23487,#23488,#23489,#23490,#23491,#23492,#23493,#23494,#23495,#23496,
#23497,#23498,#23499,#23500,#23501,#23502,#23503,#23504,#23505,#23506,#23507,
#23508,#23509,#23510));
#6436=EDGE_LOOP('',(#23511,#23512,#23513,#23514,#23515));
#6437=EDGE_LOOP('',(#23516,#23517,#23518,#23519));
#6438=EDGE_LOOP('',(#23520,#23521,#23522,#23523,#23524,#23525,#23526,#23527,
#23528,#23529,#23530,#23531,#23532,#23533,#23534,#23535,#23536,#23537,#23538,
#23539,#23540,#23541,#23542,#23543,#23544,#23545,#23546,#23547,#23548,#23549,
#23550,#23551,#23552,#23553,#23554,#23555,#23556,#23557,#23558,#23559,#23560,
#23561,#23562,#23563,#23564,#23565,#23566,#23567,#23568,#23569,#23570,#23571,
#23572,#23573,#23574,#23575,#23576,#23577,#23578,#23579,#23580,#23581,#23582,
#23583,#23584,#23585,#23586,#23587,#23588,#23589,#23590,#23591,#23592,#23593,
#23594,#23595,#23596,#23597,#23598,#23599,#23600,#23601,#23602,#23603,#23604,
#23605,#23606,#23607));
#6439=EDGE_LOOP('',(#23608,#23609,#23610,#23611,#23612,#23613));
#6440=EDGE_LOOP('',(#23614,#23615,#23616,#23617,#23618));
#6441=EDGE_LOOP('',(#23619));
#6442=EDGE_LOOP('',(#23620));
#6443=EDGE_LOOP('',(#23621,#23622,#23623,#23624));
#6444=EDGE_LOOP('',(#23625,#23626,#23627));
#6445=EDGE_LOOP('',(#23628,#23629,#23630,#23631));
#6446=EDGE_LOOP('',(#23632,#23633,#23634));
#6447=EDGE_LOOP('',(#23635,#23636,#23637,#23638));
#6448=EDGE_LOOP('',(#23639,#23640,#23641));
#6449=EDGE_LOOP('',(#23642,#23643,#23644,#23645));
#6450=EDGE_LOOP('',(#23646,#23647,#23648));
#6451=EDGE_LOOP('',(#23649,#23650,#23651,#23652));
#6452=EDGE_LOOP('',(#23653,#23654,#23655));
#6453=EDGE_LOOP('',(#23656,#23657,#23658,#23659));
#6454=EDGE_LOOP('',(#23660,#23661,#23662));
#6455=EDGE_LOOP('',(#23663,#23664,#23665,#23666));
#6456=EDGE_LOOP('',(#23667,#23668,#23669));
#6457=EDGE_LOOP('',(#23670,#23671,#23672,#23673));
#6458=EDGE_LOOP('',(#23674,#23675,#23676));
#6459=EDGE_LOOP('',(#23677,#23678,#23679,#23680));
#6460=EDGE_LOOP('',(#23681,#23682,#23683));
#6461=EDGE_LOOP('',(#23684,#23685,#23686,#23687));
#6462=EDGE_LOOP('',(#23688,#23689,#23690));
#6463=EDGE_LOOP('',(#23691,#23692,#23693,#23694));
#6464=EDGE_LOOP('',(#23695,#23696,#23697));
#6465=EDGE_LOOP('',(#23698,#23699,#23700,#23701));
#6466=EDGE_LOOP('',(#23702,#23703,#23704));
#6467=EDGE_LOOP('',(#23705,#23706,#23707,#23708));
#6468=EDGE_LOOP('',(#23709,#23710,#23711));
#6469=EDGE_LOOP('',(#23712,#23713,#23714,#23715));
#6470=EDGE_LOOP('',(#23716,#23717,#23718));
#6471=EDGE_LOOP('',(#23719,#23720,#23721,#23722));
#6472=EDGE_LOOP('',(#23723,#23724,#23725));
#6473=EDGE_LOOP('',(#23726,#23727,#23728,#23729));
#6474=EDGE_LOOP('',(#23730,#23731,#23732));
#6475=EDGE_LOOP('',(#23733,#23734,#23735,#23736));
#6476=EDGE_LOOP('',(#23737,#23738,#23739));
#6477=EDGE_LOOP('',(#23740,#23741,#23742,#23743));
#6478=EDGE_LOOP('',(#23744,#23745,#23746));
#6479=EDGE_LOOP('',(#23747,#23748,#23749,#23750));
#6480=EDGE_LOOP('',(#23751,#23752,#23753));
#6481=EDGE_LOOP('',(#23754,#23755,#23756,#23757));
#6482=EDGE_LOOP('',(#23758,#23759,#23760));
#6483=EDGE_LOOP('',(#23761,#23762,#23763,#23764));
#6484=EDGE_LOOP('',(#23765,#23766,#23767));
#6485=EDGE_LOOP('',(#23768,#23769,#23770,#23771));
#6486=EDGE_LOOP('',(#23772,#23773,#23774));
#6487=EDGE_LOOP('',(#23775,#23776,#23777,#23778));
#6488=EDGE_LOOP('',(#23779,#23780,#23781));
#6489=EDGE_LOOP('',(#23782,#23783,#23784,#23785));
#6490=EDGE_LOOP('',(#23786,#23787,#23788));
#6491=EDGE_LOOP('',(#23789,#23790,#23791,#23792));
#6492=EDGE_LOOP('',(#23793,#23794,#23795));
#6493=EDGE_LOOP('',(#23796,#23797,#23798,#23799));
#6494=EDGE_LOOP('',(#23800,#23801,#23802));
#6495=EDGE_LOOP('',(#23803,#23804,#23805,#23806));
#6496=EDGE_LOOP('',(#23807,#23808,#23809));
#6497=EDGE_LOOP('',(#23810,#23811,#23812,#23813));
#6498=EDGE_LOOP('',(#23814,#23815,#23816));
#6499=EDGE_LOOP('',(#23817,#23818,#23819,#23820));
#6500=EDGE_LOOP('',(#23821,#23822,#23823));
#6501=EDGE_LOOP('',(#23824,#23825,#23826,#23827));
#6502=EDGE_LOOP('',(#23828,#23829,#23830));
#6503=EDGE_LOOP('',(#23831,#23832,#23833,#23834));
#6504=EDGE_LOOP('',(#23835,#23836,#23837));
#6505=EDGE_LOOP('',(#23838,#23839,#23840,#23841));
#6506=EDGE_LOOP('',(#23842,#23843,#23844));
#6507=EDGE_LOOP('',(#23845,#23846,#23847,#23848));
#6508=EDGE_LOOP('',(#23849,#23850,#23851));
#6509=EDGE_LOOP('',(#23852,#23853,#23854,#23855));
#6510=EDGE_LOOP('',(#23856,#23857,#23858));
#6511=EDGE_LOOP('',(#23859,#23860,#23861,#23862));
#6512=EDGE_LOOP('',(#23863,#23864,#23865,#23866));
#6513=EDGE_LOOP('',(#23867,#23868,#23869,#23870));
#6514=EDGE_LOOP('',(#23871,#23872,#23873,#23874));
#6515=EDGE_LOOP('',(#23875,#23876,#23877,#23878));
#6516=EDGE_LOOP('',(#23879,#23880,#23881));
#6517=EDGE_LOOP('',(#23882,#23883,#23884,#23885));
#6518=EDGE_LOOP('',(#23886,#23887,#23888));
#6519=EDGE_LOOP('',(#23889,#23890,#23891,#23892));
#6520=EDGE_LOOP('',(#23893,#23894,#23895));
#6521=EDGE_LOOP('',(#23896,#23897,#23898,#23899));
#6522=EDGE_LOOP('',(#23900,#23901,#23902));
#6523=EDGE_LOOP('',(#23903,#23904,#23905,#23906));
#6524=EDGE_LOOP('',(#23907,#23908,#23909));
#6525=EDGE_LOOP('',(#23910,#23911,#23912,#23913));
#6526=EDGE_LOOP('',(#23914,#23915,#23916));
#6527=EDGE_LOOP('',(#23917,#23918,#23919,#23920));
#6528=EDGE_LOOP('',(#23921,#23922,#23923));
#6529=EDGE_LOOP('',(#23924,#23925,#23926,#23927));
#6530=EDGE_LOOP('',(#23928,#23929,#23930));
#6531=EDGE_LOOP('',(#23931,#23932,#23933,#23934));
#6532=EDGE_LOOP('',(#23935,#23936,#23937));
#6533=EDGE_LOOP('',(#23938,#23939,#23940,#23941));
#6534=EDGE_LOOP('',(#23942,#23943,#23944));
#6535=EDGE_LOOP('',(#23945,#23946,#23947,#23948));
#6536=EDGE_LOOP('',(#23949,#23950,#23951));
#6537=EDGE_LOOP('',(#23952,#23953,#23954,#23955));
#6538=EDGE_LOOP('',(#23956,#23957,#23958));
#6539=EDGE_LOOP('',(#23959,#23960,#23961,#23962));
#6540=EDGE_LOOP('',(#23963,#23964,#23965));
#6541=EDGE_LOOP('',(#23966,#23967,#23968,#23969));
#6542=EDGE_LOOP('',(#23970,#23971,#23972));
#6543=EDGE_LOOP('',(#23973,#23974,#23975,#23976));
#6544=EDGE_LOOP('',(#23977,#23978,#23979));
#6545=EDGE_LOOP('',(#23980,#23981,#23982,#23983));
#6546=EDGE_LOOP('',(#23984,#23985,#23986));
#6547=EDGE_LOOP('',(#23987,#23988,#23989,#23990));
#6548=EDGE_LOOP('',(#23991,#23992,#23993));
#6549=EDGE_LOOP('',(#23994,#23995,#23996,#23997));
#6550=EDGE_LOOP('',(#23998,#23999,#24000));
#6551=EDGE_LOOP('',(#24001,#24002,#24003,#24004));
#6552=EDGE_LOOP('',(#24005,#24006,#24007));
#6553=EDGE_LOOP('',(#24008,#24009,#24010,#24011));
#6554=EDGE_LOOP('',(#24012,#24013,#24014));
#6555=EDGE_LOOP('',(#24015,#24016,#24017,#24018));
#6556=EDGE_LOOP('',(#24019,#24020,#24021));
#6557=EDGE_LOOP('',(#24022,#24023,#24024,#24025));
#6558=EDGE_LOOP('',(#24026,#24027,#24028));
#6559=EDGE_LOOP('',(#24029,#24030,#24031,#24032));
#6560=EDGE_LOOP('',(#24033,#24034,#24035));
#6561=EDGE_LOOP('',(#24036,#24037,#24038,#24039));
#6562=EDGE_LOOP('',(#24040,#24041,#24042));
#6563=EDGE_LOOP('',(#24043,#24044,#24045,#24046));
#6564=EDGE_LOOP('',(#24047,#24048,#24049));
#6565=EDGE_LOOP('',(#24050,#24051,#24052,#24053));
#6566=EDGE_LOOP('',(#24054,#24055,#24056));
#6567=EDGE_LOOP('',(#24057,#24058,#24059,#24060));
#6568=EDGE_LOOP('',(#24061,#24062,#24063));
#6569=EDGE_LOOP('',(#24064,#24065,#24066,#24067));
#6570=EDGE_LOOP('',(#24068,#24069,#24070));
#6571=EDGE_LOOP('',(#24071,#24072,#24073,#24074));
#6572=EDGE_LOOP('',(#24075,#24076,#24077));
#6573=EDGE_LOOP('',(#24078,#24079,#24080,#24081));
#6574=EDGE_LOOP('',(#24082,#24083,#24084));
#6575=EDGE_LOOP('',(#24085,#24086,#24087,#24088));
#6576=EDGE_LOOP('',(#24089,#24090,#24091));
#6577=EDGE_LOOP('',(#24092,#24093,#24094,#24095));
#6578=EDGE_LOOP('',(#24096,#24097,#24098));
#6579=EDGE_LOOP('',(#24099,#24100,#24101,#24102));
#6580=EDGE_LOOP('',(#24103,#24104,#24105));
#6581=EDGE_LOOP('',(#24106,#24107,#24108,#24109));
#6582=EDGE_LOOP('',(#24110,#24111,#24112));
#6583=EDGE_LOOP('',(#24113,#24114,#24115,#24116));
#6584=EDGE_LOOP('',(#24117,#24118,#24119));
#6585=EDGE_LOOP('',(#24120,#24121,#24122,#24123));
#6586=EDGE_LOOP('',(#24124,#24125,#24126));
#6587=EDGE_LOOP('',(#24127,#24128,#24129));
#6588=EDGE_LOOP('',(#24130,#24131,#24132,#24133));
#6589=EDGE_LOOP('',(#24134,#24135,#24136,#24137));
#6590=EDGE_LOOP('',(#24138,#24139,#24140,#24141));
#6591=EDGE_LOOP('',(#24142,#24143,#24144,#24145));
#6592=EDGE_LOOP('',(#24146,#24147,#24148,#24149));
#6593=EDGE_LOOP('',(#24150,#24151,#24152,#24153));
#6594=EDGE_LOOP('',(#24154,#24155,#24156,#24157,#24158,#24159));
#6595=EDGE_LOOP('',(#24160));
#6596=EDGE_LOOP('',(#24161));
#6597=EDGE_LOOP('',(#24162,#24163,#24164,#24165,#24166,#24167));
#6598=EDGE_LOOP('',(#24168,#24169,#24170,#24171,#24172,#24173,#24174,#24175,
#24176,#24177,#24178,#24179));
#6599=EDGE_LOOP('',(#24180,#24181,#24182,#24183));
#6600=EDGE_LOOP('',(#24184,#24185,#24186,#24187));
#6601=EDGE_LOOP('',(#24188,#24189,#24190,#24191));
#6602=EDGE_LOOP('',(#24192,#24193,#24194,#24195));
#6603=EDGE_LOOP('',(#24196,#24197,#24198,#24199));
#6604=EDGE_LOOP('',(#24200,#24201,#24202,#24203));
#6605=EDGE_LOOP('',(#24204,#24205,#24206,#24207));
#6606=EDGE_LOOP('',(#24208,#24209,#24210,#24211));
#6607=EDGE_LOOP('',(#24212,#24213,#24214,#24215));
#6608=EDGE_LOOP('',(#24216,#24217,#24218,#24219));
#6609=EDGE_LOOP('',(#24220,#24221,#24222,#24223));
#6610=EDGE_LOOP('',(#24224,#24225,#24226,#24227));
#6611=EDGE_LOOP('',(#24228,#24229,#24230,#24231));
#6612=EDGE_LOOP('',(#24232,#24233,#24234,#24235));
#6613=EDGE_LOOP('',(#24236,#24237,#24238,#24239));
#6614=EDGE_LOOP('',(#24240,#24241,#24242,#24243));
#6615=EDGE_LOOP('',(#24244,#24245,#24246,#24247));
#6616=EDGE_LOOP('',(#24248,#24249,#24250,#24251));
#6617=EDGE_LOOP('',(#24252,#24253,#24254,#24255));
#6618=EDGE_LOOP('',(#24256,#24257,#24258,#24259));
#6619=EDGE_LOOP('',(#24260,#24261,#24262,#24263));
#6620=EDGE_LOOP('',(#24264,#24265,#24266,#24267));
#6621=EDGE_LOOP('',(#24268,#24269,#24270,#24271));
#6622=EDGE_LOOP('',(#24272,#24273,#24274,#24275));
#6623=EDGE_LOOP('',(#24276,#24277,#24278,#24279));
#6624=EDGE_LOOP('',(#24280,#24281,#24282,#24283));
#6625=EDGE_LOOP('',(#24284,#24285,#24286,#24287));
#6626=EDGE_LOOP('',(#24288,#24289,#24290,#24291));
#6627=EDGE_LOOP('',(#24292,#24293,#24294,#24295));
#6628=EDGE_LOOP('',(#24296,#24297,#24298,#24299));
#6629=EDGE_LOOP('',(#24300,#24301,#24302,#24303));
#6630=EDGE_LOOP('',(#24304,#24305,#24306,#24307));
#6631=EDGE_LOOP('',(#24308,#24309,#24310,#24311));
#6632=EDGE_LOOP('',(#24312,#24313,#24314,#24315));
#6633=EDGE_LOOP('',(#24316,#24317,#24318,#24319));
#6634=EDGE_LOOP('',(#24320,#24321,#24322,#24323));
#6635=EDGE_LOOP('',(#24324));
#6636=EDGE_LOOP('',(#24325,#24326,#24327,#24328,#24329,#24330));
#8483=LINE('',#49573,#10789);
#8484=LINE('',#49597,#10790);
#8485=LINE('',#49645,#10791);
#8486=LINE('',#49693,#10792);
#8487=LINE('',#49744,#10793);
#8488=LINE('',#49795,#10794);
#8489=LINE('',#49843,#10795);
#8490=LINE('',#49891,#10796);
#8491=LINE('',#49945,#10797);
#8492=LINE('',#49993,#10798);
#8493=LINE('',#50041,#10799);
#8494=LINE('',#50095,#10800);
#8495=LINE('',#50143,#10801);
#8496=LINE('',#50191,#10802);
#8497=LINE('',#50239,#10803);
#8498=LINE('',#50293,#10804);
#8499=LINE('',#50341,#10805);
#8500=LINE('',#50389,#10806);
#8501=LINE('',#50443,#10807);
#8502=LINE('',#50491,#10808);
#8503=LINE('',#50539,#10809);
#8504=LINE('',#50593,#10810);
#8505=LINE('',#50641,#10811);
#8506=LINE('',#50689,#10812);
#8507=LINE('',#50737,#10813);
#8508=LINE('',#50791,#10814);
#8509=LINE('',#50839,#10815);
#8510=LINE('',#50887,#10816);
#8511=LINE('',#50941,#10817);
#8512=LINE('',#50989,#10818);
#8513=LINE('',#51037,#10819);
#8514=LINE('',#51091,#10820);
#8515=LINE('',#51139,#10821);
#8516=LINE('',#51187,#10822);
#8517=LINE('',#51235,#10823);
#8518=LINE('',#51289,#10824);
#8519=LINE('',#51337,#10825);
#8520=LINE('',#51385,#10826);
#8521=LINE('',#51439,#10827);
#8522=LINE('',#51487,#10828);
#8523=LINE('',#51535,#10829);
#8524=LINE('',#51589,#10830);
#8525=LINE('',#51637,#10831);
#8526=LINE('',#51655,#10832);
#8527=LINE('',#51679,#10833);
#8528=LINE('',#51704,#10834);
#8529=LINE('',#51729,#10835);
#8530=LINE('',#51753,#10836);
#8531=LINE('',#51778,#10837);
#8532=LINE('',#51803,#10838);
#8533=LINE('',#51827,#10839);
#8534=LINE('',#51852,#10840);
#8535=LINE('',#51877,#10841);
#8536=LINE('',#51901,#10842);
#8537=LINE('',#51925,#10843);
#8538=LINE('',#51950,#10844);
#8539=LINE('',#51975,#10845);
#8540=LINE('',#51999,#10846);
#8541=LINE('',#52024,#10847);
#8542=LINE('',#52049,#10848);
#8543=LINE('',#52073,#10849);
#8544=LINE('',#52098,#10850);
#8545=LINE('',#52123,#10851);
#8546=LINE('',#52147,#10852);
#8547=LINE('',#52171,#10853);
#8548=LINE('',#52196,#10854);
#8549=LINE('',#52221,#10855);
#8550=LINE('',#52245,#10856);
#8551=LINE('',#52270,#10857);
#8552=LINE('',#52295,#10858);
#8553=LINE('',#52319,#10859);
#8554=LINE('',#52344,#10860);
#8555=LINE('',#52369,#10861);
#8556=LINE('',#52393,#10862);
#8557=LINE('',#52417,#10863);
#8558=LINE('',#52442,#10864);
#8559=LINE('',#52467,#10865);
#8560=LINE('',#52491,#10866);
#8561=LINE('',#52516,#10867);
#8562=LINE('',#52541,#10868);
#8563=LINE('',#52565,#10869);
#8564=LINE('',#52590,#10870);
#8565=LINE('',#52614,#10871);
#8566=LINE('',#52639,#10872);
#8567=LINE('',#55238,#10873);
#8568=LINE('',#55240,#10874);
#8569=LINE('',#55242,#10875);
#8570=LINE('',#55243,#10876);
#8571=LINE('',#55247,#10877);
#8572=LINE('',#55250,#10878);
#8573=LINE('',#55251,#10879);
#8574=LINE('',#55257,#10880);
#8575=LINE('',#55259,#10881);
#8576=LINE('',#55261,#10882);
#8577=LINE('',#55262,#10883);
#8578=LINE('',#55266,#10884);
#8579=LINE('',#55269,#10885);
#8580=LINE('',#55270,#10886);
#8581=LINE('',#55276,#10887);
#8582=LINE('',#55278,#10888);
#8583=LINE('',#55280,#10889);
#8584=LINE('',#55281,#10890);
#8585=LINE('',#55285,#10891);
#8586=LINE('',#55288,#10892);
#8587=LINE('',#55289,#10893);
#8588=LINE('',#55295,#10894);
#8589=LINE('',#55297,#10895);
#8590=LINE('',#55299,#10896);
#8591=LINE('',#55300,#10897);
#8592=LINE('',#55304,#10898);
#8593=LINE('',#55307,#10899);
#8594=LINE('',#55308,#10900);
#8595=LINE('',#55314,#10901);
#8596=LINE('',#55316,#10902);
#8597=LINE('',#55318,#10903);
#8598=LINE('',#55319,#10904);
#8599=LINE('',#55323,#10905);
#8600=LINE('',#55326,#10906);
#8601=LINE('',#55327,#10907);
#8602=LINE('',#55333,#10908);
#8603=LINE('',#55335,#10909);
#8604=LINE('',#55337,#10910);
#8605=LINE('',#55338,#10911);
#8606=LINE('',#55342,#10912);
#8607=LINE('',#55345,#10913);
#8608=LINE('',#55346,#10914);
#8609=LINE('',#55352,#10915);
#8610=LINE('',#55354,#10916);
#8611=LINE('',#55356,#10917);
#8612=LINE('',#55357,#10918);
#8613=LINE('',#55361,#10919);
#8614=LINE('',#55364,#10920);
#8615=LINE('',#55365,#10921);
#8616=LINE('',#55371,#10922);
#8617=LINE('',#55373,#10923);
#8618=LINE('',#55375,#10924);
#8619=LINE('',#55376,#10925);
#8620=LINE('',#55380,#10926);
#8621=LINE('',#55383,#10927);
#8622=LINE('',#55384,#10928);
#8623=LINE('',#55390,#10929);
#8624=LINE('',#55392,#10930);
#8625=LINE('',#55394,#10931);
#8626=LINE('',#55395,#10932);
#8627=LINE('',#55399,#10933);
#8628=LINE('',#55402,#10934);
#8629=LINE('',#55403,#10935);
#8630=LINE('',#55409,#10936);
#8631=LINE('',#55411,#10937);
#8632=LINE('',#55413,#10938);
#8633=LINE('',#55414,#10939);
#8634=LINE('',#55418,#10940);
#8635=LINE('',#55421,#10941);
#8636=LINE('',#55422,#10942);
#8637=LINE('',#55428,#10943);
#8638=LINE('',#55430,#10944);
#8639=LINE('',#55432,#10945);
#8640=LINE('',#55433,#10946);
#8641=LINE('',#55437,#10947);
#8642=LINE('',#55440,#10948);
#8643=LINE('',#55441,#10949);
#8644=LINE('',#55447,#10950);
#8645=LINE('',#55449,#10951);
#8646=LINE('',#55451,#10952);
#8647=LINE('',#55452,#10953);
#8648=LINE('',#55456,#10954);
#8649=LINE('',#55459,#10955);
#8650=LINE('',#55460,#10956);
#8651=LINE('',#55466,#10957);
#8652=LINE('',#55468,#10958);
#8653=LINE('',#55470,#10959);
#8654=LINE('',#55471,#10960);
#8655=LINE('',#55475,#10961);
#8656=LINE('',#55478,#10962);
#8657=LINE('',#55479,#10963);
#8658=LINE('',#55485,#10964);
#8659=LINE('',#55487,#10965);
#8660=LINE('',#55489,#10966);
#8661=LINE('',#55490,#10967);
#8662=LINE('',#55494,#10968);
#8663=LINE('',#55497,#10969);
#8664=LINE('',#55498,#10970);
#8665=LINE('',#55504,#10971);
#8666=LINE('',#55506,#10972);
#8667=LINE('',#55508,#10973);
#8668=LINE('',#55509,#10974);
#8669=LINE('',#55513,#10975);
#8670=LINE('',#55516,#10976);
#8671=LINE('',#55517,#10977);
#8672=LINE('',#55523,#10978);
#8673=LINE('',#55525,#10979);
#8674=LINE('',#55527,#10980);
#8675=LINE('',#55528,#10981);
#8676=LINE('',#55532,#10982);
#8677=LINE('',#55535,#10983);
#8678=LINE('',#55536,#10984);
#8679=LINE('',#55542,#10985);
#8680=LINE('',#55544,#10986);
#8681=LINE('',#55546,#10987);
#8682=LINE('',#55547,#10988);
#8683=LINE('',#55551,#10989);
#8684=LINE('',#55554,#10990);
#8685=LINE('',#55555,#10991);
#8686=LINE('',#55561,#10992);
#8687=LINE('',#55563,#10993);
#8688=LINE('',#55565,#10994);
#8689=LINE('',#55566,#10995);
#8690=LINE('',#55571,#10996);
#8691=LINE('',#55575,#10997);
#8692=LINE('',#55576,#10998);
#8693=LINE('',#55584,#10999);
#8694=LINE('',#55586,#11000);
#8695=LINE('',#55588,#11001);
#8696=LINE('',#55589,#11002);
#8697=LINE('',#55593,#11003);
#8698=LINE('',#55596,#11004);
#8699=LINE('',#55597,#11005);
#8700=LINE('',#55603,#11006);
#8701=LINE('',#55605,#11007);
#8702=LINE('',#55607,#11008);
#8703=LINE('',#55608,#11009);
#8704=LINE('',#55612,#11010);
#8705=LINE('',#55615,#11011);
#8706=LINE('',#55616,#11012);
#8707=LINE('',#55622,#11013);
#8708=LINE('',#55624,#11014);
#8709=LINE('',#55626,#11015);
#8710=LINE('',#55627,#11016);
#8711=LINE('',#55631,#11017);
#8712=LINE('',#55634,#11018);
#8713=LINE('',#55635,#11019);
#8714=LINE('',#55641,#11020);
#8715=LINE('',#55643,#11021);
#8716=LINE('',#55645,#11022);
#8717=LINE('',#55646,#11023);
#8718=LINE('',#55650,#11024);
#8719=LINE('',#55653,#11025);
#8720=LINE('',#55654,#11026);
#8721=LINE('',#55660,#11027);
#8722=LINE('',#55662,#11028);
#8723=LINE('',#55664,#11029);
#8724=LINE('',#55665,#11030);
#8725=LINE('',#55669,#11031);
#8726=LINE('',#55672,#11032);
#8727=LINE('',#55673,#11033);
#8728=LINE('',#55679,#11034);
#8729=LINE('',#55681,#11035);
#8730=LINE('',#55683,#11036);
#8731=LINE('',#55684,#11037);
#8732=LINE('',#55688,#11038);
#8733=LINE('',#55691,#11039);
#8734=LINE('',#55692,#11040);
#8735=LINE('',#55698,#11041);
#8736=LINE('',#55700,#11042);
#8737=LINE('',#55702,#11043);
#8738=LINE('',#55703,#11044);
#8739=LINE('',#55707,#11045);
#8740=LINE('',#55710,#11046);
#8741=LINE('',#55711,#11047);
#8742=LINE('',#55717,#11048);
#8743=LINE('',#55719,#11049);
#8744=LINE('',#55721,#11050);
#8745=LINE('',#55722,#11051);
#8746=LINE('',#55726,#11052);
#8747=LINE('',#55729,#11053);
#8748=LINE('',#55730,#11054);
#8749=LINE('',#55736,#11055);
#8750=LINE('',#55738,#11056);
#8751=LINE('',#55740,#11057);
#8752=LINE('',#55741,#11058);
#8753=LINE('',#55745,#11059);
#8754=LINE('',#55748,#11060);
#8755=LINE('',#55749,#11061);
#8756=LINE('',#55755,#11062);
#8757=LINE('',#55757,#11063);
#8758=LINE('',#55759,#11064);
#8759=LINE('',#55760,#11065);
#8760=LINE('',#55764,#11066);
#8761=LINE('',#55767,#11067);
#8762=LINE('',#55768,#11068);
#8763=LINE('',#55774,#11069);
#8764=LINE('',#55776,#11070);
#8765=LINE('',#55778,#11071);
#8766=LINE('',#55779,#11072);
#8767=LINE('',#55783,#11073);
#8768=LINE('',#55786,#11074);
#8769=LINE('',#55787,#11075);
#8770=LINE('',#55793,#11076);
#8771=LINE('',#55795,#11077);
#8772=LINE('',#55797,#11078);
#8773=LINE('',#55798,#11079);
#8774=LINE('',#55802,#11080);
#8775=LINE('',#55805,#11081);
#8776=LINE('',#55806,#11082);
#8777=LINE('',#55812,#11083);
#8778=LINE('',#55814,#11084);
#8779=LINE('',#55816,#11085);
#8780=LINE('',#55817,#11086);
#8781=LINE('',#55821,#11087);
#8782=LINE('',#55824,#11088);
#8783=LINE('',#55825,#11089);
#8784=LINE('',#55831,#11090);
#8785=LINE('',#55833,#11091);
#8786=LINE('',#55835,#11092);
#8787=LINE('',#55836,#11093);
#8788=LINE('',#55840,#11094);
#8789=LINE('',#55843,#11095);
#8790=LINE('',#55844,#11096);
#8791=LINE('',#55850,#11097);
#8792=LINE('',#55852,#11098);
#8793=LINE('',#55854,#11099);
#8794=LINE('',#55855,#11100);
#8795=LINE('',#55859,#11101);
#8796=LINE('',#55862,#11102);
#8797=LINE('',#55863,#11103);
#8798=LINE('',#55869,#11104);
#8799=LINE('',#55871,#11105);
#8800=LINE('',#55873,#11106);
#8801=LINE('',#55874,#11107);
#8802=LINE('',#55878,#11108);
#8803=LINE('',#55881,#11109);
#8804=LINE('',#55882,#11110);
#8805=LINE('',#55888,#11111);
#8806=LINE('',#55890,#11112);
#8807=LINE('',#55892,#11113);
#8808=LINE('',#55893,#11114);
#8809=LINE('',#55897,#11115);
#8810=LINE('',#55900,#11116);
#8811=LINE('',#55901,#11117);
#8812=LINE('',#55907,#11118);
#8813=LINE('',#55909,#11119);
#8814=LINE('',#55911,#11120);
#8815=LINE('',#55912,#11121);
#8816=LINE('',#55916,#11122);
#8817=LINE('',#55919,#11123);
#8818=LINE('',#55920,#11124);
#8819=LINE('',#55926,#11125);
#8820=LINE('',#55931,#11126);
#8821=LINE('',#55933,#11127);
#8822=LINE('',#55935,#11128);
#8823=LINE('',#55936,#11129);
#8824=LINE('',#55939,#11130);
#8825=LINE('',#55941,#11131);
#8826=LINE('',#55942,#11132);
#8827=LINE('',#55945,#11133);
#8828=LINE('',#55947,#11134);
#8829=LINE('',#55948,#11135);
#8830=LINE('',#55951,#11136);
#8831=LINE('',#55953,#11137);
#8832=LINE('',#55954,#11138);
#8833=LINE('',#55957,#11139);
#8834=LINE('',#55959,#11140);
#8835=LINE('',#55960,#11141);
#8836=LINE('',#55962,#11142);
#8837=LINE('',#55963,#11143);
#8838=LINE('',#55969,#11144);
#8839=LINE('',#55973,#11145);
#8840=LINE('',#55974,#11146);
#8841=LINE('',#55978,#11147);
#10789=VECTOR('',#36952,2.);
#10790=VECTOR('',#36957,2.);
#10791=VECTOR('',#36960,2.);
#10792=VECTOR('',#36963,2.);
#10793=VECTOR('',#36966,2.);
#10794=VECTOR('',#36969,2.);
#10795=VECTOR('',#36972,2.);
#10796=VECTOR('',#36975,2.);
#10797=VECTOR('',#36978,2.);
#10798=VECTOR('',#36981,2.);
#10799=VECTOR('',#36984,2.);
#10800=VECTOR('',#36987,2.);
#10801=VECTOR('',#36990,2.);
#10802=VECTOR('',#36993,2.);
#10803=VECTOR('',#36996,2.);
#10804=VECTOR('',#36999,2.);
#10805=VECTOR('',#37002,2.);
#10806=VECTOR('',#37005,2.);
#10807=VECTOR('',#37008,2.);
#10808=VECTOR('',#37011,2.);
#10809=VECTOR('',#37014,2.);
#10810=VECTOR('',#37017,2.);
#10811=VECTOR('',#37020,2.);
#10812=VECTOR('',#37023,2.);
#10813=VECTOR('',#37026,2.);
#10814=VECTOR('',#37029,2.);
#10815=VECTOR('',#37032,2.);
#10816=VECTOR('',#37035,2.);
#10817=VECTOR('',#37038,2.);
#10818=VECTOR('',#37041,2.);
#10819=VECTOR('',#37044,2.);
#10820=VECTOR('',#37047,2.);
#10821=VECTOR('',#37050,2.);
#10822=VECTOR('',#37053,2.);
#10823=VECTOR('',#37056,2.);
#10824=VECTOR('',#37059,2.);
#10825=VECTOR('',#37062,2.);
#10826=VECTOR('',#37065,2.);
#10827=VECTOR('',#37068,2.);
#10828=VECTOR('',#37071,2.);
#10829=VECTOR('',#37074,2.);
#10830=VECTOR('',#37077,2.);
#10831=VECTOR('',#37080,1.5555);
#10832=VECTOR('',#37085,1.5555);
#10833=VECTOR('',#37088,1.5555);
#10834=VECTOR('',#37091,1.5555);
#10835=VECTOR('',#37094,1.5555);
#10836=VECTOR('',#37097,1.5555);
#10837=VECTOR('',#37100,1.5555);
#10838=VECTOR('',#37103,1.5555);
#10839=VECTOR('',#37106,1.5555);
#10840=VECTOR('',#37109,1.5555);
#10841=VECTOR('',#37112,1.5555);
#10842=VECTOR('',#37115,1.5555);
#10843=VECTOR('',#37118,1.5555);
#10844=VECTOR('',#37121,1.5555);
#10845=VECTOR('',#37124,1.5555);
#10846=VECTOR('',#37127,1.5555);
#10847=VECTOR('',#37130,1.5555);
#10848=VECTOR('',#37133,1.5555);
#10849=VECTOR('',#37136,1.5555);
#10850=VECTOR('',#37139,1.5555);
#10851=VECTOR('',#37142,1.5555);
#10852=VECTOR('',#37145,1.5555);
#10853=VECTOR('',#37148,1.5555);
#10854=VECTOR('',#37151,1.5555);
#10855=VECTOR('',#37154,1.5555);
#10856=VECTOR('',#37157,1.5555);
#10857=VECTOR('',#37160,1.5555);
#10858=VECTOR('',#37163,1.5555);
#10859=VECTOR('',#37166,1.5555);
#10860=VECTOR('',#37169,1.5555);
#10861=VECTOR('',#37172,1.5555);
#10862=VECTOR('',#37175,1.5555);
#10863=VECTOR('',#37178,1.5555);
#10864=VECTOR('',#37181,1.5555);
#10865=VECTOR('',#37184,1.5555);
#10866=VECTOR('',#37187,1.5555);
#10867=VECTOR('',#37190,1.5555);
#10868=VECTOR('',#37193,1.5555);
#10869=VECTOR('',#37196,1.5555);
#10870=VECTOR('',#37199,1.5555);
#10871=VECTOR('',#37202,1.5555);
#10872=VECTOR('',#37205,1.5555);
#10873=VECTOR('',#37238,10.);
#10874=VECTOR('',#37239,10.);
#10875=VECTOR('',#37240,10.);
#10876=VECTOR('',#37241,10.);
#10877=VECTOR('',#37246,10.);
#10878=VECTOR('',#37249,10.);
#10879=VECTOR('',#37250,10.);
#10880=VECTOR('',#37257,10.);
#10881=VECTOR('',#37258,10.);
#10882=VECTOR('',#37259,10.);
#10883=VECTOR('',#37260,10.);
#10884=VECTOR('',#37265,10.);
#10885=VECTOR('',#37268,10.);
#10886=VECTOR('',#37269,10.);
#10887=VECTOR('',#37276,10.);
#10888=VECTOR('',#37277,10.);
#10889=VECTOR('',#37278,10.);
#10890=VECTOR('',#37279,10.);
#10891=VECTOR('',#37284,10.);
#10892=VECTOR('',#37287,10.);
#10893=VECTOR('',#37288,10.);
#10894=VECTOR('',#37295,10.);
#10895=VECTOR('',#37296,10.);
#10896=VECTOR('',#37297,10.);
#10897=VECTOR('',#37298,10.);
#10898=VECTOR('',#37303,10.);
#10899=VECTOR('',#37306,10.);
#10900=VECTOR('',#37307,10.);
#10901=VECTOR('',#37314,10.);
#10902=VECTOR('',#37315,10.);
#10903=VECTOR('',#37316,10.);
#10904=VECTOR('',#37317,10.);
#10905=VECTOR('',#37322,10.);
#10906=VECTOR('',#37325,10.);
#10907=VECTOR('',#37326,10.);
#10908=VECTOR('',#37333,10.);
#10909=VECTOR('',#37334,10.);
#10910=VECTOR('',#37335,10.);
#10911=VECTOR('',#37336,10.);
#10912=VECTOR('',#37341,10.);
#10913=VECTOR('',#37344,10.);
#10914=VECTOR('',#37345,10.);
#10915=VECTOR('',#37352,10.);
#10916=VECTOR('',#37353,10.);
#10917=VECTOR('',#37354,10.);
#10918=VECTOR('',#37355,10.);
#10919=VECTOR('',#37360,10.);
#10920=VECTOR('',#37363,10.);
#10921=VECTOR('',#37364,10.);
#10922=VECTOR('',#37371,10.);
#10923=VECTOR('',#37372,10.);
#10924=VECTOR('',#37373,10.);
#10925=VECTOR('',#37374,10.);
#10926=VECTOR('',#37379,10.);
#10927=VECTOR('',#37382,10.);
#10928=VECTOR('',#37383,10.);
#10929=VECTOR('',#37390,10.);
#10930=VECTOR('',#37391,10.);
#10931=VECTOR('',#37392,10.);
#10932=VECTOR('',#37393,10.);
#10933=VECTOR('',#37398,10.);
#10934=VECTOR('',#37401,10.);
#10935=VECTOR('',#37402,10.);
#10936=VECTOR('',#37409,10.);
#10937=VECTOR('',#37410,10.);
#10938=VECTOR('',#37411,10.);
#10939=VECTOR('',#37412,10.);
#10940=VECTOR('',#37417,10.);
#10941=VECTOR('',#37420,10.);
#10942=VECTOR('',#37421,10.);
#10943=VECTOR('',#37428,10.);
#10944=VECTOR('',#37429,10.);
#10945=VECTOR('',#37430,10.);
#10946=VECTOR('',#37431,10.);
#10947=VECTOR('',#37436,10.);
#10948=VECTOR('',#37439,10.);
#10949=VECTOR('',#37440,10.);
#10950=VECTOR('',#37447,10.);
#10951=VECTOR('',#37448,10.);
#10952=VECTOR('',#37449,10.);
#10953=VECTOR('',#37450,10.);
#10954=VECTOR('',#37455,10.);
#10955=VECTOR('',#37458,10.);
#10956=VECTOR('',#37459,10.);
#10957=VECTOR('',#37466,10.);
#10958=VECTOR('',#37467,10.);
#10959=VECTOR('',#37468,10.);
#10960=VECTOR('',#37469,10.);
#10961=VECTOR('',#37474,10.);
#10962=VECTOR('',#37477,10.);
#10963=VECTOR('',#37478,10.);
#10964=VECTOR('',#37485,10.);
#10965=VECTOR('',#37486,10.);
#10966=VECTOR('',#37487,10.);
#10967=VECTOR('',#37488,10.);
#10968=VECTOR('',#37493,10.);
#10969=VECTOR('',#37496,10.);
#10970=VECTOR('',#37497,10.);
#10971=VECTOR('',#37504,10.);
#10972=VECTOR('',#37505,10.);
#10973=VECTOR('',#37506,10.);
#10974=VECTOR('',#37507,10.);
#10975=VECTOR('',#37512,10.);
#10976=VECTOR('',#37515,10.);
#10977=VECTOR('',#37516,10.);
#10978=VECTOR('',#37523,10.);
#10979=VECTOR('',#37524,10.);
#10980=VECTOR('',#37525,10.);
#10981=VECTOR('',#37526,10.);
#10982=VECTOR('',#37531,10.);
#10983=VECTOR('',#37534,10.);
#10984=VECTOR('',#37535,10.);
#10985=VECTOR('',#37542,10.);
#10986=VECTOR('',#37543,10.);
#10987=VECTOR('',#37544,10.);
#10988=VECTOR('',#37545,10.);
#10989=VECTOR('',#37550,10.);
#10990=VECTOR('',#37553,10.);
#10991=VECTOR('',#37554,10.);
#10992=VECTOR('',#37561,10.);
#10993=VECTOR('',#37562,10.);
#10994=VECTOR('',#37563,10.);
#10995=VECTOR('',#37564,10.);
#10996=VECTOR('',#37569,10.);
#10997=VECTOR('',#37574,10.);
#10998=VECTOR('',#37575,10.);
#10999=VECTOR('',#37584,10.);
#11000=VECTOR('',#37585,10.);
#11001=VECTOR('',#37586,10.);
#11002=VECTOR('',#37587,10.);
#11003=VECTOR('',#37592,10.);
#11004=VECTOR('',#37595,10.);
#11005=VECTOR('',#37596,10.);
#11006=VECTOR('',#37603,10.);
#11007=VECTOR('',#37604,10.);
#11008=VECTOR('',#37605,10.);
#11009=VECTOR('',#37606,10.);
#11010=VECTOR('',#37611,10.);
#11011=VECTOR('',#37614,10.);
#11012=VECTOR('',#37615,10.);
#11013=VECTOR('',#37622,10.);
#11014=VECTOR('',#37623,10.);
#11015=VECTOR('',#37624,10.);
#11016=VECTOR('',#37625,10.);
#11017=VECTOR('',#37630,10.);
#11018=VECTOR('',#37633,10.);
#11019=VECTOR('',#37634,10.);
#11020=VECTOR('',#37641,10.);
#11021=VECTOR('',#37642,10.);
#11022=VECTOR('',#37643,10.);
#11023=VECTOR('',#37644,10.);
#11024=VECTOR('',#37649,10.);
#11025=VECTOR('',#37652,10.);
#11026=VECTOR('',#37653,10.);
#11027=VECTOR('',#37660,10.);
#11028=VECTOR('',#37661,10.);
#11029=VECTOR('',#37662,10.);
#11030=VECTOR('',#37663,10.);
#11031=VECTOR('',#37668,10.);
#11032=VECTOR('',#37671,10.);
#11033=VECTOR('',#37672,10.);
#11034=VECTOR('',#37679,10.);
#11035=VECTOR('',#37680,10.);
#11036=VECTOR('',#37681,10.);
#11037=VECTOR('',#37682,10.);
#11038=VECTOR('',#37687,10.);
#11039=VECTOR('',#37690,10.);
#11040=VECTOR('',#37691,10.);
#11041=VECTOR('',#37698,10.);
#11042=VECTOR('',#37699,10.);
#11043=VECTOR('',#37700,10.);
#11044=VECTOR('',#37701,10.);
#11045=VECTOR('',#37706,10.);
#11046=VECTOR('',#37709,10.);
#11047=VECTOR('',#37710,10.);
#11048=VECTOR('',#37717,10.);
#11049=VECTOR('',#37718,10.);
#11050=VECTOR('',#37719,10.);
#11051=VECTOR('',#37720,10.);
#11052=VECTOR('',#37725,10.);
#11053=VECTOR('',#37728,10.);
#11054=VECTOR('',#37729,10.);
#11055=VECTOR('',#37736,10.);
#11056=VECTOR('',#37737,10.);
#11057=VECTOR('',#37738,10.);
#11058=VECTOR('',#37739,10.);
#11059=VECTOR('',#37744,10.);
#11060=VECTOR('',#37747,10.);
#11061=VECTOR('',#37748,10.);
#11062=VECTOR('',#37755,10.);
#11063=VECTOR('',#37756,10.);
#11064=VECTOR('',#37757,10.);
#11065=VECTOR('',#37758,10.);
#11066=VECTOR('',#37763,10.);
#11067=VECTOR('',#37766,10.);
#11068=VECTOR('',#37767,10.);
#11069=VECTOR('',#37774,10.);
#11070=VECTOR('',#37775,10.);
#11071=VECTOR('',#37776,10.);
#11072=VECTOR('',#37777,10.);
#11073=VECTOR('',#37782,10.);
#11074=VECTOR('',#37785,10.);
#11075=VECTOR('',#37786,10.);
#11076=VECTOR('',#37793,10.);
#11077=VECTOR('',#37794,10.);
#11078=VECTOR('',#37795,10.);
#11079=VECTOR('',#37796,10.);
#11080=VECTOR('',#37801,10.);
#11081=VECTOR('',#37804,10.);
#11082=VECTOR('',#37805,10.);
#11083=VECTOR('',#37812,10.);
#11084=VECTOR('',#37813,10.);
#11085=VECTOR('',#37814,10.);
#11086=VECTOR('',#37815,10.);
#11087=VECTOR('',#37820,10.);
#11088=VECTOR('',#37823,10.);
#11089=VECTOR('',#37824,10.);
#11090=VECTOR('',#37831,10.);
#11091=VECTOR('',#37832,10.);
#11092=VECTOR('',#37833,10.);
#11093=VECTOR('',#37834,10.);
#11094=VECTOR('',#37839,10.);
#11095=VECTOR('',#37842,10.);
#11096=VECTOR('',#37843,10.);
#11097=VECTOR('',#37850,10.);
#11098=VECTOR('',#37851,10.);
#11099=VECTOR('',#37852,10.);
#11100=VECTOR('',#37853,10.);
#11101=VECTOR('',#37858,10.);
#11102=VECTOR('',#37861,10.);
#11103=VECTOR('',#37862,10.);
#11104=VECTOR('',#37869,10.);
#11105=VECTOR('',#37870,10.);
#11106=VECTOR('',#37871,10.);
#11107=VECTOR('',#37872,10.);
#11108=VECTOR('',#37877,10.);
#11109=VECTOR('',#37880,10.);
#11110=VECTOR('',#37881,10.);
#11111=VECTOR('',#37888,10.);
#11112=VECTOR('',#37889,10.);
#11113=VECTOR('',#37890,10.);
#11114=VECTOR('',#37891,10.);
#11115=VECTOR('',#37896,10.);
#11116=VECTOR('',#37899,10.);
#11117=VECTOR('',#37900,10.);
#11118=VECTOR('',#37907,10.);
#11119=VECTOR('',#37908,10.);
#11120=VECTOR('',#37909,10.);
#11121=VECTOR('',#37910,10.);
#11122=VECTOR('',#37915,10.);
#11123=VECTOR('',#37918,10.);
#11124=VECTOR('',#37919,10.);
#11125=VECTOR('',#37926,0.75);
#11126=VECTOR('',#37931,10.);
#11127=VECTOR('',#37932,10.);
#11128=VECTOR('',#37933,10.);
#11129=VECTOR('',#37934,10.);
#11130=VECTOR('',#37937,10.);
#11131=VECTOR('',#37938,10.);
#11132=VECTOR('',#37939,10.);
#11133=VECTOR('',#37942,10.);
#11134=VECTOR('',#37943,10.);
#11135=VECTOR('',#37944,10.);
#11136=VECTOR('',#37947,10.);
#11137=VECTOR('',#37948,10.);
#11138=VECTOR('',#37949,10.);
#11139=VECTOR('',#37952,10.);
#11140=VECTOR('',#37953,10.);
#11141=VECTOR('',#37954,10.);
#11142=VECTOR('',#37957,10.);
#11143=VECTOR('',#37958,10.);
#11144=VECTOR('',#37967,1.8);
#11145=VECTOR('',#37972,3.5);
#11146=VECTOR('',#37973,3.5);
#11147=VECTOR('',#37978,3.3);
#13194=VERTEX_POINT('',#49571);
#13195=VERTEX_POINT('',#49572);
#13196=VERTEX_POINT('',#49574);
#13197=VERTEX_POINT('',#49585);
#13198=VERTEX_POINT('',#49595);
#13199=VERTEX_POINT('',#49596);
#13200=VERTEX_POINT('',#49643);
#13201=VERTEX_POINT('',#49644);
#13202=VERTEX_POINT('',#49691);
#13203=VERTEX_POINT('',#49692);
#13204=VERTEX_POINT('',#49742);
#13205=VERTEX_POINT('',#49743);
#13206=VERTEX_POINT('',#49793);
#13207=VERTEX_POINT('',#49794);
#13208=VERTEX_POINT('',#49841);
#13209=VERTEX_POINT('',#49842);
#13210=VERTEX_POINT('',#49889);
#13211=VERTEX_POINT('',#49890);
#13212=VERTEX_POINT('',#49943);
#13213=VERTEX_POINT('',#49944);
#13214=VERTEX_POINT('',#49991);
#13215=VERTEX_POINT('',#49992);
#13216=VERTEX_POINT('',#50039);
#13217=VERTEX_POINT('',#50040);
#13218=VERTEX_POINT('',#50093);
#13219=VERTEX_POINT('',#50094);
#13220=VERTEX_POINT('',#50141);
#13221=VERTEX_POINT('',#50142);
#13222=VERTEX_POINT('',#50189);
#13223=VERTEX_POINT('',#50190);
#13224=VERTEX_POINT('',#50237);
#13225=VERTEX_POINT('',#50238);
#13226=VERTEX_POINT('',#50291);
#13227=VERTEX_POINT('',#50292);
#13228=VERTEX_POINT('',#50339);
#13229=VERTEX_POINT('',#50340);
#13230=VERTEX_POINT('',#50387);
#13231=VERTEX_POINT('',#50388);
#13232=VERTEX_POINT('',#50441);
#13233=VERTEX_POINT('',#50442);
#13234=VERTEX_POINT('',#50489);
#13235=VERTEX_POINT('',#50490);
#13236=VERTEX_POINT('',#50537);
#13237=VERTEX_POINT('',#50538);
#13238=VERTEX_POINT('',#50591);
#13239=VERTEX_POINT('',#50592);
#13240=VERTEX_POINT('',#50639);
#13241=VERTEX_POINT('',#50640);
#13242=VERTEX_POINT('',#50687);
#13243=VERTEX_POINT('',#50688);
#13244=VERTEX_POINT('',#50735);
#13245=VERTEX_POINT('',#50736);
#13246=VERTEX_POINT('',#50789);
#13247=VERTEX_POINT('',#50790);
#13248=VERTEX_POINT('',#50837);
#13249=VERTEX_POINT('',#50838);
#13250=VERTEX_POINT('',#50885);
#13251=VERTEX_POINT('',#50886);
#13252=VERTEX_POINT('',#50939);
#13253=VERTEX_POINT('',#50940);
#13254=VERTEX_POINT('',#50987);
#13255=VERTEX_POINT('',#50988);
#13256=VERTEX_POINT('',#51035);
#13257=VERTEX_POINT('',#51036);
#13258=VERTEX_POINT('',#51089);
#13259=VERTEX_POINT('',#51090);
#13260=VERTEX_POINT('',#51137);
#13261=VERTEX_POINT('',#51138);
#13262=VERTEX_POINT('',#51185);
#13263=VERTEX_POINT('',#51186);
#13264=VERTEX_POINT('',#51233);
#13265=VERTEX_POINT('',#51234);
#13266=VERTEX_POINT('',#51287);
#13267=VERTEX_POINT('',#51288);
#13268=VERTEX_POINT('',#51335);
#13269=VERTEX_POINT('',#51336);
#13270=VERTEX_POINT('',#51383);
#13271=VERTEX_POINT('',#51384);
#13272=VERTEX_POINT('',#51437);
#13273=VERTEX_POINT('',#51438);
#13274=VERTEX_POINT('',#51485);
#13275=VERTEX_POINT('',#51486);
#13276=VERTEX_POINT('',#51533);
#13277=VERTEX_POINT('',#51534);
#13278=VERTEX_POINT('',#51587);
#13279=VERTEX_POINT('',#51588);
#13280=VERTEX_POINT('',#51635);
#13281=VERTEX_POINT('',#51636);
#13282=VERTEX_POINT('',#51638);
#13283=VERTEX_POINT('',#51645);
#13284=VERTEX_POINT('',#51653);
#13285=VERTEX_POINT('',#51654);
#13286=VERTEX_POINT('',#51677);
#13287=VERTEX_POINT('',#51678);
#13288=VERTEX_POINT('',#51702);
#13289=VERTEX_POINT('',#51703);
#13290=VERTEX_POINT('',#51727);
#13291=VERTEX_POINT('',#51728);
#13292=VERTEX_POINT('',#51751);
#13293=VERTEX_POINT('',#51752);
#13294=VERTEX_POINT('',#51776);
#13295=VERTEX_POINT('',#51777);
#13296=VERTEX_POINT('',#51801);
#13297=VERTEX_POINT('',#51802);
#13298=VERTEX_POINT('',#51825);
#13299=VERTEX_POINT('',#51826);
#13300=VERTEX_POINT('',#51850);
#13301=VERTEX_POINT('',#51851);
#13302=VERTEX_POINT('',#51875);
#13303=VERTEX_POINT('',#51876);
#13304=VERTEX_POINT('',#51899);
#13305=VERTEX_POINT('',#51900);
#13306=VERTEX_POINT('',#51923);
#13307=VERTEX_POINT('',#51924);
#13308=VERTEX_POINT('',#51948);
#13309=VERTEX_POINT('',#51949);
#13310=VERTEX_POINT('',#51973);
#13311=VERTEX_POINT('',#51974);
#13312=VERTEX_POINT('',#51997);
#13313=VERTEX_POINT('',#51998);
#13314=VERTEX_POINT('',#52022);
#13315=VERTEX_POINT('',#52023);
#13316=VERTEX_POINT('',#52047);
#13317=VERTEX_POINT('',#52048);
#13318=VERTEX_POINT('',#52071);
#13319=VERTEX_POINT('',#52072);
#13320=VERTEX_POINT('',#52096);
#13321=VERTEX_POINT('',#52097);
#13322=VERTEX_POINT('',#52121);
#13323=VERTEX_POINT('',#52122);
#13324=VERTEX_POINT('',#52145);
#13325=VERTEX_POINT('',#52146);
#13326=VERTEX_POINT('',#52169);
#13327=VERTEX_POINT('',#52170);
#13328=VERTEX_POINT('',#52194);
#13329=VERTEX_POINT('',#52195);
#13330=VERTEX_POINT('',#52219);
#13331=VERTEX_POINT('',#52220);
#13332=VERTEX_POINT('',#52243);
#13333=VERTEX_POINT('',#52244);
#13334=VERTEX_POINT('',#52268);
#13335=VERTEX_POINT('',#52269);
#13336=VERTEX_POINT('',#52293);
#13337=VERTEX_POINT('',#52294);
#13338=VERTEX_POINT('',#52317);
#13339=VERTEX_POINT('',#52318);
#13340=VERTEX_POINT('',#52342);
#13341=VERTEX_POINT('',#52343);
#13342=VERTEX_POINT('',#52367);
#13343=VERTEX_POINT('',#52368);
#13344=VERTEX_POINT('',#52391);
#13345=VERTEX_POINT('',#52392);
#13346=VERTEX_POINT('',#52415);
#13347=VERTEX_POINT('',#52416);
#13348=VERTEX_POINT('',#52440);
#13349=VERTEX_POINT('',#52441);
#13350=VERTEX_POINT('',#52465);
#13351=VERTEX_POINT('',#52466);
#13352=VERTEX_POINT('',#52489);
#13353=VERTEX_POINT('',#52490);
#13354=VERTEX_POINT('',#52514);
#13355=VERTEX_POINT('',#52515);
#13356=VERTEX_POINT('',#52539);
#13357=VERTEX_POINT('',#52540);
#13358=VERTEX_POINT('',#52563);
#13359=VERTEX_POINT('',#52564);
#13360=VERTEX_POINT('',#52588);
#13361=VERTEX_POINT('',#52589);
#13362=VERTEX_POINT('',#52612);
#13363=VERTEX_POINT('',#52613);
#13364=VERTEX_POINT('',#52637);
#13365=VERTEX_POINT('',#52638);
#13366=VERTEX_POINT('',#52661);
#13367=VERTEX_POINT('',#52747);
#13368=VERTEX_POINT('',#53933);
#13369=VERTEX_POINT('',#54029);
#13370=VERTEX_POINT('',#54032);
#13371=VERTEX_POINT('',#55225);
#13372=VERTEX_POINT('',#55227);
#13373=VERTEX_POINT('',#55233);
#13374=VERTEX_POINT('',#55236);
#13375=VERTEX_POINT('',#55237);
#13376=VERTEX_POINT('',#55239);
#13377=VERTEX_POINT('',#55241);
#13378=VERTEX_POINT('',#55245);
#13379=VERTEX_POINT('',#55249);
#13380=VERTEX_POINT('',#55255);
#13381=VERTEX_POINT('',#55256);
#13382=VERTEX_POINT('',#55258);
#13383=VERTEX_POINT('',#55260);
#13384=VERTEX_POINT('',#55264);
#13385=VERTEX_POINT('',#55268);
#13386=VERTEX_POINT('',#55274);
#13387=VERTEX_POINT('',#55275);
#13388=VERTEX_POINT('',#55277);
#13389=VERTEX_POINT('',#55279);
#13390=VERTEX_POINT('',#55283);
#13391=VERTEX_POINT('',#55287);
#13392=VERTEX_POINT('',#55293);
#13393=VERTEX_POINT('',#55294);
#13394=VERTEX_POINT('',#55296);
#13395=VERTEX_POINT('',#55298);
#13396=VERTEX_POINT('',#55302);
#13397=VERTEX_POINT('',#55306);
#13398=VERTEX_POINT('',#55312);
#13399=VERTEX_POINT('',#55313);
#13400=VERTEX_POINT('',#55315);
#13401=VERTEX_POINT('',#55317);
#13402=VERTEX_POINT('',#55321);
#13403=VERTEX_POINT('',#55325);
#13404=VERTEX_POINT('',#55331);
#13405=VERTEX_POINT('',#55332);
#13406=VERTEX_POINT('',#55334);
#13407=VERTEX_POINT('',#55336);
#13408=VERTEX_POINT('',#55340);
#13409=VERTEX_POINT('',#55344);
#13410=VERTEX_POINT('',#55350);
#13411=VERTEX_POINT('',#55351);
#13412=VERTEX_POINT('',#55353);
#13413=VERTEX_POINT('',#55355);
#13414=VERTEX_POINT('',#55359);
#13415=VERTEX_POINT('',#55363);
#13416=VERTEX_POINT('',#55369);
#13417=VERTEX_POINT('',#55370);
#13418=VERTEX_POINT('',#55372);
#13419=VERTEX_POINT('',#55374);
#13420=VERTEX_POINT('',#55378);
#13421=VERTEX_POINT('',#55382);
#13422=VERTEX_POINT('',#55388);
#13423=VERTEX_POINT('',#55389);
#13424=VERTEX_POINT('',#55391);
#13425=VERTEX_POINT('',#55393);
#13426=VERTEX_POINT('',#55397);
#13427=VERTEX_POINT('',#55401);
#13428=VERTEX_POINT('',#55407);
#13429=VERTEX_POINT('',#55408);
#13430=VERTEX_POINT('',#55410);
#13431=VERTEX_POINT('',#55412);
#13432=VERTEX_POINT('',#55416);
#13433=VERTEX_POINT('',#55420);
#13434=VERTEX_POINT('',#55426);
#13435=VERTEX_POINT('',#55427);
#13436=VERTEX_POINT('',#55429);
#13437=VERTEX_POINT('',#55431);
#13438=VERTEX_POINT('',#55435);
#13439=VERTEX_POINT('',#55439);
#13440=VERTEX_POINT('',#55445);
#13441=VERTEX_POINT('',#55446);
#13442=VERTEX_POINT('',#55448);
#13443=VERTEX_POINT('',#55450);
#13444=VERTEX_POINT('',#55454);
#13445=VERTEX_POINT('',#55458);
#13446=VERTEX_POINT('',#55464);
#13447=VERTEX_POINT('',#55465);
#13448=VERTEX_POINT('',#55467);
#13449=VERTEX_POINT('',#55469);
#13450=VERTEX_POINT('',#55473);
#13451=VERTEX_POINT('',#55477);
#13452=VERTEX_POINT('',#55483);
#13453=VERTEX_POINT('',#55484);
#13454=VERTEX_POINT('',#55486);
#13455=VERTEX_POINT('',#55488);
#13456=VERTEX_POINT('',#55492);
#13457=VERTEX_POINT('',#55496);
#13458=VERTEX_POINT('',#55502);
#13459=VERTEX_POINT('',#55503);
#13460=VERTEX_POINT('',#55505);
#13461=VERTEX_POINT('',#55507);
#13462=VERTEX_POINT('',#55511);
#13463=VERTEX_POINT('',#55515);
#13464=VERTEX_POINT('',#55521);
#13465=VERTEX_POINT('',#55522);
#13466=VERTEX_POINT('',#55524);
#13467=VERTEX_POINT('',#55526);
#13468=VERTEX_POINT('',#55530);
#13469=VERTEX_POINT('',#55534);
#13470=VERTEX_POINT('',#55540);
#13471=VERTEX_POINT('',#55541);
#13472=VERTEX_POINT('',#55543);
#13473=VERTEX_POINT('',#55545);
#13474=VERTEX_POINT('',#55549);
#13475=VERTEX_POINT('',#55553);
#13476=VERTEX_POINT('',#55559);
#13477=VERTEX_POINT('',#55560);
#13478=VERTEX_POINT('',#55562);
#13479=VERTEX_POINT('',#55564);
#13480=VERTEX_POINT('',#55568);
#13481=VERTEX_POINT('',#55570);
#13482=VERTEX_POINT('',#55574);
#13483=VERTEX_POINT('',#55578);
#13484=VERTEX_POINT('',#55582);
#13485=VERTEX_POINT('',#55583);
#13486=VERTEX_POINT('',#55585);
#13487=VERTEX_POINT('',#55587);
#13488=VERTEX_POINT('',#55591);
#13489=VERTEX_POINT('',#55595);
#13490=VERTEX_POINT('',#55601);
#13491=VERTEX_POINT('',#55602);
#13492=VERTEX_POINT('',#55604);
#13493=VERTEX_POINT('',#55606);
#13494=VERTEX_POINT('',#55610);
#13495=VERTEX_POINT('',#55614);
#13496=VERTEX_POINT('',#55620);
#13497=VERTEX_POINT('',#55621);
#13498=VERTEX_POINT('',#55623);
#13499=VERTEX_POINT('',#55625);
#13500=VERTEX_POINT('',#55629);
#13501=VERTEX_POINT('',#55633);
#13502=VERTEX_POINT('',#55639);
#13503=VERTEX_POINT('',#55640);
#13504=VERTEX_POINT('',#55642);
#13505=VERTEX_POINT('',#55644);
#13506=VERTEX_POINT('',#55648);
#13507=VERTEX_POINT('',#55652);
#13508=VERTEX_POINT('',#55658);
#13509=VERTEX_POINT('',#55659);
#13510=VERTEX_POINT('',#55661);
#13511=VERTEX_POINT('',#55663);
#13512=VERTEX_POINT('',#55667);
#13513=VERTEX_POINT('',#55671);
#13514=VERTEX_POINT('',#55677);
#13515=VERTEX_POINT('',#55678);
#13516=VERTEX_POINT('',#55680);
#13517=VERTEX_POINT('',#55682);
#13518=VERTEX_POINT('',#55686);
#13519=VERTEX_POINT('',#55690);
#13520=VERTEX_POINT('',#55696);
#13521=VERTEX_POINT('',#55697);
#13522=VERTEX_POINT('',#55699);
#13523=VERTEX_POINT('',#55701);
#13524=VERTEX_POINT('',#55705);
#13525=VERTEX_POINT('',#55709);
#13526=VERTEX_POINT('',#55715);
#13527=VERTEX_POINT('',#55716);
#13528=VERTEX_POINT('',#55718);
#13529=VERTEX_POINT('',#55720);
#13530=VERTEX_POINT('',#55724);
#13531=VERTEX_POINT('',#55728);
#13532=VERTEX_POINT('',#55734);
#13533=VERTEX_POINT('',#55735);
#13534=VERTEX_POINT('',#55737);
#13535=VERTEX_POINT('',#55739);
#13536=VERTEX_POINT('',#55743);
#13537=VERTEX_POINT('',#55747);
#13538=VERTEX_POINT('',#55753);
#13539=VERTEX_POINT('',#55754);
#13540=VERTEX_POINT('',#55756);
#13541=VERTEX_POINT('',#55758);
#13542=VERTEX_POINT('',#55762);
#13543=VERTEX_POINT('',#55766);
#13544=VERTEX_POINT('',#55772);
#13545=VERTEX_POINT('',#55773);
#13546=VERTEX_POINT('',#55775);
#13547=VERTEX_POINT('',#55777);
#13548=VERTEX_POINT('',#55781);
#13549=VERTEX_POINT('',#55785);
#13550=VERTEX_POINT('',#55791);
#13551=VERTEX_POINT('',#55792);
#13552=VERTEX_POINT('',#55794);
#13553=VERTEX_POINT('',#55796);
#13554=VERTEX_POINT('',#55800);
#13555=VERTEX_POINT('',#55804);
#13556=VERTEX_POINT('',#55810);
#13557=VERTEX_POINT('',#55811);
#13558=VERTEX_POINT('',#55813);
#13559=VERTEX_POINT('',#55815);
#13560=VERTEX_POINT('',#55819);
#13561=VERTEX_POINT('',#55823);
#13562=VERTEX_POINT('',#55829);
#13563=VERTEX_POINT('',#55830);
#13564=VERTEX_POINT('',#55832);
#13565=VERTEX_POINT('',#55834);
#13566=VERTEX_POINT('',#55838);
#13567=VERTEX_POINT('',#55842);
#13568=VERTEX_POINT('',#55848);
#13569=VERTEX_POINT('',#55849);
#13570=VERTEX_POINT('',#55851);
#13571=VERTEX_POINT('',#55853);
#13572=VERTEX_POINT('',#55857);
#13573=VERTEX_POINT('',#55861);
#13574=VERTEX_POINT('',#55867);
#13575=VERTEX_POINT('',#55868);
#13576=VERTEX_POINT('',#55870);
#13577=VERTEX_POINT('',#55872);
#13578=VERTEX_POINT('',#55876);
#13579=VERTEX_POINT('',#55880);
#13580=VERTEX_POINT('',#55886);
#13581=VERTEX_POINT('',#55887);
#13582=VERTEX_POINT('',#55889);
#13583=VERTEX_POINT('',#55891);
#13584=VERTEX_POINT('',#55895);
#13585=VERTEX_POINT('',#55899);
#13586=VERTEX_POINT('',#55905);
#13587=VERTEX_POINT('',#55906);
#13588=VERTEX_POINT('',#55908);
#13589=VERTEX_POINT('',#55910);
#13590=VERTEX_POINT('',#55914);
#13591=VERTEX_POINT('',#55918);
#13592=VERTEX_POINT('',#55924);
#13593=VERTEX_POINT('',#55925);
#13594=VERTEX_POINT('',#55929);
#13595=VERTEX_POINT('',#55930);
#13596=VERTEX_POINT('',#55932);
#13597=VERTEX_POINT('',#55934);
#13598=VERTEX_POINT('',#55938);
#13599=VERTEX_POINT('',#55940);
#13600=VERTEX_POINT('',#55944);
#13601=VERTEX_POINT('',#55946);
#13602=VERTEX_POINT('',#55950);
#13603=VERTEX_POINT('',#55952);
#13604=VERTEX_POINT('',#55956);
#13605=VERTEX_POINT('',#55958);
#13606=VERTEX_POINT('',#55966);
#13607=VERTEX_POINT('',#55971);
#13608=VERTEX_POINT('',#55976);
#16763=EDGE_CURVE('',#13194,#13195,#8483,.T.);
#16764=EDGE_CURVE('',#13194,#13196,#2375,.T.);
#16765=EDGE_CURVE('',#13196,#13197,#1542,.T.);
#16766=EDGE_CURVE('',#13197,#13195,#2376,.T.);
#16767=EDGE_CURVE('',#13198,#13199,#8484,.T.);
#16768=EDGE_CURVE('',#13198,#13194,#2377,.T.);
#16769=EDGE_CURVE('',#13195,#13199,#2378,.T.);
#16770=EDGE_CURVE('',#13200,#13201,#8485,.T.);
#16771=EDGE_CURVE('',#13200,#13198,#2379,.T.);
#16772=EDGE_CURVE('',#13199,#13201,#2380,.T.);
#16773=EDGE_CURVE('',#13202,#13203,#8486,.T.);
#16774=EDGE_CURVE('',#13202,#13200,#2381,.T.);
#16775=EDGE_CURVE('',#13201,#13203,#2382,.T.);
#16776=EDGE_CURVE('',#13204,#13205,#8487,.T.);
#16777=EDGE_CURVE('',#13204,#13202,#2383,.T.);
#16778=EDGE_CURVE('',#13203,#13205,#2384,.T.);
#16779=EDGE_CURVE('',#13206,#13207,#8488,.T.);
#16780=EDGE_CURVE('',#13206,#13204,#2385,.T.);
#16781=EDGE_CURVE('',#13205,#13207,#2386,.T.);
#16782=EDGE_CURVE('',#13208,#13209,#8489,.T.);
#16783=EDGE_CURVE('',#13208,#13206,#2387,.T.);
#16784=EDGE_CURVE('',#13207,#13209,#2388,.T.);
#16785=EDGE_CURVE('',#13210,#13211,#8490,.T.);
#16786=EDGE_CURVE('',#13210,#13208,#2389,.T.);
#16787=EDGE_CURVE('',#13209,#13211,#2390,.T.);
#16788=EDGE_CURVE('',#13212,#13213,#8491,.T.);
#16789=EDGE_CURVE('',#13212,#13210,#2391,.T.);
#16790=EDGE_CURVE('',#13211,#13213,#2392,.T.);
#16791=EDGE_CURVE('',#13214,#13215,#8492,.T.);
#16792=EDGE_CURVE('',#13214,#13212,#2393,.T.);
#16793=EDGE_CURVE('',#13213,#13215,#2394,.T.);
#16794=EDGE_CURVE('',#13216,#13217,#8493,.T.);
#16795=EDGE_CURVE('',#13216,#13214,#2395,.T.);
#16796=EDGE_CURVE('',#13215,#13217,#2396,.T.);
#16797=EDGE_CURVE('',#13218,#13219,#8494,.T.);
#16798=EDGE_CURVE('',#13218,#13216,#2397,.T.);
#16799=EDGE_CURVE('',#13217,#13219,#2398,.T.);
#16800=EDGE_CURVE('',#13220,#13221,#8495,.T.);
#16801=EDGE_CURVE('',#13220,#13218,#2399,.T.);
#16802=EDGE_CURVE('',#13219,#13221,#2400,.T.);
#16803=EDGE_CURVE('',#13222,#13223,#8496,.T.);
#16804=EDGE_CURVE('',#13222,#13220,#2401,.T.);
#16805=EDGE_CURVE('',#13221,#13223,#2402,.T.);
#16806=EDGE_CURVE('',#13224,#13225,#8497,.T.);
#16807=EDGE_CURVE('',#13224,#13222,#2403,.T.);
#16808=EDGE_CURVE('',#13223,#13225,#2404,.T.);
#16809=EDGE_CURVE('',#13226,#13227,#8498,.T.);
#16810=EDGE_CURVE('',#13226,#13224,#2405,.T.);
#16811=EDGE_CURVE('',#13225,#13227,#2406,.T.);
#16812=EDGE_CURVE('',#13228,#13229,#8499,.T.);
#16813=EDGE_CURVE('',#13228,#13226,#2407,.T.);
#16814=EDGE_CURVE('',#13227,#13229,#2408,.T.);
#16815=EDGE_CURVE('',#13230,#13231,#8500,.T.);
#16816=EDGE_CURVE('',#13230,#13228,#2409,.T.);
#16817=EDGE_CURVE('',#13229,#13231,#2410,.T.);
#16818=EDGE_CURVE('',#13232,#13233,#8501,.T.);
#16819=EDGE_CURVE('',#13232,#13230,#2411,.T.);
#16820=EDGE_CURVE('',#13231,#13233,#2412,.T.);
#16821=EDGE_CURVE('',#13234,#13235,#8502,.T.);
#16822=EDGE_CURVE('',#13234,#13232,#2413,.T.);
#16823=EDGE_CURVE('',#13233,#13235,#2414,.T.);
#16824=EDGE_CURVE('',#13236,#13237,#8503,.T.);
#16825=EDGE_CURVE('',#13236,#13234,#2415,.T.);
#16826=EDGE_CURVE('',#13235,#13237,#2416,.T.);
#16827=EDGE_CURVE('',#13238,#13239,#8504,.T.);
#16828=EDGE_CURVE('',#13238,#13236,#2417,.T.);
#16829=EDGE_CURVE('',#13237,#13239,#2418,.T.);
#16830=EDGE_CURVE('',#13240,#13241,#8505,.T.);
#16831=EDGE_CURVE('',#13240,#13238,#2419,.T.);
#16832=EDGE_CURVE('',#13239,#13241,#2420,.T.);
#16833=EDGE_CURVE('',#13242,#13243,#8506,.T.);
#16834=EDGE_CURVE('',#13242,#13240,#2421,.T.);
#16835=EDGE_CURVE('',#13241,#13243,#2422,.T.);
#16836=EDGE_CURVE('',#13244,#13245,#8507,.T.);
#16837=EDGE_CURVE('',#13244,#13242,#2423,.T.);
#16838=EDGE_CURVE('',#13243,#13245,#2424,.T.);
#16839=EDGE_CURVE('',#13246,#13247,#8508,.T.);
#16840=EDGE_CURVE('',#13246,#13244,#2425,.T.);
#16841=EDGE_CURVE('',#13245,#13247,#2426,.T.);
#16842=EDGE_CURVE('',#13248,#13249,#8509,.T.);
#16843=EDGE_CURVE('',#13248,#13246,#2427,.T.);
#16844=EDGE_CURVE('',#13247,#13249,#2428,.T.);
#16845=EDGE_CURVE('',#13250,#13251,#8510,.T.);
#16846=EDGE_CURVE('',#13250,#13248,#2429,.T.);
#16847=EDGE_CURVE('',#13249,#13251,#2430,.T.);
#16848=EDGE_CURVE('',#13252,#13253,#8511,.T.);
#16849=EDGE_CURVE('',#13252,#13250,#2431,.T.);
#16850=EDGE_CURVE('',#13251,#13253,#2432,.T.);
#16851=EDGE_CURVE('',#13254,#13255,#8512,.T.);
#16852=EDGE_CURVE('',#13254,#13252,#2433,.T.);
#16853=EDGE_CURVE('',#13253,#13255,#2434,.T.);
#16854=EDGE_CURVE('',#13256,#13257,#8513,.T.);
#16855=EDGE_CURVE('',#13256,#13254,#2435,.T.);
#16856=EDGE_CURVE('',#13255,#13257,#2436,.T.);
#16857=EDGE_CURVE('',#13258,#13259,#8514,.T.);
#16858=EDGE_CURVE('',#13258,#13256,#2437,.T.);
#16859=EDGE_CURVE('',#13257,#13259,#2438,.T.);
#16860=EDGE_CURVE('',#13260,#13261,#8515,.T.);
#16861=EDGE_CURVE('',#13260,#13258,#2439,.T.);
#16862=EDGE_CURVE('',#13259,#13261,#2440,.T.);
#16863=EDGE_CURVE('',#13262,#13263,#8516,.T.);
#16864=EDGE_CURVE('',#13262,#13260,#2441,.T.);
#16865=EDGE_CURVE('',#13261,#13263,#2442,.T.);
#16866=EDGE_CURVE('',#13264,#13265,#8517,.T.);
#16867=EDGE_CURVE('',#13264,#13262,#2443,.T.);
#16868=EDGE_CURVE('',#13263,#13265,#2444,.T.);
#16869=EDGE_CURVE('',#13266,#13267,#8518,.T.);
#16870=EDGE_CURVE('',#13266,#13264,#2445,.T.);
#16871=EDGE_CURVE('',#13265,#13267,#2446,.T.);
#16872=EDGE_CURVE('',#13268,#13269,#8519,.T.);
#16873=EDGE_CURVE('',#13268,#13266,#2447,.T.);
#16874=EDGE_CURVE('',#13267,#13269,#2448,.T.);
#16875=EDGE_CURVE('',#13270,#13271,#8520,.T.);
#16876=EDGE_CURVE('',#13270,#13268,#2449,.T.);
#16877=EDGE_CURVE('',#13269,#13271,#2450,.T.);
#16878=EDGE_CURVE('',#13272,#13273,#8521,.T.);
#16879=EDGE_CURVE('',#13272,#13270,#2451,.T.);
#16880=EDGE_CURVE('',#13271,#13273,#2452,.T.);
#16881=EDGE_CURVE('',#13274,#13275,#8522,.T.);
#16882=EDGE_CURVE('',#13274,#13272,#2453,.T.);
#16883=EDGE_CURVE('',#13273,#13275,#2454,.T.);
#16884=EDGE_CURVE('',#13276,#13277,#8523,.T.);
#16885=EDGE_CURVE('',#13276,#13274,#2455,.T.);
#16886=EDGE_CURVE('',#13275,#13277,#2456,.T.);
#16887=EDGE_CURVE('',#13278,#13279,#8524,.T.);
#16888=EDGE_CURVE('',#13278,#13276,#2457,.T.);
#16889=EDGE_CURVE('',#13277,#13279,#2458,.T.);
#16890=EDGE_CURVE('',#13280,#13281,#8525,.T.);
#16891=EDGE_CURVE('',#13280,#13282,#2459,.T.);
#16892=EDGE_CURVE('',#13283,#13282,#1543,.T.);
#16893=EDGE_CURVE('',#13281,#13283,#2460,.T.);
#16894=EDGE_CURVE('',#13284,#13285,#8526,.T.);
#16895=EDGE_CURVE('',#13284,#13280,#2461,.T.);
#16896=EDGE_CURVE('',#13285,#13281,#2462,.T.);
#16897=EDGE_CURVE('',#13286,#13287,#8527,.T.);
#16898=EDGE_CURVE('',#13286,#13284,#2463,.T.);
#16899=EDGE_CURVE('',#13287,#13285,#2464,.T.);
#16900=EDGE_CURVE('',#13288,#13289,#8528,.T.);
#16901=EDGE_CURVE('',#13288,#13286,#2465,.T.);
#16902=EDGE_CURVE('',#13289,#13287,#2466,.T.);
#16903=EDGE_CURVE('',#13290,#13291,#8529,.T.);
#16904=EDGE_CURVE('',#13290,#13288,#2467,.T.);
#16905=EDGE_CURVE('',#13291,#13289,#2468,.T.);
#16906=EDGE_CURVE('',#13292,#13293,#8530,.T.);
#16907=EDGE_CURVE('',#13292,#13290,#2469,.T.);
#16908=EDGE_CURVE('',#13293,#13291,#2470,.T.);
#16909=EDGE_CURVE('',#13294,#13295,#8531,.T.);
#16910=EDGE_CURVE('',#13294,#13292,#2471,.T.);
#16911=EDGE_CURVE('',#13295,#13293,#2472,.T.);
#16912=EDGE_CURVE('',#13296,#13297,#8532,.T.);
#16913=EDGE_CURVE('',#13296,#13294,#2473,.T.);
#16914=EDGE_CURVE('',#13297,#13295,#2474,.T.);
#16915=EDGE_CURVE('',#13298,#13299,#8533,.T.);
#16916=EDGE_CURVE('',#13298,#13296,#2475,.T.);
#16917=EDGE_CURVE('',#13299,#13297,#2476,.T.);
#16918=EDGE_CURVE('',#13300,#13301,#8534,.T.);
#16919=EDGE_CURVE('',#13300,#13298,#2477,.T.);
#16920=EDGE_CURVE('',#13301,#13299,#2478,.T.);
#16921=EDGE_CURVE('',#13302,#13303,#8535,.T.);
#16922=EDGE_CURVE('',#13302,#13300,#2479,.T.);
#16923=EDGE_CURVE('',#13303,#13301,#2480,.T.);
#16924=EDGE_CURVE('',#13304,#13305,#8536,.T.);
#16925=EDGE_CURVE('',#13304,#13302,#2481,.T.);
#16926=EDGE_CURVE('',#13305,#13303,#2482,.T.);
#16927=EDGE_CURVE('',#13306,#13307,#8537,.T.);
#16928=EDGE_CURVE('',#13306,#13304,#2483,.T.);
#16929=EDGE_CURVE('',#13307,#13305,#2484,.T.);
#16930=EDGE_CURVE('',#13308,#13309,#8538,.T.);
#16931=EDGE_CURVE('',#13308,#13306,#2485,.T.);
#16932=EDGE_CURVE('',#13309,#13307,#2486,.T.);
#16933=EDGE_CURVE('',#13310,#13311,#8539,.T.);
#16934=EDGE_CURVE('',#13310,#13308,#2487,.T.);
#16935=EDGE_CURVE('',#13311,#13309,#2488,.T.);
#16936=EDGE_CURVE('',#13312,#13313,#8540,.T.);
#16937=EDGE_CURVE('',#13312,#13310,#2489,.T.);
#16938=EDGE_CURVE('',#13313,#13311,#2490,.T.);
#16939=EDGE_CURVE('',#13314,#13315,#8541,.T.);
#16940=EDGE_CURVE('',#13314,#13312,#2491,.T.);
#16941=EDGE_CURVE('',#13315,#13313,#2492,.T.);
#16942=EDGE_CURVE('',#13316,#13317,#8542,.T.);
#16943=EDGE_CURVE('',#13316,#13314,#2493,.T.);
#16944=EDGE_CURVE('',#13317,#13315,#2494,.T.);
#16945=EDGE_CURVE('',#13318,#13319,#8543,.T.);
#16946=EDGE_CURVE('',#13318,#13316,#2495,.T.);
#16947=EDGE_CURVE('',#13319,#13317,#2496,.T.);
#16948=EDGE_CURVE('',#13320,#13321,#8544,.T.);
#16949=EDGE_CURVE('',#13320,#13318,#2497,.T.);
#16950=EDGE_CURVE('',#13321,#13319,#2498,.T.);
#16951=EDGE_CURVE('',#13322,#13323,#8545,.T.);
#16952=EDGE_CURVE('',#13322,#13320,#2499,.T.);
#16953=EDGE_CURVE('',#13323,#13321,#2500,.T.);
#16954=EDGE_CURVE('',#13324,#13325,#8546,.T.);
#16955=EDGE_CURVE('',#13324,#13322,#2501,.T.);
#16956=EDGE_CURVE('',#13325,#13323,#2502,.T.);
#16957=EDGE_CURVE('',#13326,#13327,#8547,.T.);
#16958=EDGE_CURVE('',#13326,#13324,#2503,.T.);
#16959=EDGE_CURVE('',#13327,#13325,#2504,.T.);
#16960=EDGE_CURVE('',#13328,#13329,#8548,.T.);
#16961=EDGE_CURVE('',#13328,#13326,#2505,.T.);
#16962=EDGE_CURVE('',#13329,#13327,#2506,.T.);
#16963=EDGE_CURVE('',#13330,#13331,#8549,.T.);
#16964=EDGE_CURVE('',#13330,#13328,#2507,.T.);
#16965=EDGE_CURVE('',#13331,#13329,#2508,.T.);
#16966=EDGE_CURVE('',#13332,#13333,#8550,.T.);
#16967=EDGE_CURVE('',#13332,#13330,#2509,.T.);
#16968=EDGE_CURVE('',#13333,#13331,#2510,.T.);
#16969=EDGE_CURVE('',#13334,#13335,#8551,.T.);
#16970=EDGE_CURVE('',#13334,#13332,#2511,.T.);
#16971=EDGE_CURVE('',#13335,#13333,#2512,.T.);
#16972=EDGE_CURVE('',#13336,#13337,#8552,.T.);
#16973=EDGE_CURVE('',#13336,#13334,#2513,.T.);
#16974=EDGE_CURVE('',#13337,#13335,#2514,.T.);
#16975=EDGE_CURVE('',#13338,#13339,#8553,.T.);
#16976=EDGE_CURVE('',#13338,#13336,#2515,.T.);
#16977=EDGE_CURVE('',#13339,#13337,#2516,.T.);
#16978=EDGE_CURVE('',#13340,#13341,#8554,.T.);
#16979=EDGE_CURVE('',#13340,#13338,#2517,.T.);
#16980=EDGE_CURVE('',#13341,#13339,#2518,.T.);
#16981=EDGE_CURVE('',#13342,#13343,#8555,.T.);
#16982=EDGE_CURVE('',#13342,#13340,#2519,.T.);
#16983=EDGE_CURVE('',#13343,#13341,#2520,.T.);
#16984=EDGE_CURVE('',#13344,#13345,#8556,.T.);
#16985=EDGE_CURVE('',#13344,#13342,#2521,.T.);
#16986=EDGE_CURVE('',#13345,#13343,#2522,.T.);
#16987=EDGE_CURVE('',#13346,#13347,#8557,.T.);
#16988=EDGE_CURVE('',#13346,#13344,#2523,.T.);
#16989=EDGE_CURVE('',#13347,#13345,#2524,.T.);
#16990=EDGE_CURVE('',#13348,#13349,#8558,.T.);
#16991=EDGE_CURVE('',#13348,#13346,#2525,.T.);
#16992=EDGE_CURVE('',#13349,#13347,#2526,.T.);
#16993=EDGE_CURVE('',#13350,#13351,#8559,.T.);
#16994=EDGE_CURVE('',#13350,#13348,#2527,.T.);
#16995=EDGE_CURVE('',#13351,#13349,#2528,.T.);
#16996=EDGE_CURVE('',#13352,#13353,#8560,.T.);
#16997=EDGE_CURVE('',#13352,#13350,#2529,.T.);
#16998=EDGE_CURVE('',#13353,#13351,#2530,.T.);
#16999=EDGE_CURVE('',#13354,#13355,#8561,.T.);
#17000=EDGE_CURVE('',#13354,#13352,#2531,.T.);
#17001=EDGE_CURVE('',#13355,#13353,#2532,.T.);
#17002=EDGE_CURVE('',#13356,#13357,#8562,.T.);
#17003=EDGE_CURVE('',#13356,#13354,#2533,.T.);
#17004=EDGE_CURVE('',#13357,#13355,#2534,.T.);
#17005=EDGE_CURVE('',#13358,#13359,#8563,.T.);
#17006=EDGE_CURVE('',#13358,#13356,#2535,.T.);
#17007=EDGE_CURVE('',#13359,#13357,#2536,.T.);
#17008=EDGE_CURVE('',#13360,#13361,#8564,.T.);
#17009=EDGE_CURVE('',#13360,#13358,#2537,.T.);
#17010=EDGE_CURVE('',#13361,#13359,#2538,.T.);
#17011=EDGE_CURVE('',#13362,#13363,#8565,.T.);
#17012=EDGE_CURVE('',#13362,#13360,#2539,.T.);
#17013=EDGE_CURVE('',#13363,#13361,#2540,.T.);
#17014=EDGE_CURVE('',#13364,#13365,#8566,.T.);
#17015=EDGE_CURVE('',#13364,#13362,#2541,.T.);
#17016=EDGE_CURVE('',#13365,#13363,#2542,.T.);
#17017=EDGE_CURVE('',#13282,#13366,#2543,.T.);
#17018=EDGE_CURVE('',#13367,#13366,#1544,.T.);
#17019=EDGE_CURVE('',#13367,#13283,#2544,.T.);
#17020=EDGE_CURVE('',#13279,#13367,#2545,.T.);
#17021=EDGE_CURVE('',#13368,#13197,#2546,.T.);
#17022=EDGE_CURVE('',#13368,#13365,#2547,.T.);
#17023=EDGE_CURVE('',#13197,#13369,#1545,.T.);
#17024=EDGE_CURVE('',#13369,#13196,#1546,.T.);
#17025=EDGE_CURVE('',#13196,#13370,#2548,.T.);
#17026=EDGE_CURVE('',#13370,#13368,#1547,.T.);
#17027=EDGE_CURVE('',#13370,#13364,#2549,.T.);
#17028=EDGE_CURVE('',#13366,#13278,#2550,.T.);
#17029=EDGE_CURVE('',#13366,#13371,#1548,.T.);
#17030=EDGE_CURVE('',#13371,#13372,#1549,.T.);
#17031=EDGE_CURVE('',#13372,#13372,#1550,.T.);
#17032=EDGE_CURVE('',#13371,#13367,#1551,.T.);
#17033=EDGE_CURVE('',#13373,#13373,#1552,.T.);
#17034=EDGE_CURVE('',#13374,#13375,#8567,.T.);
#17035=EDGE_CURVE('',#13374,#13376,#8568,.T.);
#17036=EDGE_CURVE('',#13377,#13376,#8569,.T.);
#17037=EDGE_CURVE('',#13375,#13377,#8570,.T.);
#17038=EDGE_CURVE('',#13375,#13378,#1553,.T.);
#17039=EDGE_CURVE('',#13377,#13378,#8571,.T.);
#17040=EDGE_CURVE('',#13378,#13379,#8572,.T.);
#17041=EDGE_CURVE('',#13376,#13379,#8573,.T.);
#17042=EDGE_CURVE('',#13379,#13374,#1554,.T.);
#17043=EDGE_CURVE('',#13380,#13381,#8574,.T.);
#17044=EDGE_CURVE('',#13380,#13382,#8575,.T.);
#17045=EDGE_CURVE('',#13383,#13382,#8576,.T.);
#17046=EDGE_CURVE('',#13381,#13383,#8577,.T.);
#17047=EDGE_CURVE('',#13381,#13384,#1555,.T.);
#17048=EDGE_CURVE('',#13383,#13384,#8578,.T.);
#17049=EDGE_CURVE('',#13384,#13385,#8579,.T.);
#17050=EDGE_CURVE('',#13382,#13385,#8580,.T.);
#17051=EDGE_CURVE('',#13385,#13380,#1556,.T.);
#17052=EDGE_CURVE('',#13386,#13387,#8581,.T.);
#17053=EDGE_CURVE('',#13386,#13388,#8582,.T.);
#17054=EDGE_CURVE('',#13389,#13388,#8583,.T.);
#17055=EDGE_CURVE('',#13387,#13389,#8584,.T.);
#17056=EDGE_CURVE('',#13387,#13390,#1557,.T.);
#17057=EDGE_CURVE('',#13389,#13390,#8585,.T.);
#17058=EDGE_CURVE('',#13390,#13391,#8586,.T.);
#17059=EDGE_CURVE('',#13388,#13391,#8587,.T.);
#17060=EDGE_CURVE('',#13391,#13386,#1558,.T.);
#17061=EDGE_CURVE('',#13392,#13393,#8588,.T.);
#17062=EDGE_CURVE('',#13392,#13394,#8589,.T.);
#17063=EDGE_CURVE('',#13395,#13394,#8590,.T.);
#17064=EDGE_CURVE('',#13393,#13395,#8591,.T.);
#17065=EDGE_CURVE('',#13393,#13396,#1559,.T.);
#17066=EDGE_CURVE('',#13395,#13396,#8592,.T.);
#17067=EDGE_CURVE('',#13396,#13397,#8593,.T.);
#17068=EDGE_CURVE('',#13394,#13397,#8594,.T.);
#17069=EDGE_CURVE('',#13397,#13392,#1560,.T.);
#17070=EDGE_CURVE('',#13398,#13399,#8595,.T.);
#17071=EDGE_CURVE('',#13398,#13400,#8596,.T.);
#17072=EDGE_CURVE('',#13401,#13400,#8597,.T.);
#17073=EDGE_CURVE('',#13399,#13401,#8598,.T.);
#17074=EDGE_CURVE('',#13399,#13402,#1561,.T.);
#17075=EDGE_CURVE('',#13401,#13402,#8599,.T.);
#17076=EDGE_CURVE('',#13402,#13403,#8600,.T.);
#17077=EDGE_CURVE('',#13400,#13403,#8601,.T.);
#17078=EDGE_CURVE('',#13403,#13398,#1562,.T.);
#17079=EDGE_CURVE('',#13404,#13405,#8602,.T.);
#17080=EDGE_CURVE('',#13404,#13406,#8603,.T.);
#17081=EDGE_CURVE('',#13407,#13406,#8604,.T.);
#17082=EDGE_CURVE('',#13405,#13407,#8605,.T.);
#17083=EDGE_CURVE('',#13405,#13408,#1563,.T.);
#17084=EDGE_CURVE('',#13407,#13408,#8606,.T.);
#17085=EDGE_CURVE('',#13408,#13409,#8607,.T.);
#17086=EDGE_CURVE('',#13406,#13409,#8608,.T.);
#17087=EDGE_CURVE('',#13409,#13404,#1564,.T.);
#17088=EDGE_CURVE('',#13410,#13411,#8609,.T.);
#17089=EDGE_CURVE('',#13410,#13412,#8610,.T.);
#17090=EDGE_CURVE('',#13413,#13412,#8611,.T.);
#17091=EDGE_CURVE('',#13411,#13413,#8612,.T.);
#17092=EDGE_CURVE('',#13411,#13414,#1565,.T.);
#17093=EDGE_CURVE('',#13413,#13414,#8613,.T.);
#17094=EDGE_CURVE('',#13414,#13415,#8614,.T.);
#17095=EDGE_CURVE('',#13412,#13415,#8615,.T.);
#17096=EDGE_CURVE('',#13415,#13410,#1566,.T.);
#17097=EDGE_CURVE('',#13416,#13417,#8616,.T.);
#17098=EDGE_CURVE('',#13416,#13418,#8617,.T.);
#17099=EDGE_CURVE('',#13419,#13418,#8618,.T.);
#17100=EDGE_CURVE('',#13417,#13419,#8619,.T.);
#17101=EDGE_CURVE('',#13417,#13420,#1567,.T.);
#17102=EDGE_CURVE('',#13419,#13420,#8620,.T.);
#17103=EDGE_CURVE('',#13420,#13421,#8621,.T.);
#17104=EDGE_CURVE('',#13418,#13421,#8622,.T.);
#17105=EDGE_CURVE('',#13421,#13416,#1568,.T.);
#17106=EDGE_CURVE('',#13422,#13423,#8623,.T.);
#17107=EDGE_CURVE('',#13422,#13424,#8624,.T.);
#17108=EDGE_CURVE('',#13425,#13424,#8625,.T.);
#17109=EDGE_CURVE('',#13423,#13425,#8626,.T.);
#17110=EDGE_CURVE('',#13423,#13426,#1569,.T.);
#17111=EDGE_CURVE('',#13425,#13426,#8627,.T.);
#17112=EDGE_CURVE('',#13426,#13427,#8628,.T.);
#17113=EDGE_CURVE('',#13424,#13427,#8629,.T.);
#17114=EDGE_CURVE('',#13427,#13422,#1570,.T.);
#17115=EDGE_CURVE('',#13428,#13429,#8630,.T.);
#17116=EDGE_CURVE('',#13428,#13430,#8631,.T.);
#17117=EDGE_CURVE('',#13431,#13430,#8632,.T.);
#17118=EDGE_CURVE('',#13429,#13431,#8633,.T.);
#17119=EDGE_CURVE('',#13429,#13432,#1571,.T.);
#17120=EDGE_CURVE('',#13431,#13432,#8634,.T.);
#17121=EDGE_CURVE('',#13432,#13433,#8635,.T.);
#17122=EDGE_CURVE('',#13430,#13433,#8636,.T.);
#17123=EDGE_CURVE('',#13433,#13428,#1572,.T.);
#17124=EDGE_CURVE('',#13434,#13435,#8637,.T.);
#17125=EDGE_CURVE('',#13434,#13436,#8638,.T.);
#17126=EDGE_CURVE('',#13437,#13436,#8639,.T.);
#17127=EDGE_CURVE('',#13435,#13437,#8640,.T.);
#17128=EDGE_CURVE('',#13435,#13438,#1573,.T.);
#17129=EDGE_CURVE('',#13437,#13438,#8641,.T.);
#17130=EDGE_CURVE('',#13438,#13439,#8642,.T.);
#17131=EDGE_CURVE('',#13436,#13439,#8643,.T.);
#17132=EDGE_CURVE('',#13439,#13434,#1574,.T.);
#17133=EDGE_CURVE('',#13440,#13441,#8644,.T.);
#17134=EDGE_CURVE('',#13440,#13442,#8645,.T.);
#17135=EDGE_CURVE('',#13443,#13442,#8646,.T.);
#17136=EDGE_CURVE('',#13441,#13443,#8647,.T.);
#17137=EDGE_CURVE('',#13441,#13444,#1575,.T.);
#17138=EDGE_CURVE('',#13443,#13444,#8648,.T.);
#17139=EDGE_CURVE('',#13444,#13445,#8649,.T.);
#17140=EDGE_CURVE('',#13442,#13445,#8650,.T.);
#17141=EDGE_CURVE('',#13445,#13440,#1576,.T.);
#17142=EDGE_CURVE('',#13446,#13447,#8651,.T.);
#17143=EDGE_CURVE('',#13446,#13448,#8652,.T.);
#17144=EDGE_CURVE('',#13449,#13448,#8653,.T.);
#17145=EDGE_CURVE('',#13447,#13449,#8654,.T.);
#17146=EDGE_CURVE('',#13447,#13450,#1577,.T.);
#17147=EDGE_CURVE('',#13449,#13450,#8655,.T.);
#17148=EDGE_CURVE('',#13450,#13451,#8656,.T.);
#17149=EDGE_CURVE('',#13448,#13451,#8657,.T.);
#17150=EDGE_CURVE('',#13451,#13446,#1578,.T.);
#17151=EDGE_CURVE('',#13452,#13453,#8658,.T.);
#17152=EDGE_CURVE('',#13452,#13454,#8659,.T.);
#17153=EDGE_CURVE('',#13455,#13454,#8660,.T.);
#17154=EDGE_CURVE('',#13453,#13455,#8661,.T.);
#17155=EDGE_CURVE('',#13453,#13456,#1579,.T.);
#17156=EDGE_CURVE('',#13455,#13456,#8662,.T.);
#17157=EDGE_CURVE('',#13456,#13457,#8663,.T.);
#17158=EDGE_CURVE('',#13454,#13457,#8664,.T.);
#17159=EDGE_CURVE('',#13457,#13452,#1580,.T.);
#17160=EDGE_CURVE('',#13458,#13459,#8665,.T.);
#17161=EDGE_CURVE('',#13458,#13460,#8666,.T.);
#17162=EDGE_CURVE('',#13461,#13460,#8667,.T.);
#17163=EDGE_CURVE('',#13459,#13461,#8668,.T.);
#17164=EDGE_CURVE('',#13459,#13462,#1581,.T.);
#17165=EDGE_CURVE('',#13461,#13462,#8669,.T.);
#17166=EDGE_CURVE('',#13462,#13463,#8670,.T.);
#17167=EDGE_CURVE('',#13460,#13463,#8671,.T.);
#17168=EDGE_CURVE('',#13463,#13458,#1582,.T.);
#17169=EDGE_CURVE('',#13464,#13465,#8672,.T.);
#17170=EDGE_CURVE('',#13464,#13466,#8673,.T.);
#17171=EDGE_CURVE('',#13467,#13466,#8674,.T.);
#17172=EDGE_CURVE('',#13465,#13467,#8675,.T.);
#17173=EDGE_CURVE('',#13465,#13468,#1583,.T.);
#17174=EDGE_CURVE('',#13467,#13468,#8676,.T.);
#17175=EDGE_CURVE('',#13468,#13469,#8677,.T.);
#17176=EDGE_CURVE('',#13466,#13469,#8678,.T.);
#17177=EDGE_CURVE('',#13469,#13464,#1584,.T.);
#17178=EDGE_CURVE('',#13470,#13471,#8679,.T.);
#17179=EDGE_CURVE('',#13470,#13472,#8680,.T.);
#17180=EDGE_CURVE('',#13473,#13472,#8681,.T.);
#17181=EDGE_CURVE('',#13471,#13473,#8682,.T.);
#17182=EDGE_CURVE('',#13471,#13474,#1585,.T.);
#17183=EDGE_CURVE('',#13473,#13474,#8683,.T.);
#17184=EDGE_CURVE('',#13474,#13475,#8684,.T.);
#17185=EDGE_CURVE('',#13472,#13475,#8685,.T.);
#17186=EDGE_CURVE('',#13475,#13470,#1586,.T.);
#17187=EDGE_CURVE('',#13476,#13477,#8686,.T.);
#17188=EDGE_CURVE('',#13476,#13478,#8687,.T.);
#17189=EDGE_CURVE('',#13479,#13478,#8688,.T.);
#17190=EDGE_CURVE('',#13477,#13479,#8689,.T.);
#17191=EDGE_CURVE('',#13477,#13480,#1587,.T.);
#17192=EDGE_CURVE('',#13479,#13481,#8690,.T.);
#17193=EDGE_CURVE('',#13480,#13481,#1588,.T.);
#17194=EDGE_CURVE('',#13481,#13482,#8691,.T.);
#17195=EDGE_CURVE('',#13478,#13482,#8692,.T.);
#17196=EDGE_CURVE('',#13482,#13483,#1589,.T.);
#17197=EDGE_CURVE('',#13483,#13476,#1590,.T.);
#17198=EDGE_CURVE('',#13484,#13485,#8693,.T.);
#17199=EDGE_CURVE('',#13484,#13486,#8694,.T.);
#17200=EDGE_CURVE('',#13487,#13486,#8695,.T.);
#17201=EDGE_CURVE('',#13485,#13487,#8696,.T.);
#17202=EDGE_CURVE('',#13485,#13488,#1591,.T.);
#17203=EDGE_CURVE('',#13487,#13488,#8697,.T.);
#17204=EDGE_CURVE('',#13488,#13489,#8698,.T.);
#17205=EDGE_CURVE('',#13486,#13489,#8699,.T.);
#17206=EDGE_CURVE('',#13489,#13484,#1592,.T.);
#17207=EDGE_CURVE('',#13490,#13491,#8700,.T.);
#17208=EDGE_CURVE('',#13490,#13492,#8701,.T.);
#17209=EDGE_CURVE('',#13493,#13492,#8702,.T.);
#17210=EDGE_CURVE('',#13491,#13493,#8703,.T.);
#17211=EDGE_CURVE('',#13491,#13494,#1593,.T.);
#17212=EDGE_CURVE('',#13493,#13494,#8704,.T.);
#17213=EDGE_CURVE('',#13494,#13495,#8705,.T.);
#17214=EDGE_CURVE('',#13492,#13495,#8706,.T.);
#17215=EDGE_CURVE('',#13495,#13490,#1594,.T.);
#17216=EDGE_CURVE('',#13496,#13497,#8707,.T.);
#17217=EDGE_CURVE('',#13496,#13498,#8708,.T.);
#17218=EDGE_CURVE('',#13499,#13498,#8709,.T.);
#17219=EDGE_CURVE('',#13497,#13499,#8710,.T.);
#17220=EDGE_CURVE('',#13497,#13500,#1595,.T.);
#17221=EDGE_CURVE('',#13499,#13500,#8711,.T.);
#17222=EDGE_CURVE('',#13500,#13501,#8712,.T.);
#17223=EDGE_CURVE('',#13498,#13501,#8713,.T.);
#17224=EDGE_CURVE('',#13501,#13496,#1596,.T.);
#17225=EDGE_CURVE('',#13502,#13503,#8714,.T.);
#17226=EDGE_CURVE('',#13502,#13504,#8715,.T.);
#17227=EDGE_CURVE('',#13505,#13504,#8716,.T.);
#17228=EDGE_CURVE('',#13503,#13505,#8717,.T.);
#17229=EDGE_CURVE('',#13503,#13506,#1597,.T.);
#17230=EDGE_CURVE('',#13505,#13506,#8718,.T.);
#17231=EDGE_CURVE('',#13506,#13507,#8719,.T.);
#17232=EDGE_CURVE('',#13504,#13507,#8720,.T.);
#17233=EDGE_CURVE('',#13507,#13502,#1598,.T.);
#17234=EDGE_CURVE('',#13508,#13509,#8721,.T.);
#17235=EDGE_CURVE('',#13508,#13510,#8722,.T.);
#17236=EDGE_CURVE('',#13511,#13510,#8723,.T.);
#17237=EDGE_CURVE('',#13509,#13511,#8724,.T.);
#17238=EDGE_CURVE('',#13509,#13512,#1599,.T.);
#17239=EDGE_CURVE('',#13511,#13512,#8725,.T.);
#17240=EDGE_CURVE('',#13512,#13513,#8726,.T.);
#17241=EDGE_CURVE('',#13510,#13513,#8727,.T.);
#17242=EDGE_CURVE('',#13513,#13508,#1600,.T.);
#17243=EDGE_CURVE('',#13514,#13515,#8728,.T.);
#17244=EDGE_CURVE('',#13514,#13516,#8729,.T.);
#17245=EDGE_CURVE('',#13517,#13516,#8730,.T.);
#17246=EDGE_CURVE('',#13515,#13517,#8731,.T.);
#17247=EDGE_CURVE('',#13515,#13518,#1601,.T.);
#17248=EDGE_CURVE('',#13517,#13518,#8732,.T.);
#17249=EDGE_CURVE('',#13518,#13519,#8733,.T.);
#17250=EDGE_CURVE('',#13516,#13519,#8734,.T.);
#17251=EDGE_CURVE('',#13519,#13514,#1602,.T.);
#17252=EDGE_CURVE('',#13520,#13521,#8735,.T.);
#17253=EDGE_CURVE('',#13520,#13522,#8736,.T.);
#17254=EDGE_CURVE('',#13523,#13522,#8737,.T.);
#17255=EDGE_CURVE('',#13521,#13523,#8738,.T.);
#17256=EDGE_CURVE('',#13521,#13524,#1603,.T.);
#17257=EDGE_CURVE('',#13523,#13524,#8739,.T.);
#17258=EDGE_CURVE('',#13524,#13525,#8740,.T.);
#17259=EDGE_CURVE('',#13522,#13525,#8741,.T.);
#17260=EDGE_CURVE('',#13525,#13520,#1604,.T.);
#17261=EDGE_CURVE('',#13526,#13527,#8742,.T.);
#17262=EDGE_CURVE('',#13526,#13528,#8743,.T.);
#17263=EDGE_CURVE('',#13529,#13528,#8744,.T.);
#17264=EDGE_CURVE('',#13527,#13529,#8745,.T.);
#17265=EDGE_CURVE('',#13527,#13530,#1605,.T.);
#17266=EDGE_CURVE('',#13529,#13530,#8746,.T.);
#17267=EDGE_CURVE('',#13530,#13531,#8747,.T.);
#17268=EDGE_CURVE('',#13528,#13531,#8748,.T.);
#17269=EDGE_CURVE('',#13531,#13526,#1606,.T.);
#17270=EDGE_CURVE('',#13532,#13533,#8749,.T.);
#17271=EDGE_CURVE('',#13532,#13534,#8750,.T.);
#17272=EDGE_CURVE('',#13535,#13534,#8751,.T.);
#17273=EDGE_CURVE('',#13533,#13535,#8752,.T.);
#17274=EDGE_CURVE('',#13533,#13536,#1607,.T.);
#17275=EDGE_CURVE('',#13535,#13536,#8753,.T.);
#17276=EDGE_CURVE('',#13536,#13537,#8754,.T.);
#17277=EDGE_CURVE('',#13534,#13537,#8755,.T.);
#17278=EDGE_CURVE('',#13537,#13532,#1608,.T.);
#17279=EDGE_CURVE('',#13538,#13539,#8756,.T.);
#17280=EDGE_CURVE('',#13538,#13540,#8757,.T.);
#17281=EDGE_CURVE('',#13541,#13540,#8758,.T.);
#17282=EDGE_CURVE('',#13539,#13541,#8759,.T.);
#17283=EDGE_CURVE('',#13539,#13542,#1609,.T.);
#17284=EDGE_CURVE('',#13541,#13542,#8760,.T.);
#17285=EDGE_CURVE('',#13542,#13543,#8761,.T.);
#17286=EDGE_CURVE('',#13540,#13543,#8762,.T.);
#17287=EDGE_CURVE('',#13543,#13538,#1610,.T.);
#17288=EDGE_CURVE('',#13544,#13545,#8763,.T.);
#17289=EDGE_CURVE('',#13544,#13546,#8764,.T.);
#17290=EDGE_CURVE('',#13547,#13546,#8765,.T.);
#17291=EDGE_CURVE('',#13545,#13547,#8766,.T.);
#17292=EDGE_CURVE('',#13545,#13548,#1611,.T.);
#17293=EDGE_CURVE('',#13547,#13548,#8767,.T.);
#17294=EDGE_CURVE('',#13548,#13549,#8768,.T.);
#17295=EDGE_CURVE('',#13546,#13549,#8769,.T.);
#17296=EDGE_CURVE('',#13549,#13544,#1612,.T.);
#17297=EDGE_CURVE('',#13550,#13551,#8770,.T.);
#17298=EDGE_CURVE('',#13550,#13552,#8771,.T.);
#17299=EDGE_CURVE('',#13553,#13552,#8772,.T.);
#17300=EDGE_CURVE('',#13551,#13553,#8773,.T.);
#17301=EDGE_CURVE('',#13551,#13554,#1613,.T.);
#17302=EDGE_CURVE('',#13553,#13554,#8774,.T.);
#17303=EDGE_CURVE('',#13554,#13555,#8775,.T.);
#17304=EDGE_CURVE('',#13552,#13555,#8776,.T.);
#17305=EDGE_CURVE('',#13555,#13550,#1614,.T.);
#17306=EDGE_CURVE('',#13556,#13557,#8777,.T.);
#17307=EDGE_CURVE('',#13556,#13558,#8778,.T.);
#17308=EDGE_CURVE('',#13559,#13558,#8779,.T.);
#17309=EDGE_CURVE('',#13557,#13559,#8780,.T.);
#17310=EDGE_CURVE('',#13557,#13560,#1615,.T.);
#17311=EDGE_CURVE('',#13559,#13560,#8781,.T.);
#17312=EDGE_CURVE('',#13560,#13561,#8782,.T.);
#17313=EDGE_CURVE('',#13558,#13561,#8783,.T.);
#17314=EDGE_CURVE('',#13561,#13556,#1616,.T.);
#17315=EDGE_CURVE('',#13562,#13563,#8784,.T.);
#17316=EDGE_CURVE('',#13562,#13564,#8785,.T.);
#17317=EDGE_CURVE('',#13565,#13564,#8786,.T.);
#17318=EDGE_CURVE('',#13563,#13565,#8787,.T.);
#17319=EDGE_CURVE('',#13563,#13566,#1617,.T.);
#17320=EDGE_CURVE('',#13565,#13566,#8788,.T.);
#17321=EDGE_CURVE('',#13566,#13567,#8789,.T.);
#17322=EDGE_CURVE('',#13564,#13567,#8790,.T.);
#17323=EDGE_CURVE('',#13567,#13562,#1618,.T.);
#17324=EDGE_CURVE('',#13568,#13569,#8791,.T.);
#17325=EDGE_CURVE('',#13568,#13570,#8792,.T.);
#17326=EDGE_CURVE('',#13571,#13570,#8793,.T.);
#17327=EDGE_CURVE('',#13569,#13571,#8794,.T.);
#17328=EDGE_CURVE('',#13569,#13572,#1619,.T.);
#17329=EDGE_CURVE('',#13571,#13572,#8795,.T.);
#17330=EDGE_CURVE('',#13572,#13573,#8796,.T.);
#17331=EDGE_CURVE('',#13570,#13573,#8797,.T.);
#17332=EDGE_CURVE('',#13573,#13568,#1620,.T.);
#17333=EDGE_CURVE('',#13574,#13575,#8798,.T.);
#17334=EDGE_CURVE('',#13574,#13576,#8799,.T.);
#17335=EDGE_CURVE('',#13577,#13576,#8800,.T.);
#17336=EDGE_CURVE('',#13575,#13577,#8801,.T.);
#17337=EDGE_CURVE('',#13575,#13578,#1621,.T.);
#17338=EDGE_CURVE('',#13577,#13578,#8802,.T.);
#17339=EDGE_CURVE('',#13578,#13579,#8803,.T.);
#17340=EDGE_CURVE('',#13576,#13579,#8804,.T.);
#17341=EDGE_CURVE('',#13579,#13574,#1622,.T.);
#17342=EDGE_CURVE('',#13580,#13581,#8805,.T.);
#17343=EDGE_CURVE('',#13580,#13582,#8806,.T.);
#17344=EDGE_CURVE('',#13583,#13582,#8807,.T.);
#17345=EDGE_CURVE('',#13581,#13583,#8808,.T.);
#17346=EDGE_CURVE('',#13581,#13584,#1623,.T.);
#17347=EDGE_CURVE('',#13583,#13584,#8809,.T.);
#17348=EDGE_CURVE('',#13584,#13585,#8810,.T.);
#17349=EDGE_CURVE('',#13582,#13585,#8811,.T.);
#17350=EDGE_CURVE('',#13585,#13580,#1624,.T.);
#17351=EDGE_CURVE('',#13586,#13587,#8812,.T.);
#17352=EDGE_CURVE('',#13586,#13588,#8813,.T.);
#17353=EDGE_CURVE('',#13589,#13588,#8814,.T.);
#17354=EDGE_CURVE('',#13587,#13589,#8815,.T.);
#17355=EDGE_CURVE('',#13587,#13590,#1625,.T.);
#17356=EDGE_CURVE('',#13589,#13590,#8816,.T.);
#17357=EDGE_CURVE('',#13590,#13591,#8817,.T.);
#17358=EDGE_CURVE('',#13588,#13591,#8818,.T.);
#17359=EDGE_CURVE('',#13591,#13586,#1626,.T.);
#17360=EDGE_CURVE('',#13592,#13593,#8819,.T.);
#17361=EDGE_CURVE('',#13593,#13593,#1627,.T.);
#17362=EDGE_CURVE('',#13594,#13595,#8820,.T.);
#17363=EDGE_CURVE('',#13594,#13596,#8821,.T.);
#17364=EDGE_CURVE('',#13596,#13597,#8822,.T.);
#17365=EDGE_CURVE('',#13595,#13597,#8823,.T.);
#17366=EDGE_CURVE('',#13598,#13594,#8824,.T.);
#17367=EDGE_CURVE('',#13598,#13599,#8825,.T.);
#17368=EDGE_CURVE('',#13599,#13596,#8826,.T.);
#17369=EDGE_CURVE('',#13600,#13598,#8827,.T.);
#17370=EDGE_CURVE('',#13600,#13601,#8828,.T.);
#17371=EDGE_CURVE('',#13601,#13599,#8829,.T.);
#17372=EDGE_CURVE('',#13602,#13600,#8830,.T.);
#17373=EDGE_CURVE('',#13602,#13603,#8831,.T.);
#17374=EDGE_CURVE('',#13603,#13601,#8832,.T.);
#17375=EDGE_CURVE('',#13604,#13602,#8833,.T.);
#17376=EDGE_CURVE('',#13604,#13605,#8834,.T.);
#17377=EDGE_CURVE('',#13605,#13603,#8835,.T.);
#17378=EDGE_CURVE('',#13595,#13604,#8836,.T.);
#17379=EDGE_CURVE('',#13597,#13605,#8837,.T.);
#17380=EDGE_CURVE('',#13606,#13606,#1628,.T.);
#17381=EDGE_CURVE('',#13369,#13606,#8838,.T.);
#17382=EDGE_CURVE('',#13607,#13607,#1629,.T.);
#17383=EDGE_CURVE('',#13607,#13483,#8839,.T.);
#17384=EDGE_CURVE('',#13480,#13373,#8840,.T.);
#17385=EDGE_CURVE('',#13608,#13608,#1630,.T.);
#17386=EDGE_CURVE('',#13608,#13607,#8841,.T.);
#23083=ORIENTED_EDGE('',*,*,#16763,.F.);
#23084=ORIENTED_EDGE('',*,*,#16764,.T.);
#23085=ORIENTED_EDGE('',*,*,#16765,.T.);
#23086=ORIENTED_EDGE('',*,*,#16766,.T.);
#23087=ORIENTED_EDGE('',*,*,#16767,.F.);
#23088=ORIENTED_EDGE('',*,*,#16768,.T.);
#23089=ORIENTED_EDGE('',*,*,#16763,.T.);
#23090=ORIENTED_EDGE('',*,*,#16769,.T.);
#23091=ORIENTED_EDGE('',*,*,#16770,.F.);
#23092=ORIENTED_EDGE('',*,*,#16771,.T.);
#23093=ORIENTED_EDGE('',*,*,#16767,.T.);
#23094=ORIENTED_EDGE('',*,*,#16772,.T.);
#23095=ORIENTED_EDGE('',*,*,#16773,.F.);
#23096=ORIENTED_EDGE('',*,*,#16774,.T.);
#23097=ORIENTED_EDGE('',*,*,#16770,.T.);
#23098=ORIENTED_EDGE('',*,*,#16775,.T.);
#23099=ORIENTED_EDGE('',*,*,#16776,.F.);
#23100=ORIENTED_EDGE('',*,*,#16777,.T.);
#23101=ORIENTED_EDGE('',*,*,#16773,.T.);
#23102=ORIENTED_EDGE('',*,*,#16778,.T.);
#23103=ORIENTED_EDGE('',*,*,#16779,.F.);
#23104=ORIENTED_EDGE('',*,*,#16780,.T.);
#23105=ORIENTED_EDGE('',*,*,#16776,.T.);
#23106=ORIENTED_EDGE('',*,*,#16781,.T.);
#23107=ORIENTED_EDGE('',*,*,#16782,.F.);
#23108=ORIENTED_EDGE('',*,*,#16783,.T.);
#23109=ORIENTED_EDGE('',*,*,#16779,.T.);
#23110=ORIENTED_EDGE('',*,*,#16784,.T.);
#23111=ORIENTED_EDGE('',*,*,#16785,.F.);
#23112=ORIENTED_EDGE('',*,*,#16786,.T.);
#23113=ORIENTED_EDGE('',*,*,#16782,.T.);
#23114=ORIENTED_EDGE('',*,*,#16787,.T.);
#23115=ORIENTED_EDGE('',*,*,#16788,.F.);
#23116=ORIENTED_EDGE('',*,*,#16789,.T.);
#23117=ORIENTED_EDGE('',*,*,#16785,.T.);
#23118=ORIENTED_EDGE('',*,*,#16790,.T.);
#23119=ORIENTED_EDGE('',*,*,#16791,.F.);
#23120=ORIENTED_EDGE('',*,*,#16792,.T.);
#23121=ORIENTED_EDGE('',*,*,#16788,.T.);
#23122=ORIENTED_EDGE('',*,*,#16793,.T.);
#23123=ORIENTED_EDGE('',*,*,#16794,.F.);
#23124=ORIENTED_EDGE('',*,*,#16795,.T.);
#23125=ORIENTED_EDGE('',*,*,#16791,.T.);
#23126=ORIENTED_EDGE('',*,*,#16796,.T.);
#23127=ORIENTED_EDGE('',*,*,#16797,.F.);
#23128=ORIENTED_EDGE('',*,*,#16798,.T.);
#23129=ORIENTED_EDGE('',*,*,#16794,.T.);
#23130=ORIENTED_EDGE('',*,*,#16799,.T.);
#23131=ORIENTED_EDGE('',*,*,#16800,.F.);
#23132=ORIENTED_EDGE('',*,*,#16801,.T.);
#23133=ORIENTED_EDGE('',*,*,#16797,.T.);
#23134=ORIENTED_EDGE('',*,*,#16802,.T.);
#23135=ORIENTED_EDGE('',*,*,#16803,.F.);
#23136=ORIENTED_EDGE('',*,*,#16804,.T.);
#23137=ORIENTED_EDGE('',*,*,#16800,.T.);
#23138=ORIENTED_EDGE('',*,*,#16805,.T.);
#23139=ORIENTED_EDGE('',*,*,#16806,.F.);
#23140=ORIENTED_EDGE('',*,*,#16807,.T.);
#23141=ORIENTED_EDGE('',*,*,#16803,.T.);
#23142=ORIENTED_EDGE('',*,*,#16808,.T.);
#23143=ORIENTED_EDGE('',*,*,#16809,.F.);
#23144=ORIENTED_EDGE('',*,*,#16810,.T.);
#23145=ORIENTED_EDGE('',*,*,#16806,.T.);
#23146=ORIENTED_EDGE('',*,*,#16811,.T.);
#23147=ORIENTED_EDGE('',*,*,#16812,.F.);
#23148=ORIENTED_EDGE('',*,*,#16813,.T.);
#23149=ORIENTED_EDGE('',*,*,#16809,.T.);
#23150=ORIENTED_EDGE('',*,*,#16814,.T.);
#23151=ORIENTED_EDGE('',*,*,#16815,.F.);
#23152=ORIENTED_EDGE('',*,*,#16816,.T.);
#23153=ORIENTED_EDGE('',*,*,#16812,.T.);
#23154=ORIENTED_EDGE('',*,*,#16817,.T.);
#23155=ORIENTED_EDGE('',*,*,#16818,.F.);
#23156=ORIENTED_EDGE('',*,*,#16819,.T.);
#23157=ORIENTED_EDGE('',*,*,#16815,.T.);
#23158=ORIENTED_EDGE('',*,*,#16820,.T.);
#23159=ORIENTED_EDGE('',*,*,#16821,.F.);
#23160=ORIENTED_EDGE('',*,*,#16822,.T.);
#23161=ORIENTED_EDGE('',*,*,#16818,.T.);
#23162=ORIENTED_EDGE('',*,*,#16823,.T.);
#23163=ORIENTED_EDGE('',*,*,#16824,.F.);
#23164=ORIENTED_EDGE('',*,*,#16825,.T.);
#23165=ORIENTED_EDGE('',*,*,#16821,.T.);
#23166=ORIENTED_EDGE('',*,*,#16826,.T.);
#23167=ORIENTED_EDGE('',*,*,#16827,.F.);
#23168=ORIENTED_EDGE('',*,*,#16828,.T.);
#23169=ORIENTED_EDGE('',*,*,#16824,.T.);
#23170=ORIENTED_EDGE('',*,*,#16829,.T.);
#23171=ORIENTED_EDGE('',*,*,#16830,.F.);
#23172=ORIENTED_EDGE('',*,*,#16831,.T.);
#23173=ORIENTED_EDGE('',*,*,#16827,.T.);
#23174=ORIENTED_EDGE('',*,*,#16832,.T.);
#23175=ORIENTED_EDGE('',*,*,#16833,.F.);
#23176=ORIENTED_EDGE('',*,*,#16834,.T.);
#23177=ORIENTED_EDGE('',*,*,#16830,.T.);
#23178=ORIENTED_EDGE('',*,*,#16835,.T.);
#23179=ORIENTED_EDGE('',*,*,#16836,.F.);
#23180=ORIENTED_EDGE('',*,*,#16837,.T.);
#23181=ORIENTED_EDGE('',*,*,#16833,.T.);
#23182=ORIENTED_EDGE('',*,*,#16838,.T.);
#23183=ORIENTED_EDGE('',*,*,#16839,.F.);
#23184=ORIENTED_EDGE('',*,*,#16840,.T.);
#23185=ORIENTED_EDGE('',*,*,#16836,.T.);
#23186=ORIENTED_EDGE('',*,*,#16841,.T.);
#23187=ORIENTED_EDGE('',*,*,#16842,.F.);
#23188=ORIENTED_EDGE('',*,*,#16843,.T.);
#23189=ORIENTED_EDGE('',*,*,#16839,.T.);
#23190=ORIENTED_EDGE('',*,*,#16844,.T.);
#23191=ORIENTED_EDGE('',*,*,#16845,.F.);
#23192=ORIENTED_EDGE('',*,*,#16846,.T.);
#23193=ORIENTED_EDGE('',*,*,#16842,.T.);
#23194=ORIENTED_EDGE('',*,*,#16847,.T.);
#23195=ORIENTED_EDGE('',*,*,#16848,.F.);
#23196=ORIENTED_EDGE('',*,*,#16849,.T.);
#23197=ORIENTED_EDGE('',*,*,#16845,.T.);
#23198=ORIENTED_EDGE('',*,*,#16850,.T.);
#23199=ORIENTED_EDGE('',*,*,#16851,.F.);
#23200=ORIENTED_EDGE('',*,*,#16852,.T.);
#23201=ORIENTED_EDGE('',*,*,#16848,.T.);
#23202=ORIENTED_EDGE('',*,*,#16853,.T.);
#23203=ORIENTED_EDGE('',*,*,#16854,.F.);
#23204=ORIENTED_EDGE('',*,*,#16855,.T.);
#23205=ORIENTED_EDGE('',*,*,#16851,.T.);
#23206=ORIENTED_EDGE('',*,*,#16856,.T.);
#23207=ORIENTED_EDGE('',*,*,#16857,.F.);
#23208=ORIENTED_EDGE('',*,*,#16858,.T.);
#23209=ORIENTED_EDGE('',*,*,#16854,.T.);
#23210=ORIENTED_EDGE('',*,*,#16859,.T.);
#23211=ORIENTED_EDGE('',*,*,#16860,.F.);
#23212=ORIENTED_EDGE('',*,*,#16861,.T.);
#23213=ORIENTED_EDGE('',*,*,#16857,.T.);
#23214=ORIENTED_EDGE('',*,*,#16862,.T.);
#23215=ORIENTED_EDGE('',*,*,#16863,.F.);
#23216=ORIENTED_EDGE('',*,*,#16864,.T.);
#23217=ORIENTED_EDGE('',*,*,#16860,.T.);
#23218=ORIENTED_EDGE('',*,*,#16865,.T.);
#23219=ORIENTED_EDGE('',*,*,#16866,.F.);
#23220=ORIENTED_EDGE('',*,*,#16867,.T.);
#23221=ORIENTED_EDGE('',*,*,#16863,.T.);
#23222=ORIENTED_EDGE('',*,*,#16868,.T.);
#23223=ORIENTED_EDGE('',*,*,#16869,.F.);
#23224=ORIENTED_EDGE('',*,*,#16870,.T.);
#23225=ORIENTED_EDGE('',*,*,#16866,.T.);
#23226=ORIENTED_EDGE('',*,*,#16871,.T.);
#23227=ORIENTED_EDGE('',*,*,#16872,.F.);
#23228=ORIENTED_EDGE('',*,*,#16873,.T.);
#23229=ORIENTED_EDGE('',*,*,#16869,.T.);
#23230=ORIENTED_EDGE('',*,*,#16874,.T.);
#23231=ORIENTED_EDGE('',*,*,#16875,.F.);
#23232=ORIENTED_EDGE('',*,*,#16876,.T.);
#23233=ORIENTED_EDGE('',*,*,#16872,.T.);
#23234=ORIENTED_EDGE('',*,*,#16877,.T.);
#23235=ORIENTED_EDGE('',*,*,#16878,.F.);
#23236=ORIENTED_EDGE('',*,*,#16879,.T.);
#23237=ORIENTED_EDGE('',*,*,#16875,.T.);
#23238=ORIENTED_EDGE('',*,*,#16880,.T.);
#23239=ORIENTED_EDGE('',*,*,#16881,.F.);
#23240=ORIENTED_EDGE('',*,*,#16882,.T.);
#23241=ORIENTED_EDGE('',*,*,#16878,.T.);
#23242=ORIENTED_EDGE('',*,*,#16883,.T.);
#23243=ORIENTED_EDGE('',*,*,#16884,.F.);
#23244=ORIENTED_EDGE('',*,*,#16885,.T.);
#23245=ORIENTED_EDGE('',*,*,#16881,.T.);
#23246=ORIENTED_EDGE('',*,*,#16886,.T.);
#23247=ORIENTED_EDGE('',*,*,#16887,.F.);
#23248=ORIENTED_EDGE('',*,*,#16888,.T.);
#23249=ORIENTED_EDGE('',*,*,#16884,.T.);
#23250=ORIENTED_EDGE('',*,*,#16889,.T.);
#23251=ORIENTED_EDGE('',*,*,#16890,.F.);
#23252=ORIENTED_EDGE('',*,*,#16891,.T.);
#23253=ORIENTED_EDGE('',*,*,#16892,.F.);
#23254=ORIENTED_EDGE('',*,*,#16893,.F.);
#23255=ORIENTED_EDGE('',*,*,#16894,.F.);
#23256=ORIENTED_EDGE('',*,*,#16895,.T.);
#23257=ORIENTED_EDGE('',*,*,#16890,.T.);
#23258=ORIENTED_EDGE('',*,*,#16896,.F.);
#23259=ORIENTED_EDGE('',*,*,#16897,.F.);
#23260=ORIENTED_EDGE('',*,*,#16898,.T.);
#23261=ORIENTED_EDGE('',*,*,#16894,.T.);
#23262=ORIENTED_EDGE('',*,*,#16899,.F.);
#23263=ORIENTED_EDGE('',*,*,#16900,.F.);
#23264=ORIENTED_EDGE('',*,*,#16901,.T.);
#23265=ORIENTED_EDGE('',*,*,#16897,.T.);
#23266=ORIENTED_EDGE('',*,*,#16902,.F.);
#23267=ORIENTED_EDGE('',*,*,#16903,.F.);
#23268=ORIENTED_EDGE('',*,*,#16904,.T.);
#23269=ORIENTED_EDGE('',*,*,#16900,.T.);
#23270=ORIENTED_EDGE('',*,*,#16905,.F.);
#23271=ORIENTED_EDGE('',*,*,#16906,.F.);
#23272=ORIENTED_EDGE('',*,*,#16907,.T.);
#23273=ORIENTED_EDGE('',*,*,#16903,.T.);
#23274=ORIENTED_EDGE('',*,*,#16908,.F.);
#23275=ORIENTED_EDGE('',*,*,#16909,.F.);
#23276=ORIENTED_EDGE('',*,*,#16910,.T.);
#23277=ORIENTED_EDGE('',*,*,#16906,.T.);
#23278=ORIENTED_EDGE('',*,*,#16911,.F.);
#23279=ORIENTED_EDGE('',*,*,#16912,.F.);
#23280=ORIENTED_EDGE('',*,*,#16913,.T.);
#23281=ORIENTED_EDGE('',*,*,#16909,.T.);
#23282=ORIENTED_EDGE('',*,*,#16914,.F.);
#23283=ORIENTED_EDGE('',*,*,#16915,.F.);
#23284=ORIENTED_EDGE('',*,*,#16916,.T.);
#23285=ORIENTED_EDGE('',*,*,#16912,.T.);
#23286=ORIENTED_EDGE('',*,*,#16917,.F.);
#23287=ORIENTED_EDGE('',*,*,#16918,.F.);
#23288=ORIENTED_EDGE('',*,*,#16919,.T.);
#23289=ORIENTED_EDGE('',*,*,#16915,.T.);
#23290=ORIENTED_EDGE('',*,*,#16920,.F.);
#23291=ORIENTED_EDGE('',*,*,#16921,.F.);
#23292=ORIENTED_EDGE('',*,*,#16922,.T.);
#23293=ORIENTED_EDGE('',*,*,#16918,.T.);
#23294=ORIENTED_EDGE('',*,*,#16923,.F.);
#23295=ORIENTED_EDGE('',*,*,#16924,.F.);
#23296=ORIENTED_EDGE('',*,*,#16925,.T.);
#23297=ORIENTED_EDGE('',*,*,#16921,.T.);
#23298=ORIENTED_EDGE('',*,*,#16926,.F.);
#23299=ORIENTED_EDGE('',*,*,#16927,.F.);
#23300=ORIENTED_EDGE('',*,*,#16928,.T.);
#23301=ORIENTED_EDGE('',*,*,#16924,.T.);
#23302=ORIENTED_EDGE('',*,*,#16929,.F.);
#23303=ORIENTED_EDGE('',*,*,#16930,.F.);
#23304=ORIENTED_EDGE('',*,*,#16931,.T.);
#23305=ORIENTED_EDGE('',*,*,#16927,.T.);
#23306=ORIENTED_EDGE('',*,*,#16932,.F.);
#23307=ORIENTED_EDGE('',*,*,#16933,.F.);
#23308=ORIENTED_EDGE('',*,*,#16934,.T.);
#23309=ORIENTED_EDGE('',*,*,#16930,.T.);
#23310=ORIENTED_EDGE('',*,*,#16935,.F.);
#23311=ORIENTED_EDGE('',*,*,#16936,.F.);
#23312=ORIENTED_EDGE('',*,*,#16937,.T.);
#23313=ORIENTED_EDGE('',*,*,#16933,.T.);
#23314=ORIENTED_EDGE('',*,*,#16938,.F.);
#23315=ORIENTED_EDGE('',*,*,#16939,.F.);
#23316=ORIENTED_EDGE('',*,*,#16940,.T.);
#23317=ORIENTED_EDGE('',*,*,#16936,.T.);
#23318=ORIENTED_EDGE('',*,*,#16941,.F.);
#23319=ORIENTED_EDGE('',*,*,#16942,.F.);
#23320=ORIENTED_EDGE('',*,*,#16943,.T.);
#23321=ORIENTED_EDGE('',*,*,#16939,.T.);
#23322=ORIENTED_EDGE('',*,*,#16944,.F.);
#23323=ORIENTED_EDGE('',*,*,#16945,.F.);
#23324=ORIENTED_EDGE('',*,*,#16946,.T.);
#23325=ORIENTED_EDGE('',*,*,#16942,.T.);
#23326=ORIENTED_EDGE('',*,*,#16947,.F.);
#23327=ORIENTED_EDGE('',*,*,#16948,.F.);
#23328=ORIENTED_EDGE('',*,*,#16949,.T.);
#23329=ORIENTED_EDGE('',*,*,#16945,.T.);
#23330=ORIENTED_EDGE('',*,*,#16950,.F.);
#23331=ORIENTED_EDGE('',*,*,#16951,.F.);
#23332=ORIENTED_EDGE('',*,*,#16952,.T.);
#23333=ORIENTED_EDGE('',*,*,#16948,.T.);
#23334=ORIENTED_EDGE('',*,*,#16953,.F.);
#23335=ORIENTED_EDGE('',*,*,#16954,.F.);
#23336=ORIENTED_EDGE('',*,*,#16955,.T.);
#23337=ORIENTED_EDGE('',*,*,#16951,.T.);
#23338=ORIENTED_EDGE('',*,*,#16956,.F.);
#23339=ORIENTED_EDGE('',*,*,#16957,.F.);
#23340=ORIENTED_EDGE('',*,*,#16958,.T.);
#23341=ORIENTED_EDGE('',*,*,#16954,.T.);
#23342=ORIENTED_EDGE('',*,*,#16959,.F.);
#23343=ORIENTED_EDGE('',*,*,#16960,.F.);
#23344=ORIENTED_EDGE('',*,*,#16961,.T.);
#23345=ORIENTED_EDGE('',*,*,#16957,.T.);
#23346=ORIENTED_EDGE('',*,*,#16962,.F.);
#23347=ORIENTED_EDGE('',*,*,#16963,.F.);
#23348=ORIENTED_EDGE('',*,*,#16964,.T.);
#23349=ORIENTED_EDGE('',*,*,#16960,.T.);
#23350=ORIENTED_EDGE('',*,*,#16965,.F.);
#23351=ORIENTED_EDGE('',*,*,#16966,.F.);
#23352=ORIENTED_EDGE('',*,*,#16967,.T.);
#23353=ORIENTED_EDGE('',*,*,#16963,.T.);
#23354=ORIENTED_EDGE('',*,*,#16968,.F.);
#23355=ORIENTED_EDGE('',*,*,#16969,.F.);
#23356=ORIENTED_EDGE('',*,*,#16970,.T.);
#23357=ORIENTED_EDGE('',*,*,#16966,.T.);
#23358=ORIENTED_EDGE('',*,*,#16971,.F.);
#23359=ORIENTED_EDGE('',*,*,#16972,.F.);
#23360=ORIENTED_EDGE('',*,*,#16973,.T.);
#23361=ORIENTED_EDGE('',*,*,#16969,.T.);
#23362=ORIENTED_EDGE('',*,*,#16974,.F.);
#23363=ORIENTED_EDGE('',*,*,#16975,.F.);
#23364=ORIENTED_EDGE('',*,*,#16976,.T.);
#23365=ORIENTED_EDGE('',*,*,#16972,.T.);
#23366=ORIENTED_EDGE('',*,*,#16977,.F.);
#23367=ORIENTED_EDGE('',*,*,#16978,.F.);
#23368=ORIENTED_EDGE('',*,*,#16979,.T.);
#23369=ORIENTED_EDGE('',*,*,#16975,.T.);
#23370=ORIENTED_EDGE('',*,*,#16980,.F.);
#23371=ORIENTED_EDGE('',*,*,#16981,.F.);
#23372=ORIENTED_EDGE('',*,*,#16982,.T.);
#23373=ORIENTED_EDGE('',*,*,#16978,.T.);
#23374=ORIENTED_EDGE('',*,*,#16983,.F.);
#23375=ORIENTED_EDGE('',*,*,#16984,.F.);
#23376=ORIENTED_EDGE('',*,*,#16985,.T.);
#23377=ORIENTED_EDGE('',*,*,#16981,.T.);
#23378=ORIENTED_EDGE('',*,*,#16986,.F.);
#23379=ORIENTED_EDGE('',*,*,#16987,.F.);
#23380=ORIENTED_EDGE('',*,*,#16988,.T.);
#23381=ORIENTED_EDGE('',*,*,#16984,.T.);
#23382=ORIENTED_EDGE('',*,*,#16989,.F.);
#23383=ORIENTED_EDGE('',*,*,#16990,.F.);
#23384=ORIENTED_EDGE('',*,*,#16991,.T.);
#23385=ORIENTED_EDGE('',*,*,#16987,.T.);
#23386=ORIENTED_EDGE('',*,*,#16992,.F.);
#23387=ORIENTED_EDGE('',*,*,#16993,.F.);
#23388=ORIENTED_EDGE('',*,*,#16994,.T.);
#23389=ORIENTED_EDGE('',*,*,#16990,.T.);
#23390=ORIENTED_EDGE('',*,*,#16995,.F.);
#23391=ORIENTED_EDGE('',*,*,#16996,.F.);
#23392=ORIENTED_EDGE('',*,*,#16997,.T.);
#23393=ORIENTED_EDGE('',*,*,#16993,.T.);
#23394=ORIENTED_EDGE('',*,*,#16998,.F.);
#23395=ORIENTED_EDGE('',*,*,#16999,.F.);
#23396=ORIENTED_EDGE('',*,*,#17000,.T.);
#23397=ORIENTED_EDGE('',*,*,#16996,.T.);
#23398=ORIENTED_EDGE('',*,*,#17001,.F.);
#23399=ORIENTED_EDGE('',*,*,#17002,.F.);
#23400=ORIENTED_EDGE('',*,*,#17003,.T.);
#23401=ORIENTED_EDGE('',*,*,#16999,.T.);
#23402=ORIENTED_EDGE('',*,*,#17004,.F.);
#23403=ORIENTED_EDGE('',*,*,#17005,.F.);
#23404=ORIENTED_EDGE('',*,*,#17006,.T.);
#23405=ORIENTED_EDGE('',*,*,#17002,.T.);
#23406=ORIENTED_EDGE('',*,*,#17007,.F.);
#23407=ORIENTED_EDGE('',*,*,#17008,.F.);
#23408=ORIENTED_EDGE('',*,*,#17009,.T.);
#23409=ORIENTED_EDGE('',*,*,#17005,.T.);
#23410=ORIENTED_EDGE('',*,*,#17010,.F.);
#23411=ORIENTED_EDGE('',*,*,#17011,.F.);
#23412=ORIENTED_EDGE('',*,*,#17012,.T.);
#23413=ORIENTED_EDGE('',*,*,#17008,.T.);
#23414=ORIENTED_EDGE('',*,*,#17013,.F.);
#23415=ORIENTED_EDGE('',*,*,#17014,.F.);
#23416=ORIENTED_EDGE('',*,*,#17015,.T.);
#23417=ORIENTED_EDGE('',*,*,#17011,.T.);
#23418=ORIENTED_EDGE('',*,*,#17016,.F.);
#23419=ORIENTED_EDGE('',*,*,#16892,.T.);
#23420=ORIENTED_EDGE('',*,*,#17017,.T.);
#23421=ORIENTED_EDGE('',*,*,#17018,.F.);
#23422=ORIENTED_EDGE('',*,*,#17019,.T.);
#23423=ORIENTED_EDGE('',*,*,#17019,.F.);
#23424=ORIENTED_EDGE('',*,*,#17020,.F.);
#23425=ORIENTED_EDGE('',*,*,#16889,.F.);
#23426=ORIENTED_EDGE('',*,*,#16886,.F.);
#23427=ORIENTED_EDGE('',*,*,#16883,.F.);
#23428=ORIENTED_EDGE('',*,*,#16880,.F.);
#23429=ORIENTED_EDGE('',*,*,#16877,.F.);
#23430=ORIENTED_EDGE('',*,*,#16874,.F.);
#23431=ORIENTED_EDGE('',*,*,#16871,.F.);
#23432=ORIENTED_EDGE('',*,*,#16868,.F.);
#23433=ORIENTED_EDGE('',*,*,#16865,.F.);
#23434=ORIENTED_EDGE('',*,*,#16862,.F.);
#23435=ORIENTED_EDGE('',*,*,#16859,.F.);
#23436=ORIENTED_EDGE('',*,*,#16856,.F.);
#23437=ORIENTED_EDGE('',*,*,#16853,.F.);
#23438=ORIENTED_EDGE('',*,*,#16850,.F.);
#23439=ORIENTED_EDGE('',*,*,#16847,.F.);
#23440=ORIENTED_EDGE('',*,*,#16844,.F.);
#23441=ORIENTED_EDGE('',*,*,#16841,.F.);
#23442=ORIENTED_EDGE('',*,*,#16838,.F.);
#23443=ORIENTED_EDGE('',*,*,#16835,.F.);
#23444=ORIENTED_EDGE('',*,*,#16832,.F.);
#23445=ORIENTED_EDGE('',*,*,#16829,.F.);
#23446=ORIENTED_EDGE('',*,*,#16826,.F.);
#23447=ORIENTED_EDGE('',*,*,#16823,.F.);
#23448=ORIENTED_EDGE('',*,*,#16820,.F.);
#23449=ORIENTED_EDGE('',*,*,#16817,.F.);
#23450=ORIENTED_EDGE('',*,*,#16814,.F.);
#23451=ORIENTED_EDGE('',*,*,#16811,.F.);
#23452=ORIENTED_EDGE('',*,*,#16808,.F.);
#23453=ORIENTED_EDGE('',*,*,#16805,.F.);
#23454=ORIENTED_EDGE('',*,*,#16802,.F.);
#23455=ORIENTED_EDGE('',*,*,#16799,.F.);
#23456=ORIENTED_EDGE('',*,*,#16796,.F.);
#23457=ORIENTED_EDGE('',*,*,#16793,.F.);
#23458=ORIENTED_EDGE('',*,*,#16790,.F.);
#23459=ORIENTED_EDGE('',*,*,#16787,.F.);
#23460=ORIENTED_EDGE('',*,*,#16784,.F.);
#23461=ORIENTED_EDGE('',*,*,#16781,.F.);
#23462=ORIENTED_EDGE('',*,*,#16778,.F.);
#23463=ORIENTED_EDGE('',*,*,#16775,.F.);
#23464=ORIENTED_EDGE('',*,*,#16772,.F.);
#23465=ORIENTED_EDGE('',*,*,#16769,.F.);
#23466=ORIENTED_EDGE('',*,*,#16766,.F.);
#23467=ORIENTED_EDGE('',*,*,#17021,.F.);
#23468=ORIENTED_EDGE('',*,*,#17022,.T.);
#23469=ORIENTED_EDGE('',*,*,#17016,.T.);
#23470=ORIENTED_EDGE('',*,*,#17013,.T.);
#23471=ORIENTED_EDGE('',*,*,#17010,.T.);
#23472=ORIENTED_EDGE('',*,*,#17007,.T.);
#23473=ORIENTED_EDGE('',*,*,#17004,.T.);
#23474=ORIENTED_EDGE('',*,*,#17001,.T.);
#23475=ORIENTED_EDGE('',*,*,#16998,.T.);
#23476=ORIENTED_EDGE('',*,*,#16995,.T.);
#23477=ORIENTED_EDGE('',*,*,#16992,.T.);
#23478=ORIENTED_EDGE('',*,*,#16989,.T.);
#23479=ORIENTED_EDGE('',*,*,#16986,.T.);
#23480=ORIENTED_EDGE('',*,*,#16983,.T.);
#23481=ORIENTED_EDGE('',*,*,#16980,.T.);
#23482=ORIENTED_EDGE('',*,*,#16977,.T.);
#23483=ORIENTED_EDGE('',*,*,#16974,.T.);
#23484=ORIENTED_EDGE('',*,*,#16971,.T.);
#23485=ORIENTED_EDGE('',*,*,#16968,.T.);
#23486=ORIENTED_EDGE('',*,*,#16965,.T.);
#23487=ORIENTED_EDGE('',*,*,#16962,.T.);
#23488=ORIENTED_EDGE('',*,*,#16959,.T.);
#23489=ORIENTED_EDGE('',*,*,#16956,.T.);
#23490=ORIENTED_EDGE('',*,*,#16953,.T.);
#23491=ORIENTED_EDGE('',*,*,#16950,.T.);
#23492=ORIENTED_EDGE('',*,*,#16947,.T.);
#23493=ORIENTED_EDGE('',*,*,#16944,.T.);
#23494=ORIENTED_EDGE('',*,*,#16941,.T.);
#23495=ORIENTED_EDGE('',*,*,#16938,.T.);
#23496=ORIENTED_EDGE('',*,*,#16935,.T.);
#23497=ORIENTED_EDGE('',*,*,#16932,.T.);
#23498=ORIENTED_EDGE('',*,*,#16929,.T.);
#23499=ORIENTED_EDGE('',*,*,#16926,.T.);
#23500=ORIENTED_EDGE('',*,*,#16923,.T.);
#23501=ORIENTED_EDGE('',*,*,#16920,.T.);
#23502=ORIENTED_EDGE('',*,*,#16917,.T.);
#23503=ORIENTED_EDGE('',*,*,#16914,.T.);
#23504=ORIENTED_EDGE('',*,*,#16911,.T.);
#23505=ORIENTED_EDGE('',*,*,#16908,.T.);
#23506=ORIENTED_EDGE('',*,*,#16905,.T.);
#23507=ORIENTED_EDGE('',*,*,#16902,.T.);
#23508=ORIENTED_EDGE('',*,*,#16899,.T.);
#23509=ORIENTED_EDGE('',*,*,#16896,.T.);
#23510=ORIENTED_EDGE('',*,*,#16893,.T.);
#23511=ORIENTED_EDGE('',*,*,#17023,.T.);
#23512=ORIENTED_EDGE('',*,*,#17024,.T.);
#23513=ORIENTED_EDGE('',*,*,#17025,.T.);
#23514=ORIENTED_EDGE('',*,*,#17026,.T.);
#23515=ORIENTED_EDGE('',*,*,#17021,.T.);
#23516=ORIENTED_EDGE('',*,*,#17014,.T.);
#23517=ORIENTED_EDGE('',*,*,#17022,.F.);
#23518=ORIENTED_EDGE('',*,*,#17026,.F.);
#23519=ORIENTED_EDGE('',*,*,#17027,.T.);
#23520=ORIENTED_EDGE('',*,*,#17017,.F.);
#23521=ORIENTED_EDGE('',*,*,#16891,.F.);
#23522=ORIENTED_EDGE('',*,*,#16895,.F.);
#23523=ORIENTED_EDGE('',*,*,#16898,.F.);
#23524=ORIENTED_EDGE('',*,*,#16901,.F.);
#23525=ORIENTED_EDGE('',*,*,#16904,.F.);
#23526=ORIENTED_EDGE('',*,*,#16907,.F.);
#23527=ORIENTED_EDGE('',*,*,#16910,.F.);
#23528=ORIENTED_EDGE('',*,*,#16913,.F.);
#23529=ORIENTED_EDGE('',*,*,#16916,.F.);
#23530=ORIENTED_EDGE('',*,*,#16919,.F.);
#23531=ORIENTED_EDGE('',*,*,#16922,.F.);
#23532=ORIENTED_EDGE('',*,*,#16925,.F.);
#23533=ORIENTED_EDGE('',*,*,#16928,.F.);
#23534=ORIENTED_EDGE('',*,*,#16931,.F.);
#23535=ORIENTED_EDGE('',*,*,#16934,.F.);
#23536=ORIENTED_EDGE('',*,*,#16937,.F.);
#23537=ORIENTED_EDGE('',*,*,#16940,.F.);
#23538=ORIENTED_EDGE('',*,*,#16943,.F.);
#23539=ORIENTED_EDGE('',*,*,#16946,.F.);
#23540=ORIENTED_EDGE('',*,*,#16949,.F.);
#23541=ORIENTED_EDGE('',*,*,#16952,.F.);
#23542=ORIENTED_EDGE('',*,*,#16955,.F.);
#23543=ORIENTED_EDGE('',*,*,#16958,.F.);
#23544=ORIENTED_EDGE('',*,*,#16961,.F.);
#23545=ORIENTED_EDGE('',*,*,#16964,.F.);
#23546=ORIENTED_EDGE('',*,*,#16967,.F.);
#23547=ORIENTED_EDGE('',*,*,#16970,.F.);
#23548=ORIENTED_EDGE('',*,*,#16973,.F.);
#23549=ORIENTED_EDGE('',*,*,#16976,.F.);
#23550=ORIENTED_EDGE('',*,*,#16979,.F.);
#23551=ORIENTED_EDGE('',*,*,#16982,.F.);
#23552=ORIENTED_EDGE('',*,*,#16985,.F.);
#23553=ORIENTED_EDGE('',*,*,#16988,.F.);
#23554=ORIENTED_EDGE('',*,*,#16991,.F.);
#23555=ORIENTED_EDGE('',*,*,#16994,.F.);
#23556=ORIENTED_EDGE('',*,*,#16997,.F.);
#23557=ORIENTED_EDGE('',*,*,#17000,.F.);
#23558=ORIENTED_EDGE('',*,*,#17003,.F.);
#23559=ORIENTED_EDGE('',*,*,#17006,.F.);
#23560=ORIENTED_EDGE('',*,*,#17009,.F.);
#23561=ORIENTED_EDGE('',*,*,#17012,.F.);
#23562=ORIENTED_EDGE('',*,*,#17015,.F.);
#23563=ORIENTED_EDGE('',*,*,#17027,.F.);
#23564=ORIENTED_EDGE('',*,*,#17025,.F.);
#23565=ORIENTED_EDGE('',*,*,#16764,.F.);
#23566=ORIENTED_EDGE('',*,*,#16768,.F.);
#23567=ORIENTED_EDGE('',*,*,#16771,.F.);
#23568=ORIENTED_EDGE('',*,*,#16774,.F.);
#23569=ORIENTED_EDGE('',*,*,#16777,.F.);
#23570=ORIENTED_EDGE('',*,*,#16780,.F.);
#23571=ORIENTED_EDGE('',*,*,#16783,.F.);
#23572=ORIENTED_EDGE('',*,*,#16786,.F.);
#23573=ORIENTED_EDGE('',*,*,#16789,.F.);
#23574=ORIENTED_EDGE('',*,*,#16792,.F.);
#23575=ORIENTED_EDGE('',*,*,#16795,.F.);
#23576=ORIENTED_EDGE('',*,*,#16798,.F.);
#23577=ORIENTED_EDGE('',*,*,#16801,.F.);
#23578=ORIENTED_EDGE('',*,*,#16804,.F.);
#23579=ORIENTED_EDGE('',*,*,#16807,.F.);
#23580=ORIENTED_EDGE('',*,*,#16810,.F.);
#23581=ORIENTED_EDGE('',*,*,#16813,.F.);
#23582=ORIENTED_EDGE('',*,*,#16816,.F.);
#23583=ORIENTED_EDGE('',*,*,#16819,.F.);
#23584=ORIENTED_EDGE('',*,*,#16822,.F.);
#23585=ORIENTED_EDGE('',*,*,#16825,.F.);
#23586=ORIENTED_EDGE('',*,*,#16828,.F.);
#23587=ORIENTED_EDGE('',*,*,#16831,.F.);
#23588=ORIENTED_EDGE('',*,*,#16834,.F.);
#23589=ORIENTED_EDGE('',*,*,#16837,.F.);
#23590=ORIENTED_EDGE('',*,*,#16840,.F.);
#23591=ORIENTED_EDGE('',*,*,#16843,.F.);
#23592=ORIENTED_EDGE('',*,*,#16846,.F.);
#23593=ORIENTED_EDGE('',*,*,#16849,.F.);
#23594=ORIENTED_EDGE('',*,*,#16852,.F.);
#23595=ORIENTED_EDGE('',*,*,#16855,.F.);
#23596=ORIENTED_EDGE('',*,*,#16858,.F.);
#23597=ORIENTED_EDGE('',*,*,#16861,.F.);
#23598=ORIENTED_EDGE('',*,*,#16864,.F.);
#23599=ORIENTED_EDGE('',*,*,#16867,.F.);
#23600=ORIENTED_EDGE('',*,*,#16870,.F.);
#23601=ORIENTED_EDGE('',*,*,#16873,.F.);
#23602=ORIENTED_EDGE('',*,*,#16876,.F.);
#23603=ORIENTED_EDGE('',*,*,#16879,.F.);
#23604=ORIENTED_EDGE('',*,*,#16882,.F.);
#23605=ORIENTED_EDGE('',*,*,#16885,.F.);
#23606=ORIENTED_EDGE('',*,*,#16888,.F.);
#23607=ORIENTED_EDGE('',*,*,#17028,.F.);
#23608=ORIENTED_EDGE('',*,*,#17018,.T.);
#23609=ORIENTED_EDGE('',*,*,#17029,.T.);
#23610=ORIENTED_EDGE('',*,*,#17030,.T.);
#23611=ORIENTED_EDGE('',*,*,#17031,.T.);
#23612=ORIENTED_EDGE('',*,*,#17030,.F.);
#23613=ORIENTED_EDGE('',*,*,#17032,.T.);
#23614=ORIENTED_EDGE('',*,*,#16887,.T.);
#23615=ORIENTED_EDGE('',*,*,#17020,.T.);
#23616=ORIENTED_EDGE('',*,*,#17032,.F.);
#23617=ORIENTED_EDGE('',*,*,#17029,.F.);
#23618=ORIENTED_EDGE('',*,*,#17028,.T.);
#23619=ORIENTED_EDGE('',*,*,#17033,.F.);
#23620=ORIENTED_EDGE('',*,*,#17031,.F.);
#23621=ORIENTED_EDGE('',*,*,#17034,.F.);
#23622=ORIENTED_EDGE('',*,*,#17035,.T.);
#23623=ORIENTED_EDGE('',*,*,#17036,.F.);
#23624=ORIENTED_EDGE('',*,*,#17037,.F.);
#23625=ORIENTED_EDGE('',*,*,#17038,.F.);
#23626=ORIENTED_EDGE('',*,*,#17037,.T.);
#23627=ORIENTED_EDGE('',*,*,#17039,.T.);
#23628=ORIENTED_EDGE('',*,*,#17040,.F.);
#23629=ORIENTED_EDGE('',*,*,#17039,.F.);
#23630=ORIENTED_EDGE('',*,*,#17036,.T.);
#23631=ORIENTED_EDGE('',*,*,#17041,.T.);
#23632=ORIENTED_EDGE('',*,*,#17042,.F.);
#23633=ORIENTED_EDGE('',*,*,#17041,.F.);
#23634=ORIENTED_EDGE('',*,*,#17035,.F.);
#23635=ORIENTED_EDGE('',*,*,#17043,.F.);
#23636=ORIENTED_EDGE('',*,*,#17044,.T.);
#23637=ORIENTED_EDGE('',*,*,#17045,.F.);
#23638=ORIENTED_EDGE('',*,*,#17046,.F.);
#23639=ORIENTED_EDGE('',*,*,#17047,.F.);
#23640=ORIENTED_EDGE('',*,*,#17046,.T.);
#23641=ORIENTED_EDGE('',*,*,#17048,.T.);
#23642=ORIENTED_EDGE('',*,*,#17049,.F.);
#23643=ORIENTED_EDGE('',*,*,#17048,.F.);
#23644=ORIENTED_EDGE('',*,*,#17045,.T.);
#23645=ORIENTED_EDGE('',*,*,#17050,.T.);
#23646=ORIENTED_EDGE('',*,*,#17051,.F.);
#23647=ORIENTED_EDGE('',*,*,#17050,.F.);
#23648=ORIENTED_EDGE('',*,*,#17044,.F.);
#23649=ORIENTED_EDGE('',*,*,#17052,.F.);
#23650=ORIENTED_EDGE('',*,*,#17053,.T.);
#23651=ORIENTED_EDGE('',*,*,#17054,.F.);
#23652=ORIENTED_EDGE('',*,*,#17055,.F.);
#23653=ORIENTED_EDGE('',*,*,#17056,.F.);
#23654=ORIENTED_EDGE('',*,*,#17055,.T.);
#23655=ORIENTED_EDGE('',*,*,#17057,.T.);
#23656=ORIENTED_EDGE('',*,*,#17058,.F.);
#23657=ORIENTED_EDGE('',*,*,#17057,.F.);
#23658=ORIENTED_EDGE('',*,*,#17054,.T.);
#23659=ORIENTED_EDGE('',*,*,#17059,.T.);
#23660=ORIENTED_EDGE('',*,*,#17060,.F.);
#23661=ORIENTED_EDGE('',*,*,#17059,.F.);
#23662=ORIENTED_EDGE('',*,*,#17053,.F.);
#23663=ORIENTED_EDGE('',*,*,#17061,.F.);
#23664=ORIENTED_EDGE('',*,*,#17062,.T.);
#23665=ORIENTED_EDGE('',*,*,#17063,.F.);
#23666=ORIENTED_EDGE('',*,*,#17064,.F.);
#23667=ORIENTED_EDGE('',*,*,#17065,.F.);
#23668=ORIENTED_EDGE('',*,*,#17064,.T.);
#23669=ORIENTED_EDGE('',*,*,#17066,.T.);
#23670=ORIENTED_EDGE('',*,*,#17067,.F.);
#23671=ORIENTED_EDGE('',*,*,#17066,.F.);
#23672=ORIENTED_EDGE('',*,*,#17063,.T.);
#23673=ORIENTED_EDGE('',*,*,#17068,.T.);
#23674=ORIENTED_EDGE('',*,*,#17069,.F.);
#23675=ORIENTED_EDGE('',*,*,#17068,.F.);
#23676=ORIENTED_EDGE('',*,*,#17062,.F.);
#23677=ORIENTED_EDGE('',*,*,#17070,.F.);
#23678=ORIENTED_EDGE('',*,*,#17071,.T.);
#23679=ORIENTED_EDGE('',*,*,#17072,.F.);
#23680=ORIENTED_EDGE('',*,*,#17073,.F.);
#23681=ORIENTED_EDGE('',*,*,#17074,.F.);
#23682=ORIENTED_EDGE('',*,*,#17073,.T.);
#23683=ORIENTED_EDGE('',*,*,#17075,.T.);
#23684=ORIENTED_EDGE('',*,*,#17076,.F.);
#23685=ORIENTED_EDGE('',*,*,#17075,.F.);
#23686=ORIENTED_EDGE('',*,*,#17072,.T.);
#23687=ORIENTED_EDGE('',*,*,#17077,.T.);
#23688=ORIENTED_EDGE('',*,*,#17078,.F.);
#23689=ORIENTED_EDGE('',*,*,#17077,.F.);
#23690=ORIENTED_EDGE('',*,*,#17071,.F.);
#23691=ORIENTED_EDGE('',*,*,#17079,.F.);
#23692=ORIENTED_EDGE('',*,*,#17080,.T.);
#23693=ORIENTED_EDGE('',*,*,#17081,.F.);
#23694=ORIENTED_EDGE('',*,*,#17082,.F.);
#23695=ORIENTED_EDGE('',*,*,#17083,.F.);
#23696=ORIENTED_EDGE('',*,*,#17082,.T.);
#23697=ORIENTED_EDGE('',*,*,#17084,.T.);
#23698=ORIENTED_EDGE('',*,*,#17085,.F.);
#23699=ORIENTED_EDGE('',*,*,#17084,.F.);
#23700=ORIENTED_EDGE('',*,*,#17081,.T.);
#23701=ORIENTED_EDGE('',*,*,#17086,.T.);
#23702=ORIENTED_EDGE('',*,*,#17087,.F.);
#23703=ORIENTED_EDGE('',*,*,#17086,.F.);
#23704=ORIENTED_EDGE('',*,*,#17080,.F.);
#23705=ORIENTED_EDGE('',*,*,#17088,.F.);
#23706=ORIENTED_EDGE('',*,*,#17089,.T.);
#23707=ORIENTED_EDGE('',*,*,#17090,.F.);
#23708=ORIENTED_EDGE('',*,*,#17091,.F.);
#23709=ORIENTED_EDGE('',*,*,#17092,.F.);
#23710=ORIENTED_EDGE('',*,*,#17091,.T.);
#23711=ORIENTED_EDGE('',*,*,#17093,.T.);
#23712=ORIENTED_EDGE('',*,*,#17094,.F.);
#23713=ORIENTED_EDGE('',*,*,#17093,.F.);
#23714=ORIENTED_EDGE('',*,*,#17090,.T.);
#23715=ORIENTED_EDGE('',*,*,#17095,.T.);
#23716=ORIENTED_EDGE('',*,*,#17096,.F.);
#23717=ORIENTED_EDGE('',*,*,#17095,.F.);
#23718=ORIENTED_EDGE('',*,*,#17089,.F.);
#23719=ORIENTED_EDGE('',*,*,#17097,.F.);
#23720=ORIENTED_EDGE('',*,*,#17098,.T.);
#23721=ORIENTED_EDGE('',*,*,#17099,.F.);
#23722=ORIENTED_EDGE('',*,*,#17100,.F.);
#23723=ORIENTED_EDGE('',*,*,#17101,.F.);
#23724=ORIENTED_EDGE('',*,*,#17100,.T.);
#23725=ORIENTED_EDGE('',*,*,#17102,.T.);
#23726=ORIENTED_EDGE('',*,*,#17103,.F.);
#23727=ORIENTED_EDGE('',*,*,#17102,.F.);
#23728=ORIENTED_EDGE('',*,*,#17099,.T.);
#23729=ORIENTED_EDGE('',*,*,#17104,.T.);
#23730=ORIENTED_EDGE('',*,*,#17105,.F.);
#23731=ORIENTED_EDGE('',*,*,#17104,.F.);
#23732=ORIENTED_EDGE('',*,*,#17098,.F.);
#23733=ORIENTED_EDGE('',*,*,#17106,.F.);
#23734=ORIENTED_EDGE('',*,*,#17107,.T.);
#23735=ORIENTED_EDGE('',*,*,#17108,.F.);
#23736=ORIENTED_EDGE('',*,*,#17109,.F.);
#23737=ORIENTED_EDGE('',*,*,#17110,.F.);
#23738=ORIENTED_EDGE('',*,*,#17109,.T.);
#23739=ORIENTED_EDGE('',*,*,#17111,.T.);
#23740=ORIENTED_EDGE('',*,*,#17112,.F.);
#23741=ORIENTED_EDGE('',*,*,#17111,.F.);
#23742=ORIENTED_EDGE('',*,*,#17108,.T.);
#23743=ORIENTED_EDGE('',*,*,#17113,.T.);
#23744=ORIENTED_EDGE('',*,*,#17114,.F.);
#23745=ORIENTED_EDGE('',*,*,#17113,.F.);
#23746=ORIENTED_EDGE('',*,*,#17107,.F.);
#23747=ORIENTED_EDGE('',*,*,#17115,.F.);
#23748=ORIENTED_EDGE('',*,*,#17116,.T.);
#23749=ORIENTED_EDGE('',*,*,#17117,.F.);
#23750=ORIENTED_EDGE('',*,*,#17118,.F.);
#23751=ORIENTED_EDGE('',*,*,#17119,.F.);
#23752=ORIENTED_EDGE('',*,*,#17118,.T.);
#23753=ORIENTED_EDGE('',*,*,#17120,.T.);
#23754=ORIENTED_EDGE('',*,*,#17121,.F.);
#23755=ORIENTED_EDGE('',*,*,#17120,.F.);
#23756=ORIENTED_EDGE('',*,*,#17117,.T.);
#23757=ORIENTED_EDGE('',*,*,#17122,.T.);
#23758=ORIENTED_EDGE('',*,*,#17123,.F.);
#23759=ORIENTED_EDGE('',*,*,#17122,.F.);
#23760=ORIENTED_EDGE('',*,*,#17116,.F.);
#23761=ORIENTED_EDGE('',*,*,#17124,.F.);
#23762=ORIENTED_EDGE('',*,*,#17125,.T.);
#23763=ORIENTED_EDGE('',*,*,#17126,.F.);
#23764=ORIENTED_EDGE('',*,*,#17127,.F.);
#23765=ORIENTED_EDGE('',*,*,#17128,.F.);
#23766=ORIENTED_EDGE('',*,*,#17127,.T.);
#23767=ORIENTED_EDGE('',*,*,#17129,.T.);
#23768=ORIENTED_EDGE('',*,*,#17130,.F.);
#23769=ORIENTED_EDGE('',*,*,#17129,.F.);
#23770=ORIENTED_EDGE('',*,*,#17126,.T.);
#23771=ORIENTED_EDGE('',*,*,#17131,.T.);
#23772=ORIENTED_EDGE('',*,*,#17132,.F.);
#23773=ORIENTED_EDGE('',*,*,#17131,.F.);
#23774=ORIENTED_EDGE('',*,*,#17125,.F.);
#23775=ORIENTED_EDGE('',*,*,#17133,.F.);
#23776=ORIENTED_EDGE('',*,*,#17134,.T.);
#23777=ORIENTED_EDGE('',*,*,#17135,.F.);
#23778=ORIENTED_EDGE('',*,*,#17136,.F.);
#23779=ORIENTED_EDGE('',*,*,#17137,.F.);
#23780=ORIENTED_EDGE('',*,*,#17136,.T.);
#23781=ORIENTED_EDGE('',*,*,#17138,.T.);
#23782=ORIENTED_EDGE('',*,*,#17139,.F.);
#23783=ORIENTED_EDGE('',*,*,#17138,.F.);
#23784=ORIENTED_EDGE('',*,*,#17135,.T.);
#23785=ORIENTED_EDGE('',*,*,#17140,.T.);
#23786=ORIENTED_EDGE('',*,*,#17141,.F.);
#23787=ORIENTED_EDGE('',*,*,#17140,.F.);
#23788=ORIENTED_EDGE('',*,*,#17134,.F.);
#23789=ORIENTED_EDGE('',*,*,#17142,.F.);
#23790=ORIENTED_EDGE('',*,*,#17143,.T.);
#23791=ORIENTED_EDGE('',*,*,#17144,.F.);
#23792=ORIENTED_EDGE('',*,*,#17145,.F.);
#23793=ORIENTED_EDGE('',*,*,#17146,.F.);
#23794=ORIENTED_EDGE('',*,*,#17145,.T.);
#23795=ORIENTED_EDGE('',*,*,#17147,.T.);
#23796=ORIENTED_EDGE('',*,*,#17148,.F.);
#23797=ORIENTED_EDGE('',*,*,#17147,.F.);
#23798=ORIENTED_EDGE('',*,*,#17144,.T.);
#23799=ORIENTED_EDGE('',*,*,#17149,.T.);
#23800=ORIENTED_EDGE('',*,*,#17150,.F.);
#23801=ORIENTED_EDGE('',*,*,#17149,.F.);
#23802=ORIENTED_EDGE('',*,*,#17143,.F.);
#23803=ORIENTED_EDGE('',*,*,#17151,.F.);
#23804=ORIENTED_EDGE('',*,*,#17152,.T.);
#23805=ORIENTED_EDGE('',*,*,#17153,.F.);
#23806=ORIENTED_EDGE('',*,*,#17154,.F.);
#23807=ORIENTED_EDGE('',*,*,#17155,.F.);
#23808=ORIENTED_EDGE('',*,*,#17154,.T.);
#23809=ORIENTED_EDGE('',*,*,#17156,.T.);
#23810=ORIENTED_EDGE('',*,*,#17157,.F.);
#23811=ORIENTED_EDGE('',*,*,#17156,.F.);
#23812=ORIENTED_EDGE('',*,*,#17153,.T.);
#23813=ORIENTED_EDGE('',*,*,#17158,.T.);
#23814=ORIENTED_EDGE('',*,*,#17159,.F.);
#23815=ORIENTED_EDGE('',*,*,#17158,.F.);
#23816=ORIENTED_EDGE('',*,*,#17152,.F.);
#23817=ORIENTED_EDGE('',*,*,#17160,.F.);
#23818=ORIENTED_EDGE('',*,*,#17161,.T.);
#23819=ORIENTED_EDGE('',*,*,#17162,.F.);
#23820=ORIENTED_EDGE('',*,*,#17163,.F.);
#23821=ORIENTED_EDGE('',*,*,#17164,.F.);
#23822=ORIENTED_EDGE('',*,*,#17163,.T.);
#23823=ORIENTED_EDGE('',*,*,#17165,.T.);
#23824=ORIENTED_EDGE('',*,*,#17166,.F.);
#23825=ORIENTED_EDGE('',*,*,#17165,.F.);
#23826=ORIENTED_EDGE('',*,*,#17162,.T.);
#23827=ORIENTED_EDGE('',*,*,#17167,.T.);
#23828=ORIENTED_EDGE('',*,*,#17168,.F.);
#23829=ORIENTED_EDGE('',*,*,#17167,.F.);
#23830=ORIENTED_EDGE('',*,*,#17161,.F.);
#23831=ORIENTED_EDGE('',*,*,#17169,.F.);
#23832=ORIENTED_EDGE('',*,*,#17170,.T.);
#23833=ORIENTED_EDGE('',*,*,#17171,.F.);
#23834=ORIENTED_EDGE('',*,*,#17172,.F.);
#23835=ORIENTED_EDGE('',*,*,#17173,.F.);
#23836=ORIENTED_EDGE('',*,*,#17172,.T.);
#23837=ORIENTED_EDGE('',*,*,#17174,.T.);
#23838=ORIENTED_EDGE('',*,*,#17175,.F.);
#23839=ORIENTED_EDGE('',*,*,#17174,.F.);
#23840=ORIENTED_EDGE('',*,*,#17171,.T.);
#23841=ORIENTED_EDGE('',*,*,#17176,.T.);
#23842=ORIENTED_EDGE('',*,*,#17177,.F.);
#23843=ORIENTED_EDGE('',*,*,#17176,.F.);
#23844=ORIENTED_EDGE('',*,*,#17170,.F.);
#23845=ORIENTED_EDGE('',*,*,#17178,.F.);
#23846=ORIENTED_EDGE('',*,*,#17179,.T.);
#23847=ORIENTED_EDGE('',*,*,#17180,.F.);
#23848=ORIENTED_EDGE('',*,*,#17181,.F.);
#23849=ORIENTED_EDGE('',*,*,#17182,.F.);
#23850=ORIENTED_EDGE('',*,*,#17181,.T.);
#23851=ORIENTED_EDGE('',*,*,#17183,.T.);
#23852=ORIENTED_EDGE('',*,*,#17184,.F.);
#23853=ORIENTED_EDGE('',*,*,#17183,.F.);
#23854=ORIENTED_EDGE('',*,*,#17180,.T.);
#23855=ORIENTED_EDGE('',*,*,#17185,.T.);
#23856=ORIENTED_EDGE('',*,*,#17186,.F.);
#23857=ORIENTED_EDGE('',*,*,#17185,.F.);
#23858=ORIENTED_EDGE('',*,*,#17179,.F.);
#23859=ORIENTED_EDGE('',*,*,#17187,.F.);
#23860=ORIENTED_EDGE('',*,*,#17188,.T.);
#23861=ORIENTED_EDGE('',*,*,#17189,.F.);
#23862=ORIENTED_EDGE('',*,*,#17190,.F.);
#23863=ORIENTED_EDGE('',*,*,#17191,.F.);
#23864=ORIENTED_EDGE('',*,*,#17190,.T.);
#23865=ORIENTED_EDGE('',*,*,#17192,.T.);
#23866=ORIENTED_EDGE('',*,*,#17193,.F.);
#23867=ORIENTED_EDGE('',*,*,#17194,.F.);
#23868=ORIENTED_EDGE('',*,*,#17192,.F.);
#23869=ORIENTED_EDGE('',*,*,#17189,.T.);
#23870=ORIENTED_EDGE('',*,*,#17195,.T.);
#23871=ORIENTED_EDGE('',*,*,#17196,.F.);
#23872=ORIENTED_EDGE('',*,*,#17195,.F.);
#23873=ORIENTED_EDGE('',*,*,#17188,.F.);
#23874=ORIENTED_EDGE('',*,*,#17197,.F.);
#23875=ORIENTED_EDGE('',*,*,#17198,.F.);
#23876=ORIENTED_EDGE('',*,*,#17199,.T.);
#23877=ORIENTED_EDGE('',*,*,#17200,.F.);
#23878=ORIENTED_EDGE('',*,*,#17201,.F.);
#23879=ORIENTED_EDGE('',*,*,#17202,.F.);
#23880=ORIENTED_EDGE('',*,*,#17201,.T.);
#23881=ORIENTED_EDGE('',*,*,#17203,.T.);
#23882=ORIENTED_EDGE('',*,*,#17204,.F.);
#23883=ORIENTED_EDGE('',*,*,#17203,.F.);
#23884=ORIENTED_EDGE('',*,*,#17200,.T.);
#23885=ORIENTED_EDGE('',*,*,#17205,.T.);
#23886=ORIENTED_EDGE('',*,*,#17206,.F.);
#23887=ORIENTED_EDGE('',*,*,#17205,.F.);
#23888=ORIENTED_EDGE('',*,*,#17199,.F.);
#23889=ORIENTED_EDGE('',*,*,#17207,.F.);
#23890=ORIENTED_EDGE('',*,*,#17208,.T.);
#23891=ORIENTED_EDGE('',*,*,#17209,.F.);
#23892=ORIENTED_EDGE('',*,*,#17210,.F.);
#23893=ORIENTED_EDGE('',*,*,#17211,.F.);
#23894=ORIENTED_EDGE('',*,*,#17210,.T.);
#23895=ORIENTED_EDGE('',*,*,#17212,.T.);
#23896=ORIENTED_EDGE('',*,*,#17213,.F.);
#23897=ORIENTED_EDGE('',*,*,#17212,.F.);
#23898=ORIENTED_EDGE('',*,*,#17209,.T.);
#23899=ORIENTED_EDGE('',*,*,#17214,.T.);
#23900=ORIENTED_EDGE('',*,*,#17215,.F.);
#23901=ORIENTED_EDGE('',*,*,#17214,.F.);
#23902=ORIENTED_EDGE('',*,*,#17208,.F.);
#23903=ORIENTED_EDGE('',*,*,#17216,.F.);
#23904=ORIENTED_EDGE('',*,*,#17217,.T.);
#23905=ORIENTED_EDGE('',*,*,#17218,.F.);
#23906=ORIENTED_EDGE('',*,*,#17219,.F.);
#23907=ORIENTED_EDGE('',*,*,#17220,.F.);
#23908=ORIENTED_EDGE('',*,*,#17219,.T.);
#23909=ORIENTED_EDGE('',*,*,#17221,.T.);
#23910=ORIENTED_EDGE('',*,*,#17222,.F.);
#23911=ORIENTED_EDGE('',*,*,#17221,.F.);
#23912=ORIENTED_EDGE('',*,*,#17218,.T.);
#23913=ORIENTED_EDGE('',*,*,#17223,.T.);
#23914=ORIENTED_EDGE('',*,*,#17224,.F.);
#23915=ORIENTED_EDGE('',*,*,#17223,.F.);
#23916=ORIENTED_EDGE('',*,*,#17217,.F.);
#23917=ORIENTED_EDGE('',*,*,#17225,.F.);
#23918=ORIENTED_EDGE('',*,*,#17226,.T.);
#23919=ORIENTED_EDGE('',*,*,#17227,.F.);
#23920=ORIENTED_EDGE('',*,*,#17228,.F.);
#23921=ORIENTED_EDGE('',*,*,#17229,.F.);
#23922=ORIENTED_EDGE('',*,*,#17228,.T.);
#23923=ORIENTED_EDGE('',*,*,#17230,.T.);
#23924=ORIENTED_EDGE('',*,*,#17231,.F.);
#23925=ORIENTED_EDGE('',*,*,#17230,.F.);
#23926=ORIENTED_EDGE('',*,*,#17227,.T.);
#23927=ORIENTED_EDGE('',*,*,#17232,.T.);
#23928=ORIENTED_EDGE('',*,*,#17233,.F.);
#23929=ORIENTED_EDGE('',*,*,#17232,.F.);
#23930=ORIENTED_EDGE('',*,*,#17226,.F.);
#23931=ORIENTED_EDGE('',*,*,#17234,.F.);
#23932=ORIENTED_EDGE('',*,*,#17235,.T.);
#23933=ORIENTED_EDGE('',*,*,#17236,.F.);
#23934=ORIENTED_EDGE('',*,*,#17237,.F.);
#23935=ORIENTED_EDGE('',*,*,#17238,.F.);
#23936=ORIENTED_EDGE('',*,*,#17237,.T.);
#23937=ORIENTED_EDGE('',*,*,#17239,.T.);
#23938=ORIENTED_EDGE('',*,*,#17240,.F.);
#23939=ORIENTED_EDGE('',*,*,#17239,.F.);
#23940=ORIENTED_EDGE('',*,*,#17236,.T.);
#23941=ORIENTED_EDGE('',*,*,#17241,.T.);
#23942=ORIENTED_EDGE('',*,*,#17242,.F.);
#23943=ORIENTED_EDGE('',*,*,#17241,.F.);
#23944=ORIENTED_EDGE('',*,*,#17235,.F.);
#23945=ORIENTED_EDGE('',*,*,#17243,.F.);
#23946=ORIENTED_EDGE('',*,*,#17244,.T.);
#23947=ORIENTED_EDGE('',*,*,#17245,.F.);
#23948=ORIENTED_EDGE('',*,*,#17246,.F.);
#23949=ORIENTED_EDGE('',*,*,#17247,.F.);
#23950=ORIENTED_EDGE('',*,*,#17246,.T.);
#23951=ORIENTED_EDGE('',*,*,#17248,.T.);
#23952=ORIENTED_EDGE('',*,*,#17249,.F.);
#23953=ORIENTED_EDGE('',*,*,#17248,.F.);
#23954=ORIENTED_EDGE('',*,*,#17245,.T.);
#23955=ORIENTED_EDGE('',*,*,#17250,.T.);
#23956=ORIENTED_EDGE('',*,*,#17251,.F.);
#23957=ORIENTED_EDGE('',*,*,#17250,.F.);
#23958=ORIENTED_EDGE('',*,*,#17244,.F.);
#23959=ORIENTED_EDGE('',*,*,#17252,.F.);
#23960=ORIENTED_EDGE('',*,*,#17253,.T.);
#23961=ORIENTED_EDGE('',*,*,#17254,.F.);
#23962=ORIENTED_EDGE('',*,*,#17255,.F.);
#23963=ORIENTED_EDGE('',*,*,#17256,.F.);
#23964=ORIENTED_EDGE('',*,*,#17255,.T.);
#23965=ORIENTED_EDGE('',*,*,#17257,.T.);
#23966=ORIENTED_EDGE('',*,*,#17258,.F.);
#23967=ORIENTED_EDGE('',*,*,#17257,.F.);
#23968=ORIENTED_EDGE('',*,*,#17254,.T.);
#23969=ORIENTED_EDGE('',*,*,#17259,.T.);
#23970=ORIENTED_EDGE('',*,*,#17260,.F.);
#23971=ORIENTED_EDGE('',*,*,#17259,.F.);
#23972=ORIENTED_EDGE('',*,*,#17253,.F.);
#23973=ORIENTED_EDGE('',*,*,#17261,.F.);
#23974=ORIENTED_EDGE('',*,*,#17262,.T.);
#23975=ORIENTED_EDGE('',*,*,#17263,.F.);
#23976=ORIENTED_EDGE('',*,*,#17264,.F.);
#23977=ORIENTED_EDGE('',*,*,#17265,.F.);
#23978=ORIENTED_EDGE('',*,*,#17264,.T.);
#23979=ORIENTED_EDGE('',*,*,#17266,.T.);
#23980=ORIENTED_EDGE('',*,*,#17267,.F.);
#23981=ORIENTED_EDGE('',*,*,#17266,.F.);
#23982=ORIENTED_EDGE('',*,*,#17263,.T.);
#23983=ORIENTED_EDGE('',*,*,#17268,.T.);
#23984=ORIENTED_EDGE('',*,*,#17269,.F.);
#23985=ORIENTED_EDGE('',*,*,#17268,.F.);
#23986=ORIENTED_EDGE('',*,*,#17262,.F.);
#23987=ORIENTED_EDGE('',*,*,#17270,.F.);
#23988=ORIENTED_EDGE('',*,*,#17271,.T.);
#23989=ORIENTED_EDGE('',*,*,#17272,.F.);
#23990=ORIENTED_EDGE('',*,*,#17273,.F.);
#23991=ORIENTED_EDGE('',*,*,#17274,.F.);
#23992=ORIENTED_EDGE('',*,*,#17273,.T.);
#23993=ORIENTED_EDGE('',*,*,#17275,.T.);
#23994=ORIENTED_EDGE('',*,*,#17276,.F.);
#23995=ORIENTED_EDGE('',*,*,#17275,.F.);
#23996=ORIENTED_EDGE('',*,*,#17272,.T.);
#23997=ORIENTED_EDGE('',*,*,#17277,.T.);
#23998=ORIENTED_EDGE('',*,*,#17278,.F.);
#23999=ORIENTED_EDGE('',*,*,#17277,.F.);
#24000=ORIENTED_EDGE('',*,*,#17271,.F.);
#24001=ORIENTED_EDGE('',*,*,#17279,.F.);
#24002=ORIENTED_EDGE('',*,*,#17280,.T.);
#24003=ORIENTED_EDGE('',*,*,#17281,.F.);
#24004=ORIENTED_EDGE('',*,*,#17282,.F.);
#24005=ORIENTED_EDGE('',*,*,#17283,.F.);
#24006=ORIENTED_EDGE('',*,*,#17282,.T.);
#24007=ORIENTED_EDGE('',*,*,#17284,.T.);
#24008=ORIENTED_EDGE('',*,*,#17285,.F.);
#24009=ORIENTED_EDGE('',*,*,#17284,.F.);
#24010=ORIENTED_EDGE('',*,*,#17281,.T.);
#24011=ORIENTED_EDGE('',*,*,#17286,.T.);
#24012=ORIENTED_EDGE('',*,*,#17287,.F.);
#24013=ORIENTED_EDGE('',*,*,#17286,.F.);
#24014=ORIENTED_EDGE('',*,*,#17280,.F.);
#24015=ORIENTED_EDGE('',*,*,#17288,.F.);
#24016=ORIENTED_EDGE('',*,*,#17289,.T.);
#24017=ORIENTED_EDGE('',*,*,#17290,.F.);
#24018=ORIENTED_EDGE('',*,*,#17291,.F.);
#24019=ORIENTED_EDGE('',*,*,#17292,.F.);
#24020=ORIENTED_EDGE('',*,*,#17291,.T.);
#24021=ORIENTED_EDGE('',*,*,#17293,.T.);
#24022=ORIENTED_EDGE('',*,*,#17294,.F.);
#24023=ORIENTED_EDGE('',*,*,#17293,.F.);
#24024=ORIENTED_EDGE('',*,*,#17290,.T.);
#24025=ORIENTED_EDGE('',*,*,#17295,.T.);
#24026=ORIENTED_EDGE('',*,*,#17296,.F.);
#24027=ORIENTED_EDGE('',*,*,#17295,.F.);
#24028=ORIENTED_EDGE('',*,*,#17289,.F.);
#24029=ORIENTED_EDGE('',*,*,#17297,.F.);
#24030=ORIENTED_EDGE('',*,*,#17298,.T.);
#24031=ORIENTED_EDGE('',*,*,#17299,.F.);
#24032=ORIENTED_EDGE('',*,*,#17300,.F.);
#24033=ORIENTED_EDGE('',*,*,#17301,.F.);
#24034=ORIENTED_EDGE('',*,*,#17300,.T.);
#24035=ORIENTED_EDGE('',*,*,#17302,.T.);
#24036=ORIENTED_EDGE('',*,*,#17303,.F.);
#24037=ORIENTED_EDGE('',*,*,#17302,.F.);
#24038=ORIENTED_EDGE('',*,*,#17299,.T.);
#24039=ORIENTED_EDGE('',*,*,#17304,.T.);
#24040=ORIENTED_EDGE('',*,*,#17305,.F.);
#24041=ORIENTED_EDGE('',*,*,#17304,.F.);
#24042=ORIENTED_EDGE('',*,*,#17298,.F.);
#24043=ORIENTED_EDGE('',*,*,#17306,.F.);
#24044=ORIENTED_EDGE('',*,*,#17307,.T.);
#24045=ORIENTED_EDGE('',*,*,#17308,.F.);
#24046=ORIENTED_EDGE('',*,*,#17309,.F.);
#24047=ORIENTED_EDGE('',*,*,#17310,.F.);
#24048=ORIENTED_EDGE('',*,*,#17309,.T.);
#24049=ORIENTED_EDGE('',*,*,#17311,.T.);
#24050=ORIENTED_EDGE('',*,*,#17312,.F.);
#24051=ORIENTED_EDGE('',*,*,#17311,.F.);
#24052=ORIENTED_EDGE('',*,*,#17308,.T.);
#24053=ORIENTED_EDGE('',*,*,#17313,.T.);
#24054=ORIENTED_EDGE('',*,*,#17314,.F.);
#24055=ORIENTED_EDGE('',*,*,#17313,.F.);
#24056=ORIENTED_EDGE('',*,*,#17307,.F.);
#24057=ORIENTED_EDGE('',*,*,#17315,.F.);
#24058=ORIENTED_EDGE('',*,*,#17316,.T.);
#24059=ORIENTED_EDGE('',*,*,#17317,.F.);
#24060=ORIENTED_EDGE('',*,*,#17318,.F.);
#24061=ORIENTED_EDGE('',*,*,#17319,.F.);
#24062=ORIENTED_EDGE('',*,*,#17318,.T.);
#24063=ORIENTED_EDGE('',*,*,#17320,.T.);
#24064=ORIENTED_EDGE('',*,*,#17321,.F.);
#24065=ORIENTED_EDGE('',*,*,#17320,.F.);
#24066=ORIENTED_EDGE('',*,*,#17317,.T.);
#24067=ORIENTED_EDGE('',*,*,#17322,.T.);
#24068=ORIENTED_EDGE('',*,*,#17323,.F.);
#24069=ORIENTED_EDGE('',*,*,#17322,.F.);
#24070=ORIENTED_EDGE('',*,*,#17316,.F.);
#24071=ORIENTED_EDGE('',*,*,#17324,.F.);
#24072=ORIENTED_EDGE('',*,*,#17325,.T.);
#24073=ORIENTED_EDGE('',*,*,#17326,.F.);
#24074=ORIENTED_EDGE('',*,*,#17327,.F.);
#24075=ORIENTED_EDGE('',*,*,#17328,.F.);
#24076=ORIENTED_EDGE('',*,*,#17327,.T.);
#24077=ORIENTED_EDGE('',*,*,#17329,.T.);
#24078=ORIENTED_EDGE('',*,*,#17330,.F.);
#24079=ORIENTED_EDGE('',*,*,#17329,.F.);
#24080=ORIENTED_EDGE('',*,*,#17326,.T.);
#24081=ORIENTED_EDGE('',*,*,#17331,.T.);
#24082=ORIENTED_EDGE('',*,*,#17332,.F.);
#24083=ORIENTED_EDGE('',*,*,#17331,.F.);
#24084=ORIENTED_EDGE('',*,*,#17325,.F.);
#24085=ORIENTED_EDGE('',*,*,#17333,.F.);
#24086=ORIENTED_EDGE('',*,*,#17334,.T.);
#24087=ORIENTED_EDGE('',*,*,#17335,.F.);
#24088=ORIENTED_EDGE('',*,*,#17336,.F.);
#24089=ORIENTED_EDGE('',*,*,#17337,.F.);
#24090=ORIENTED_EDGE('',*,*,#17336,.T.);
#24091=ORIENTED_EDGE('',*,*,#17338,.T.);
#24092=ORIENTED_EDGE('',*,*,#17339,.F.);
#24093=ORIENTED_EDGE('',*,*,#17338,.F.);
#24094=ORIENTED_EDGE('',*,*,#17335,.T.);
#24095=ORIENTED_EDGE('',*,*,#17340,.T.);
#24096=ORIENTED_EDGE('',*,*,#17341,.F.);
#24097=ORIENTED_EDGE('',*,*,#17340,.F.);
#24098=ORIENTED_EDGE('',*,*,#17334,.F.);
#24099=ORIENTED_EDGE('',*,*,#17342,.F.);
#24100=ORIENTED_EDGE('',*,*,#17343,.T.);
#24101=ORIENTED_EDGE('',*,*,#17344,.F.);
#24102=ORIENTED_EDGE('',*,*,#17345,.F.);
#24103=ORIENTED_EDGE('',*,*,#17346,.F.);
#24104=ORIENTED_EDGE('',*,*,#17345,.T.);
#24105=ORIENTED_EDGE('',*,*,#17347,.T.);
#24106=ORIENTED_EDGE('',*,*,#17348,.F.);
#24107=ORIENTED_EDGE('',*,*,#17347,.F.);
#24108=ORIENTED_EDGE('',*,*,#17344,.T.);
#24109=ORIENTED_EDGE('',*,*,#17349,.T.);
#24110=ORIENTED_EDGE('',*,*,#17350,.F.);
#24111=ORIENTED_EDGE('',*,*,#17349,.F.);
#24112=ORIENTED_EDGE('',*,*,#17343,.F.);
#24113=ORIENTED_EDGE('',*,*,#17351,.F.);
#24114=ORIENTED_EDGE('',*,*,#17352,.T.);
#24115=ORIENTED_EDGE('',*,*,#17353,.F.);
#24116=ORIENTED_EDGE('',*,*,#17354,.F.);
#24117=ORIENTED_EDGE('',*,*,#17355,.F.);
#24118=ORIENTED_EDGE('',*,*,#17354,.T.);
#24119=ORIENTED_EDGE('',*,*,#17356,.T.);
#24120=ORIENTED_EDGE('',*,*,#17357,.F.);
#24121=ORIENTED_EDGE('',*,*,#17356,.F.);
#24122=ORIENTED_EDGE('',*,*,#17353,.T.);
#24123=ORIENTED_EDGE('',*,*,#17358,.T.);
#24124=ORIENTED_EDGE('',*,*,#17359,.F.);
#24125=ORIENTED_EDGE('',*,*,#17358,.F.);
#24126=ORIENTED_EDGE('',*,*,#17352,.F.);
#24127=ORIENTED_EDGE('',*,*,#17360,.T.);
#24128=ORIENTED_EDGE('',*,*,#17361,.F.);
#24129=ORIENTED_EDGE('',*,*,#17360,.F.);
#24130=ORIENTED_EDGE('',*,*,#17362,.F.);
#24131=ORIENTED_EDGE('',*,*,#17363,.T.);
#24132=ORIENTED_EDGE('',*,*,#17364,.T.);
#24133=ORIENTED_EDGE('',*,*,#17365,.F.);
#24134=ORIENTED_EDGE('',*,*,#17366,.F.);
#24135=ORIENTED_EDGE('',*,*,#17367,.T.);
#24136=ORIENTED_EDGE('',*,*,#17368,.T.);
#24137=ORIENTED_EDGE('',*,*,#17363,.F.);
#24138=ORIENTED_EDGE('',*,*,#17369,.F.);
#24139=ORIENTED_EDGE('',*,*,#17370,.T.);
#24140=ORIENTED_EDGE('',*,*,#17371,.T.);
#24141=ORIENTED_EDGE('',*,*,#17367,.F.);
#24142=ORIENTED_EDGE('',*,*,#17372,.F.);
#24143=ORIENTED_EDGE('',*,*,#17373,.T.);
#24144=ORIENTED_EDGE('',*,*,#17374,.T.);
#24145=ORIENTED_EDGE('',*,*,#17370,.F.);
#24146=ORIENTED_EDGE('',*,*,#17375,.F.);
#24147=ORIENTED_EDGE('',*,*,#17376,.T.);
#24148=ORIENTED_EDGE('',*,*,#17377,.T.);
#24149=ORIENTED_EDGE('',*,*,#17373,.F.);
#24150=ORIENTED_EDGE('',*,*,#17378,.F.);
#24151=ORIENTED_EDGE('',*,*,#17365,.T.);
#24152=ORIENTED_EDGE('',*,*,#17379,.T.);
#24153=ORIENTED_EDGE('',*,*,#17376,.F.);
#24154=ORIENTED_EDGE('',*,*,#17379,.F.);
#24155=ORIENTED_EDGE('',*,*,#17364,.F.);
#24156=ORIENTED_EDGE('',*,*,#17368,.F.);
#24157=ORIENTED_EDGE('',*,*,#17371,.F.);
#24158=ORIENTED_EDGE('',*,*,#17374,.F.);
#24159=ORIENTED_EDGE('',*,*,#17377,.F.);
#24160=ORIENTED_EDGE('',*,*,#17361,.T.);
#24161=ORIENTED_EDGE('',*,*,#17380,.F.);
#24162=ORIENTED_EDGE('',*,*,#17023,.F.);
#24163=ORIENTED_EDGE('',*,*,#16765,.F.);
#24164=ORIENTED_EDGE('',*,*,#17024,.F.);
#24165=ORIENTED_EDGE('',*,*,#17381,.T.);
#24166=ORIENTED_EDGE('',*,*,#17380,.T.);
#24167=ORIENTED_EDGE('',*,*,#17381,.F.);
#24168=ORIENTED_EDGE('',*,*,#17382,.F.);
#24169=ORIENTED_EDGE('',*,*,#17383,.T.);
#24170=ORIENTED_EDGE('',*,*,#17197,.T.);
#24171=ORIENTED_EDGE('',*,*,#17187,.T.);
#24172=ORIENTED_EDGE('',*,*,#17191,.T.);
#24173=ORIENTED_EDGE('',*,*,#17384,.T.);
#24174=ORIENTED_EDGE('',*,*,#17033,.T.);
#24175=ORIENTED_EDGE('',*,*,#17384,.F.);
#24176=ORIENTED_EDGE('',*,*,#17193,.T.);
#24177=ORIENTED_EDGE('',*,*,#17194,.T.);
#24178=ORIENTED_EDGE('',*,*,#17196,.T.);
#24179=ORIENTED_EDGE('',*,*,#17383,.F.);
#24180=ORIENTED_EDGE('',*,*,#17040,.T.);
#24181=ORIENTED_EDGE('',*,*,#17042,.T.);
#24182=ORIENTED_EDGE('',*,*,#17034,.T.);
#24183=ORIENTED_EDGE('',*,*,#17038,.T.);
#24184=ORIENTED_EDGE('',*,*,#17049,.T.);
#24185=ORIENTED_EDGE('',*,*,#17051,.T.);
#24186=ORIENTED_EDGE('',*,*,#17043,.T.);
#24187=ORIENTED_EDGE('',*,*,#17047,.T.);
#24188=ORIENTED_EDGE('',*,*,#17058,.T.);
#24189=ORIENTED_EDGE('',*,*,#17060,.T.);
#24190=ORIENTED_EDGE('',*,*,#17052,.T.);
#24191=ORIENTED_EDGE('',*,*,#17056,.T.);
#24192=ORIENTED_EDGE('',*,*,#17067,.T.);
#24193=ORIENTED_EDGE('',*,*,#17069,.T.);
#24194=ORIENTED_EDGE('',*,*,#17061,.T.);
#24195=ORIENTED_EDGE('',*,*,#17065,.T.);
#24196=ORIENTED_EDGE('',*,*,#17076,.T.);
#24197=ORIENTED_EDGE('',*,*,#17078,.T.);
#24198=ORIENTED_EDGE('',*,*,#17070,.T.);
#24199=ORIENTED_EDGE('',*,*,#17074,.T.);
#24200=ORIENTED_EDGE('',*,*,#17085,.T.);
#24201=ORIENTED_EDGE('',*,*,#17087,.T.);
#24202=ORIENTED_EDGE('',*,*,#17079,.T.);
#24203=ORIENTED_EDGE('',*,*,#17083,.T.);
#24204=ORIENTED_EDGE('',*,*,#17094,.T.);
#24205=ORIENTED_EDGE('',*,*,#17096,.T.);
#24206=ORIENTED_EDGE('',*,*,#17088,.T.);
#24207=ORIENTED_EDGE('',*,*,#17092,.T.);
#24208=ORIENTED_EDGE('',*,*,#17103,.T.);
#24209=ORIENTED_EDGE('',*,*,#17105,.T.);
#24210=ORIENTED_EDGE('',*,*,#17097,.T.);
#24211=ORIENTED_EDGE('',*,*,#17101,.T.);
#24212=ORIENTED_EDGE('',*,*,#17112,.T.);
#24213=ORIENTED_EDGE('',*,*,#17114,.T.);
#24214=ORIENTED_EDGE('',*,*,#17106,.T.);
#24215=ORIENTED_EDGE('',*,*,#17110,.T.);
#24216=ORIENTED_EDGE('',*,*,#17121,.T.);
#24217=ORIENTED_EDGE('',*,*,#17123,.T.);
#24218=ORIENTED_EDGE('',*,*,#17115,.T.);
#24219=ORIENTED_EDGE('',*,*,#17119,.T.);
#24220=ORIENTED_EDGE('',*,*,#17130,.T.);
#24221=ORIENTED_EDGE('',*,*,#17132,.T.);
#24222=ORIENTED_EDGE('',*,*,#17124,.T.);
#24223=ORIENTED_EDGE('',*,*,#17128,.T.);
#24224=ORIENTED_EDGE('',*,*,#17139,.T.);
#24225=ORIENTED_EDGE('',*,*,#17141,.T.);
#24226=ORIENTED_EDGE('',*,*,#17133,.T.);
#24227=ORIENTED_EDGE('',*,*,#17137,.T.);
#24228=ORIENTED_EDGE('',*,*,#17148,.T.);
#24229=ORIENTED_EDGE('',*,*,#17150,.T.);
#24230=ORIENTED_EDGE('',*,*,#17142,.T.);
#24231=ORIENTED_EDGE('',*,*,#17146,.T.);
#24232=ORIENTED_EDGE('',*,*,#17157,.T.);
#24233=ORIENTED_EDGE('',*,*,#17159,.T.);
#24234=ORIENTED_EDGE('',*,*,#17151,.T.);
#24235=ORIENTED_EDGE('',*,*,#17155,.T.);
#24236=ORIENTED_EDGE('',*,*,#17166,.T.);
#24237=ORIENTED_EDGE('',*,*,#17168,.T.);
#24238=ORIENTED_EDGE('',*,*,#17160,.T.);
#24239=ORIENTED_EDGE('',*,*,#17164,.T.);
#24240=ORIENTED_EDGE('',*,*,#17175,.T.);
#24241=ORIENTED_EDGE('',*,*,#17177,.T.);
#24242=ORIENTED_EDGE('',*,*,#17169,.T.);
#24243=ORIENTED_EDGE('',*,*,#17173,.T.);
#24244=ORIENTED_EDGE('',*,*,#17184,.T.);
#24245=ORIENTED_EDGE('',*,*,#17186,.T.);
#24246=ORIENTED_EDGE('',*,*,#17178,.T.);
#24247=ORIENTED_EDGE('',*,*,#17182,.T.);
#24248=ORIENTED_EDGE('',*,*,#17204,.T.);
#24249=ORIENTED_EDGE('',*,*,#17206,.T.);
#24250=ORIENTED_EDGE('',*,*,#17198,.T.);
#24251=ORIENTED_EDGE('',*,*,#17202,.T.);
#24252=ORIENTED_EDGE('',*,*,#17213,.T.);
#24253=ORIENTED_EDGE('',*,*,#17215,.T.);
#24254=ORIENTED_EDGE('',*,*,#17207,.T.);
#24255=ORIENTED_EDGE('',*,*,#17211,.T.);
#24256=ORIENTED_EDGE('',*,*,#17222,.T.);
#24257=ORIENTED_EDGE('',*,*,#17224,.T.);
#24258=ORIENTED_EDGE('',*,*,#17216,.T.);
#24259=ORIENTED_EDGE('',*,*,#17220,.T.);
#24260=ORIENTED_EDGE('',*,*,#17231,.T.);
#24261=ORIENTED_EDGE('',*,*,#17233,.T.);
#24262=ORIENTED_EDGE('',*,*,#17225,.T.);
#24263=ORIENTED_EDGE('',*,*,#17229,.T.);
#24264=ORIENTED_EDGE('',*,*,#17240,.T.);
#24265=ORIENTED_EDGE('',*,*,#17242,.T.);
#24266=ORIENTED_EDGE('',*,*,#17234,.T.);
#24267=ORIENTED_EDGE('',*,*,#17238,.T.);
#24268=ORIENTED_EDGE('',*,*,#17249,.T.);
#24269=ORIENTED_EDGE('',*,*,#17251,.T.);
#24270=ORIENTED_EDGE('',*,*,#17243,.T.);
#24271=ORIENTED_EDGE('',*,*,#17247,.T.);
#24272=ORIENTED_EDGE('',*,*,#17258,.T.);
#24273=ORIENTED_EDGE('',*,*,#17260,.T.);
#24274=ORIENTED_EDGE('',*,*,#17252,.T.);
#24275=ORIENTED_EDGE('',*,*,#17256,.T.);
#24276=ORIENTED_EDGE('',*,*,#17267,.T.);
#24277=ORIENTED_EDGE('',*,*,#17269,.T.);
#24278=ORIENTED_EDGE('',*,*,#17261,.T.);
#24279=ORIENTED_EDGE('',*,*,#17265,.T.);
#24280=ORIENTED_EDGE('',*,*,#17276,.T.);
#24281=ORIENTED_EDGE('',*,*,#17278,.T.);
#24282=ORIENTED_EDGE('',*,*,#17270,.T.);
#24283=ORIENTED_EDGE('',*,*,#17274,.T.);
#24284=ORIENTED_EDGE('',*,*,#17285,.T.);
#24285=ORIENTED_EDGE('',*,*,#17287,.T.);
#24286=ORIENTED_EDGE('',*,*,#17279,.T.);
#24287=ORIENTED_EDGE('',*,*,#17283,.T.);
#24288=ORIENTED_EDGE('',*,*,#17294,.T.);
#24289=ORIENTED_EDGE('',*,*,#17296,.T.);
#24290=ORIENTED_EDGE('',*,*,#17288,.T.);
#24291=ORIENTED_EDGE('',*,*,#17292,.T.);
#24292=ORIENTED_EDGE('',*,*,#17303,.T.);
#24293=ORIENTED_EDGE('',*,*,#17305,.T.);
#24294=ORIENTED_EDGE('',*,*,#17297,.T.);
#24295=ORIENTED_EDGE('',*,*,#17301,.T.);
#24296=ORIENTED_EDGE('',*,*,#17312,.T.);
#24297=ORIENTED_EDGE('',*,*,#17314,.T.);
#24298=ORIENTED_EDGE('',*,*,#17306,.T.);
#24299=ORIENTED_EDGE('',*,*,#17310,.T.);
#24300=ORIENTED_EDGE('',*,*,#17321,.T.);
#24301=ORIENTED_EDGE('',*,*,#17323,.T.);
#24302=ORIENTED_EDGE('',*,*,#17315,.T.);
#24303=ORIENTED_EDGE('',*,*,#17319,.T.);
#24304=ORIENTED_EDGE('',*,*,#17330,.T.);
#24305=ORIENTED_EDGE('',*,*,#17332,.T.);
#24306=ORIENTED_EDGE('',*,*,#17324,.T.);
#24307=ORIENTED_EDGE('',*,*,#17328,.T.);
#24308=ORIENTED_EDGE('',*,*,#17339,.T.);
#24309=ORIENTED_EDGE('',*,*,#17341,.T.);
#24310=ORIENTED_EDGE('',*,*,#17333,.T.);
#24311=ORIENTED_EDGE('',*,*,#17337,.T.);
#24312=ORIENTED_EDGE('',*,*,#17348,.T.);
#24313=ORIENTED_EDGE('',*,*,#17350,.T.);
#24314=ORIENTED_EDGE('',*,*,#17342,.T.);
#24315=ORIENTED_EDGE('',*,*,#17346,.T.);
#24316=ORIENTED_EDGE('',*,*,#17357,.T.);
#24317=ORIENTED_EDGE('',*,*,#17359,.T.);
#24318=ORIENTED_EDGE('',*,*,#17351,.T.);
#24319=ORIENTED_EDGE('',*,*,#17355,.T.);
#24320=ORIENTED_EDGE('',*,*,#17385,.F.);
#24321=ORIENTED_EDGE('',*,*,#17386,.T.);
#24322=ORIENTED_EDGE('',*,*,#17382,.T.);
#24323=ORIENTED_EDGE('',*,*,#17386,.F.);
#24324=ORIENTED_EDGE('',*,*,#17385,.T.);
#24325=ORIENTED_EDGE('',*,*,#17362,.T.);
#24326=ORIENTED_EDGE('',*,*,#17378,.T.);
#24327=ORIENTED_EDGE('',*,*,#17375,.T.);
#24328=ORIENTED_EDGE('',*,*,#17372,.T.);
#24329=ORIENTED_EDGE('',*,*,#17369,.T.);
#24330=ORIENTED_EDGE('',*,*,#17366,.T.);
#28478=PLANE('',#32194);
#28479=PLANE('',#32196);
#28480=PLANE('',#32207);
#28481=PLANE('',#32209);
#28482=PLANE('',#32210);
#28483=PLANE('',#32212);
#28484=PLANE('',#32213);
#28485=PLANE('',#32215);
#28486=PLANE('',#32216);
#28487=PLANE('',#32218);
#28488=PLANE('',#32219);
#28489=PLANE('',#32221);
#28490=PLANE('',#32222);
#28491=PLANE('',#32224);
#28492=PLANE('',#32225);
#28493=PLANE('',#32227);
#28494=PLANE('',#32228);
#28495=PLANE('',#32230);
#28496=PLANE('',#32231);
#28497=PLANE('',#32233);
#28498=PLANE('',#32234);
#28499=PLANE('',#32236);
#28500=PLANE('',#32237);
#28501=PLANE('',#32239);
#28502=PLANE('',#32240);
#28503=PLANE('',#32242);
#28504=PLANE('',#32243);
#28505=PLANE('',#32245);
#28506=PLANE('',#32246);
#28507=PLANE('',#32248);
#28508=PLANE('',#32249);
#28509=PLANE('',#32251);
#28510=PLANE('',#32252);
#28511=PLANE('',#32254);
#28512=PLANE('',#32255);
#28513=PLANE('',#32257);
#28514=PLANE('',#32258);
#28515=PLANE('',#32260);
#28516=PLANE('',#32261);
#28517=PLANE('',#32263);
#28518=PLANE('',#32264);
#28519=PLANE('',#32266);
#28520=PLANE('',#32267);
#28521=PLANE('',#32269);
#28522=PLANE('',#32270);
#28523=PLANE('',#32272);
#28524=PLANE('',#32273);
#28525=PLANE('',#32275);
#28526=PLANE('',#32276);
#28527=PLANE('',#32278);
#28528=PLANE('',#32279);
#28529=PLANE('',#32281);
#28530=PLANE('',#32282);
#28531=PLANE('',#32284);
#28532=PLANE('',#32285);
#28533=PLANE('',#32287);
#28534=PLANE('',#32288);
#28535=PLANE('',#32290);
#28536=PLANE('',#32291);
#28537=PLANE('',#32293);
#28538=PLANE('',#32294);
#28539=PLANE('',#32296);
#28540=PLANE('',#32297);
#28541=PLANE('',#32299);
#28542=PLANE('',#32300);
#28543=PLANE('',#32302);
#28544=PLANE('',#32303);
#28545=PLANE('',#32305);
#28546=PLANE('',#32306);
#28547=PLANE('',#32308);
#28548=PLANE('',#32309);
#28549=PLANE('',#32311);
#28550=PLANE('',#32312);
#28551=PLANE('',#32315);
#28552=PLANE('',#32316);
#28553=PLANE('',#32319);
#28554=PLANE('',#32320);
#28555=PLANE('',#32322);
#28556=PLANE('',#32323);
#28557=PLANE('',#32325);
#28558=PLANE('',#32326);
#28559=PLANE('',#32328);
#28560=PLANE('',#32329);
#28561=PLANE('',#32331);
#28562=PLANE('',#32332);
#28563=PLANE('',#32334);
#28564=PLANE('',#32335);
#28565=PLANE('',#32337);
#28566=PLANE('',#32338);
#28567=PLANE('',#32340);
#28568=PLANE('',#32341);
#28569=PLANE('',#32343);
#28570=PLANE('',#32344);
#28571=PLANE('',#32346);
#28572=PLANE('',#32347);
#28573=PLANE('',#32349);
#28574=PLANE('',#32350);
#28575=PLANE('',#32352);
#28576=PLANE('',#32353);
#28577=PLANE('',#32355);
#28578=PLANE('',#32356);
#28579=PLANE('',#32358);
#28580=PLANE('',#32359);
#28581=PLANE('',#32361);
#28582=PLANE('',#32362);
#28583=PLANE('',#32364);
#28584=PLANE('',#32365);
#28585=PLANE('',#32367);
#28586=PLANE('',#32368);
#28587=PLANE('',#32370);
#28588=PLANE('',#32371);
#28589=PLANE('',#32373);
#28590=PLANE('',#32374);
#28591=PLANE('',#32376);
#28592=PLANE('',#32377);
#28593=PLANE('',#32379);
#28594=PLANE('',#32380);
#28595=PLANE('',#32382);
#28596=PLANE('',#32383);
#28597=PLANE('',#32385);
#28598=PLANE('',#32386);
#28599=PLANE('',#32388);
#28600=PLANE('',#32389);
#28601=PLANE('',#32391);
#28602=PLANE('',#32392);
#28603=PLANE('',#32394);
#28604=PLANE('',#32395);
#28605=PLANE('',#32397);
#28606=PLANE('',#32398);
#28607=PLANE('',#32400);
#28608=PLANE('',#32401);
#28609=PLANE('',#32403);
#28610=PLANE('',#32404);
#28611=PLANE('',#32406);
#28612=PLANE('',#32407);
#28613=PLANE('',#32409);
#28614=PLANE('',#32410);
#28615=PLANE('',#32412);
#28616=PLANE('',#32413);
#28617=PLANE('',#32415);
#28618=PLANE('',#32416);
#28619=PLANE('',#32418);
#28620=PLANE('',#32419);
#28621=PLANE('',#32421);
#28622=PLANE('',#32422);
#28623=PLANE('',#32424);
#28624=PLANE('',#32425);
#28625=PLANE('',#32429);
#28626=PLANE('',#32430);
#28627=PLANE('',#32431);
#28628=PLANE('',#32432);
#28629=PLANE('',#32433);
#28630=PLANE('',#32434);
#28631=PLANE('',#32435);
#28632=PLANE('',#32436);
#28633=PLANE('',#32443);
#29718=ADVANCED_FACE('',(#4390),#578,.T.);
#29719=ADVANCED_FACE('',(#4391),#579,.T.);
#29720=ADVANCED_FACE('',(#4392),#580,.T.);
#29721=ADVANCED_FACE('',(#4393),#581,.T.);
#29722=ADVANCED_FACE('',(#4394),#582,.T.);
#29723=ADVANCED_FACE('',(#4395),#583,.T.);
#29724=ADVANCED_FACE('',(#4396),#584,.T.);
#29725=ADVANCED_FACE('',(#4397),#585,.T.);
#29726=ADVANCED_FACE('',(#4398),#586,.T.);
#29727=ADVANCED_FACE('',(#4399),#587,.T.);
#29728=ADVANCED_FACE('',(#4400),#588,.T.);
#29729=ADVANCED_FACE('',(#4401),#589,.T.);
#29730=ADVANCED_FACE('',(#4402),#590,.T.);
#29731=ADVANCED_FACE('',(#4403),#591,.T.);
#29732=ADVANCED_FACE('',(#4404),#592,.T.);
#29733=ADVANCED_FACE('',(#4405),#593,.T.);
#29734=ADVANCED_FACE('',(#4406),#594,.T.);
#29735=ADVANCED_FACE('',(#4407),#595,.T.);
#29736=ADVANCED_FACE('',(#4408),#596,.T.);
#29737=ADVANCED_FACE('',(#4409),#597,.T.);
#29738=ADVANCED_FACE('',(#4410),#598,.T.);
#29739=ADVANCED_FACE('',(#4411),#599,.T.);
#29740=ADVANCED_FACE('',(#4412),#600,.T.);
#29741=ADVANCED_FACE('',(#4413),#601,.T.);
#29742=ADVANCED_FACE('',(#4414),#602,.T.);
#29743=ADVANCED_FACE('',(#4415),#603,.T.);
#29744=ADVANCED_FACE('',(#4416),#604,.T.);
#29745=ADVANCED_FACE('',(#4417),#605,.T.);
#29746=ADVANCED_FACE('',(#4418),#606,.T.);
#29747=ADVANCED_FACE('',(#4419),#607,.T.);
#29748=ADVANCED_FACE('',(#4420),#608,.T.);
#29749=ADVANCED_FACE('',(#4421),#609,.T.);
#29750=ADVANCED_FACE('',(#4422),#610,.T.);
#29751=ADVANCED_FACE('',(#4423),#611,.T.);
#29752=ADVANCED_FACE('',(#4424),#612,.T.);
#29753=ADVANCED_FACE('',(#4425),#613,.T.);
#29754=ADVANCED_FACE('',(#4426),#614,.T.);
#29755=ADVANCED_FACE('',(#4427),#615,.T.);
#29756=ADVANCED_FACE('',(#4428),#616,.T.);
#29757=ADVANCED_FACE('',(#4429),#617,.T.);
#29758=ADVANCED_FACE('',(#4430),#618,.T.);
#29759=ADVANCED_FACE('',(#4431),#619,.T.);
#29760=ADVANCED_FACE('',(#4432),#620,.T.);
#29761=ADVANCED_FACE('',(#4433),#621,.T.);
#29762=ADVANCED_FACE('',(#4434),#622,.T.);
#29763=ADVANCED_FACE('',(#4435),#623,.T.);
#29764=ADVANCED_FACE('',(#4436),#624,.T.);
#29765=ADVANCED_FACE('',(#4437),#625,.T.);
#29766=ADVANCED_FACE('',(#4438),#626,.T.);
#29767=ADVANCED_FACE('',(#4439),#627,.T.);
#29768=ADVANCED_FACE('',(#4440),#628,.T.);
#29769=ADVANCED_FACE('',(#4441),#629,.T.);
#29770=ADVANCED_FACE('',(#4442),#630,.T.);
#29771=ADVANCED_FACE('',(#4443),#631,.T.);
#29772=ADVANCED_FACE('',(#4444),#632,.T.);
#29773=ADVANCED_FACE('',(#4445),#633,.T.);
#29774=ADVANCED_FACE('',(#4446),#634,.T.);
#29775=ADVANCED_FACE('',(#4447),#635,.T.);
#29776=ADVANCED_FACE('',(#4448),#636,.T.);
#29777=ADVANCED_FACE('',(#4449),#637,.T.);
#29778=ADVANCED_FACE('',(#4450),#638,.T.);
#29779=ADVANCED_FACE('',(#4451),#639,.T.);
#29780=ADVANCED_FACE('',(#4452),#640,.T.);
#29781=ADVANCED_FACE('',(#4453),#641,.T.);
#29782=ADVANCED_FACE('',(#4454),#642,.T.);
#29783=ADVANCED_FACE('',(#4455),#643,.T.);
#29784=ADVANCED_FACE('',(#4456),#644,.T.);
#29785=ADVANCED_FACE('',(#4457),#645,.T.);
#29786=ADVANCED_FACE('',(#4458),#646,.T.);
#29787=ADVANCED_FACE('',(#4459),#647,.T.);
#29788=ADVANCED_FACE('',(#4460),#648,.T.);
#29789=ADVANCED_FACE('',(#4461),#649,.T.);
#29790=ADVANCED_FACE('',(#4462),#650,.T.);
#29791=ADVANCED_FACE('',(#4463),#651,.T.);
#29792=ADVANCED_FACE('',(#4464),#652,.T.);
#29793=ADVANCED_FACE('',(#4465),#653,.T.);
#29794=ADVANCED_FACE('',(#4466),#654,.T.);
#29795=ADVANCED_FACE('',(#4467),#655,.T.);
#29796=ADVANCED_FACE('',(#4468),#656,.T.);
#29797=ADVANCED_FACE('',(#4469),#657,.T.);
#29798=ADVANCED_FACE('',(#4470),#658,.T.);
#29799=ADVANCED_FACE('',(#4471),#659,.T.);
#29800=ADVANCED_FACE('',(#4472),#660,.T.);
#29801=ADVANCED_FACE('',(#4473),#661,.T.);
#29802=ADVANCED_FACE('',(#4474),#28478,.F.);
#29803=ADVANCED_FACE('',(#4475),#422,.F.);
#29804=ADVANCED_FACE('',(#4476),#28479,.T.);
#29805=ADVANCED_FACE('',(#4477),#662,.T.);
#29806=ADVANCED_FACE('',(#4478),#423,.F.);
#29807=ADVANCED_FACE('',(#4479),#160,.F.);
#29808=ADVANCED_FACE('',(#4480),#663,.T.);
#29809=ADVANCED_FACE('',(#4481,#3488),#28480,.T.);
#29810=ADVANCED_FACE('',(#4482),#28481,.F.);
#29811=ADVANCED_FACE('',(#4483),#28482,.T.);
#29812=ADVANCED_FACE('',(#4484),#28483,.F.);
#29813=ADVANCED_FACE('',(#4485),#28484,.F.);
#29814=ADVANCED_FACE('',(#4486),#28485,.F.);
#29815=ADVANCED_FACE('',(#4487),#28486,.T.);
#29816=ADVANCED_FACE('',(#4488),#28487,.F.);
#29817=ADVANCED_FACE('',(#4489),#28488,.F.);
#29818=ADVANCED_FACE('',(#4490),#28489,.F.);
#29819=ADVANCED_FACE('',(#4491),#28490,.T.);
#29820=ADVANCED_FACE('',(#4492),#28491,.F.);
#29821=ADVANCED_FACE('',(#4493),#28492,.F.);
#29822=ADVANCED_FACE('',(#4494),#28493,.F.);
#29823=ADVANCED_FACE('',(#4495),#28494,.T.);
#29824=ADVANCED_FACE('',(#4496),#28495,.F.);
#29825=ADVANCED_FACE('',(#4497),#28496,.F.);
#29826=ADVANCED_FACE('',(#4498),#28497,.F.);
#29827=ADVANCED_FACE('',(#4499),#28498,.T.);
#29828=ADVANCED_FACE('',(#4500),#28499,.F.);
#29829=ADVANCED_FACE('',(#4501),#28500,.F.);
#29830=ADVANCED_FACE('',(#4502),#28501,.F.);
#29831=ADVANCED_FACE('',(#4503),#28502,.T.);
#29832=ADVANCED_FACE('',(#4504),#28503,.F.);
#29833=ADVANCED_FACE('',(#4505),#28504,.F.);
#29834=ADVANCED_FACE('',(#4506),#28505,.F.);
#29835=ADVANCED_FACE('',(#4507),#28506,.T.);
#29836=ADVANCED_FACE('',(#4508),#28507,.F.);
#29837=ADVANCED_FACE('',(#4509),#28508,.F.);
#29838=ADVANCED_FACE('',(#4510),#28509,.F.);
#29839=ADVANCED_FACE('',(#4511),#28510,.T.);
#29840=ADVANCED_FACE('',(#4512),#28511,.F.);
#29841=ADVANCED_FACE('',(#4513),#28512,.F.);
#29842=ADVANCED_FACE('',(#4514),#28513,.F.);
#29843=ADVANCED_FACE('',(#4515),#28514,.T.);
#29844=ADVANCED_FACE('',(#4516),#28515,.F.);
#29845=ADVANCED_FACE('',(#4517),#28516,.F.);
#29846=ADVANCED_FACE('',(#4518),#28517,.F.);
#29847=ADVANCED_FACE('',(#4519),#28518,.T.);
#29848=ADVANCED_FACE('',(#4520),#28519,.F.);
#29849=ADVANCED_FACE('',(#4521),#28520,.F.);
#29850=ADVANCED_FACE('',(#4522),#28521,.F.);
#29851=ADVANCED_FACE('',(#4523),#28522,.T.);
#29852=ADVANCED_FACE('',(#4524),#28523,.F.);
#29853=ADVANCED_FACE('',(#4525),#28524,.F.);
#29854=ADVANCED_FACE('',(#4526),#28525,.F.);
#29855=ADVANCED_FACE('',(#4527),#28526,.T.);
#29856=ADVANCED_FACE('',(#4528),#28527,.F.);
#29857=ADVANCED_FACE('',(#4529),#28528,.F.);
#29858=ADVANCED_FACE('',(#4530),#28529,.F.);
#29859=ADVANCED_FACE('',(#4531),#28530,.T.);
#29860=ADVANCED_FACE('',(#4532),#28531,.F.);
#29861=ADVANCED_FACE('',(#4533),#28532,.F.);
#29862=ADVANCED_FACE('',(#4534),#28533,.F.);
#29863=ADVANCED_FACE('',(#4535),#28534,.T.);
#29864=ADVANCED_FACE('',(#4536),#28535,.F.);
#29865=ADVANCED_FACE('',(#4537),#28536,.F.);
#29866=ADVANCED_FACE('',(#4538),#28537,.F.);
#29867=ADVANCED_FACE('',(#4539),#28538,.T.);
#29868=ADVANCED_FACE('',(#4540),#28539,.F.);
#29869=ADVANCED_FACE('',(#4541),#28540,.F.);
#29870=ADVANCED_FACE('',(#4542),#28541,.F.);
#29871=ADVANCED_FACE('',(#4543),#28542,.T.);
#29872=ADVANCED_FACE('',(#4544),#28543,.F.);
#29873=ADVANCED_FACE('',(#4545),#28544,.F.);
#29874=ADVANCED_FACE('',(#4546),#28545,.F.);
#29875=ADVANCED_FACE('',(#4547),#28546,.T.);
#29876=ADVANCED_FACE('',(#4548),#28547,.F.);
#29877=ADVANCED_FACE('',(#4549),#28548,.F.);
#29878=ADVANCED_FACE('',(#4550),#28549,.F.);
#29879=ADVANCED_FACE('',(#4551),#28550,.T.);
#29880=ADVANCED_FACE('',(#4552),#28551,.F.);
#29881=ADVANCED_FACE('',(#4553),#28552,.F.);
#29882=ADVANCED_FACE('',(#4554),#28553,.F.);
#29883=ADVANCED_FACE('',(#4555),#28554,.T.);
#29884=ADVANCED_FACE('',(#4556),#28555,.F.);
#29885=ADVANCED_FACE('',(#4557),#28556,.F.);
#29886=ADVANCED_FACE('',(#4558),#28557,.F.);
#29887=ADVANCED_FACE('',(#4559),#28558,.T.);
#29888=ADVANCED_FACE('',(#4560),#28559,.F.);
#29889=ADVANCED_FACE('',(#4561),#28560,.F.);
#29890=ADVANCED_FACE('',(#4562),#28561,.F.);
#29891=ADVANCED_FACE('',(#4563),#28562,.T.);
#29892=ADVANCED_FACE('',(#4564),#28563,.F.);
#29893=ADVANCED_FACE('',(#4565),#28564,.F.);
#29894=ADVANCED_FACE('',(#4566),#28565,.F.);
#29895=ADVANCED_FACE('',(#4567),#28566,.T.);
#29896=ADVANCED_FACE('',(#4568),#28567,.F.);
#29897=ADVANCED_FACE('',(#4569),#28568,.F.);
#29898=ADVANCED_FACE('',(#4570),#28569,.F.);
#29899=ADVANCED_FACE('',(#4571),#28570,.T.);
#29900=ADVANCED_FACE('',(#4572),#28571,.F.);
#29901=ADVANCED_FACE('',(#4573),#28572,.F.);
#29902=ADVANCED_FACE('',(#4574),#28573,.F.);
#29903=ADVANCED_FACE('',(#4575),#28574,.T.);
#29904=ADVANCED_FACE('',(#4576),#28575,.F.);
#29905=ADVANCED_FACE('',(#4577),#28576,.F.);
#29906=ADVANCED_FACE('',(#4578),#28577,.F.);
#29907=ADVANCED_FACE('',(#4579),#28578,.T.);
#29908=ADVANCED_FACE('',(#4580),#28579,.F.);
#29909=ADVANCED_FACE('',(#4581),#28580,.F.);
#29910=ADVANCED_FACE('',(#4582),#28581,.F.);
#29911=ADVANCED_FACE('',(#4583),#28582,.T.);
#29912=ADVANCED_FACE('',(#4584),#28583,.F.);
#29913=ADVANCED_FACE('',(#4585),#28584,.F.);
#29914=ADVANCED_FACE('',(#4586),#28585,.F.);
#29915=ADVANCED_FACE('',(#4587),#28586,.T.);
#29916=ADVANCED_FACE('',(#4588),#28587,.F.);
#29917=ADVANCED_FACE('',(#4589),#28588,.F.);
#29918=ADVANCED_FACE('',(#4590),#28589,.F.);
#29919=ADVANCED_FACE('',(#4591),#28590,.T.);
#29920=ADVANCED_FACE('',(#4592),#28591,.F.);
#29921=ADVANCED_FACE('',(#4593),#28592,.F.);
#29922=ADVANCED_FACE('',(#4594),#28593,.F.);
#29923=ADVANCED_FACE('',(#4595),#28594,.T.);
#29924=ADVANCED_FACE('',(#4596),#28595,.F.);
#29925=ADVANCED_FACE('',(#4597),#28596,.F.);
#29926=ADVANCED_FACE('',(#4598),#28597,.F.);
#29927=ADVANCED_FACE('',(#4599),#28598,.T.);
#29928=ADVANCED_FACE('',(#4600),#28599,.F.);
#29929=ADVANCED_FACE('',(#4601),#28600,.F.);
#29930=ADVANCED_FACE('',(#4602),#28601,.F.);
#29931=ADVANCED_FACE('',(#4603),#28602,.T.);
#29932=ADVANCED_FACE('',(#4604),#28603,.F.);
#29933=ADVANCED_FACE('',(#4605),#28604,.F.);
#29934=ADVANCED_FACE('',(#4606),#28605,.F.);
#29935=ADVANCED_FACE('',(#4607),#28606,.T.);
#29936=ADVANCED_FACE('',(#4608),#28607,.F.);
#29937=ADVANCED_FACE('',(#4609),#28608,.F.);
#29938=ADVANCED_FACE('',(#4610),#28609,.F.);
#29939=ADVANCED_FACE('',(#4611),#28610,.T.);
#29940=ADVANCED_FACE('',(#4612),#28611,.F.);
#29941=ADVANCED_FACE('',(#4613),#28612,.F.);
#29942=ADVANCED_FACE('',(#4614),#28613,.F.);
#29943=ADVANCED_FACE('',(#4615),#28614,.T.);
#29944=ADVANCED_FACE('',(#4616),#28615,.F.);
#29945=ADVANCED_FACE('',(#4617),#28616,.F.);
#29946=ADVANCED_FACE('',(#4618),#28617,.F.);
#29947=ADVANCED_FACE('',(#4619),#28618,.T.);
#29948=ADVANCED_FACE('',(#4620),#28619,.F.);
#29949=ADVANCED_FACE('',(#4621),#28620,.F.);
#29950=ADVANCED_FACE('',(#4622),#28621,.F.);
#29951=ADVANCED_FACE('',(#4623),#28622,.T.);
#29952=ADVANCED_FACE('',(#4624),#28623,.F.);
#29953=ADVANCED_FACE('',(#4625),#28624,.F.);
#29954=ADVANCED_FACE('',(#4626),#2039,.F.);
#29955=ADVANCED_FACE('',(#4627),#28625,.F.);
#29956=ADVANCED_FACE('',(#4628),#28626,.F.);
#29957=ADVANCED_FACE('',(#4629),#28627,.F.);
#29958=ADVANCED_FACE('',(#4630),#28628,.F.);
#29959=ADVANCED_FACE('',(#4631),#28629,.F.);
#29960=ADVANCED_FACE('',(#4632),#28630,.F.);
#29961=ADVANCED_FACE('',(#4633,#3489),#28631,.F.);
#29962=ADVANCED_FACE('',(#4634),#28632,.T.);
#29963=ADVANCED_FACE('',(#4635),#2040,.T.);
#29964=ADVANCED_FACE('',(#4636,#3490,#3491,#3492,#3493,#3494,#3495,#3496,
#3497,#3498,#3499,#3500,#3501,#3502,#3503,#3504,#3505,#3506,#3507,#3508,
#3509,#3510,#3511,#3512,#3513,#3514,#3515,#3516,#3517,#3518,#3519,#3520,
#3521,#3522,#3523,#3524),#664,.T.);
#29965=ADVANCED_FACE('',(#4637),#2041,.T.);
#29966=ADVANCED_FACE('',(#4638,#3525),#28633,.T.);
#30672=CLOSED_SHELL('',(#29718,#29719,#29720,#29721,#29722,#29723,#29724,
#29725,#29726,#29727,#29728,#29729,#29730,#29731,#29732,#29733,#29734,#29735,
#29736,#29737,#29738,#29739,#29740,#29741,#29742,#29743,#29744,#29745,#29746,
#29747,#29748,#29749,#29750,#29751,#29752,#29753,#29754,#29755,#29756,#29757,
#29758,#29759,#29760,#29761,#29762,#29763,#29764,#29765,#29766,#29767,#29768,
#29769,#29770,#29771,#29772,#29773,#29774,#29775,#29776,#29777,#29778,#29779,
#29780,#29781,#29782,#29783,#29784,#29785,#29786,#29787,#29788,#29789,#29790,
#29791,#29792,#29793,#29794,#29795,#29796,#29797,#29798,#29799,#29800,#29801,
#29802,#29803,#29804,#29805,#29806,#29807,#29808,#29809,#29810,#29811,#29812,
#29813,#29814,#29815,#29816,#29817,#29818,#29819,#29820,#29821,#29822,#29823,
#29824,#29825,#29826,#29827,#29828,#29829,#29830,#29831,#29832,#29833,#29834,
#29835,#29836,#29837,#29838,#29839,#29840,#29841,#29842,#29843,#29844,#29845,
#29846,#29847,#29848,#29849,#29850,#29851,#29852,#29853,#29854,#29855,#29856,
#29857,#29858,#29859,#29860,#29861,#29862,#29863,#29864,#29865,#29866,#29867,
#29868,#29869,#29870,#29871,#29872,#29873,#29874,#29875,#29876,#29877,#29878,
#29879,#29880,#29881,#29882,#29883,#29884,#29885,#29886,#29887,#29888,#29889,
#29890,#29891,#29892,#29893,#29894,#29895,#29896,#29897,#29898,#29899,#29900,
#29901,#29902,#29903,#29904,#29905,#29906,#29907,#29908,#29909,#29910,#29911,
#29912,#29913,#29914,#29915,#29916,#29917,#29918,#29919,#29920,#29921,#29922,
#29923,#29924,#29925,#29926,#29927,#29928,#29929,#29930,#29931,#29932,#29933,
#29934,#29935,#29936,#29937,#29938,#29939,#29940,#29941,#29942,#29943,#29944,
#29945,#29946,#29947,#29948,#29949,#29950,#29951,#29952,#29953,#29954,#29955,
#29956,#29957,#29958,#29959,#29960,#29961,#29962,#29963,#29964,#29965,#29966));
#32107=AXIS2_PLACEMENT_3D('',#49569,#36948,#36949);
#32108=AXIS2_PLACEMENT_3D('',#49570,#36950,#36951);
#32109=AXIS2_PLACEMENT_3D('',#49586,#36953,#36954);
#32110=AXIS2_PLACEMENT_3D('',#49594,#36955,#36956);
#32111=AXIS2_PLACEMENT_3D('',#49642,#36958,#36959);
#32112=AXIS2_PLACEMENT_3D('',#49690,#36961,#36962);
#32113=AXIS2_PLACEMENT_3D('',#49741,#36964,#36965);
#32114=AXIS2_PLACEMENT_3D('',#49792,#36967,#36968);
#32115=AXIS2_PLACEMENT_3D('',#49840,#36970,#36971);
#32116=AXIS2_PLACEMENT_3D('',#49888,#36973,#36974);
#32117=AXIS2_PLACEMENT_3D('',#49942,#36976,#36977);
#32118=AXIS2_PLACEMENT_3D('',#49990,#36979,#36980);
#32119=AXIS2_PLACEMENT_3D('',#50038,#36982,#36983);
#32120=AXIS2_PLACEMENT_3D('',#50092,#36985,#36986);
#32121=AXIS2_PLACEMENT_3D('',#50140,#36988,#36989);
#32122=AXIS2_PLACEMENT_3D('',#50188,#36991,#36992);
#32123=AXIS2_PLACEMENT_3D('',#50236,#36994,#36995);
#32124=AXIS2_PLACEMENT_3D('',#50290,#36997,#36998);
#32125=AXIS2_PLACEMENT_3D('',#50338,#37000,#37001);
#32126=AXIS2_PLACEMENT_3D('',#50386,#37003,#37004);
#32127=AXIS2_PLACEMENT_3D('',#50440,#37006,#37007);
#32128=AXIS2_PLACEMENT_3D('',#50488,#37009,#37010);
#32129=AXIS2_PLACEMENT_3D('',#50536,#37012,#37013);
#32130=AXIS2_PLACEMENT_3D('',#50590,#37015,#37016);
#32131=AXIS2_PLACEMENT_3D('',#50638,#37018,#37019);
#32132=AXIS2_PLACEMENT_3D('',#50686,#37021,#37022);
#32133=AXIS2_PLACEMENT_3D('',#50734,#37024,#37025);
#32134=AXIS2_PLACEMENT_3D('',#50788,#37027,#37028);
#32135=AXIS2_PLACEMENT_3D('',#50836,#37030,#37031);
#32136=AXIS2_PLACEMENT_3D('',#50884,#37033,#37034);
#32137=AXIS2_PLACEMENT_3D('',#50938,#37036,#37037);
#32138=AXIS2_PLACEMENT_3D('',#50986,#37039,#37040);
#32139=AXIS2_PLACEMENT_3D('',#51034,#37042,#37043);
#32140=AXIS2_PLACEMENT_3D('',#51088,#37045,#37046);
#32141=AXIS2_PLACEMENT_3D('',#51136,#37048,#37049);
#32142=AXIS2_PLACEMENT_3D('',#51184,#37051,#37052);
#32143=AXIS2_PLACEMENT_3D('',#51232,#37054,#37055);
#32144=AXIS2_PLACEMENT_3D('',#51286,#37057,#37058);
#32145=AXIS2_PLACEMENT_3D('',#51334,#37060,#37061);
#32146=AXIS2_PLACEMENT_3D('',#51382,#37063,#37064);
#32147=AXIS2_PLACEMENT_3D('',#51436,#37066,#37067);
#32148=AXIS2_PLACEMENT_3D('',#51484,#37069,#37070);
#32149=AXIS2_PLACEMENT_3D('',#51532,#37072,#37073);
#32150=AXIS2_PLACEMENT_3D('',#51586,#37075,#37076);
#32151=AXIS2_PLACEMENT_3D('',#51634,#37078,#37079);
#32152=AXIS2_PLACEMENT_3D('',#51646,#37081,#37082);
#32153=AXIS2_PLACEMENT_3D('',#51652,#37083,#37084);
#32154=AXIS2_PLACEMENT_3D('',#51676,#37086,#37087);
#32155=AXIS2_PLACEMENT_3D('',#51701,#37089,#37090);
#32156=AXIS2_PLACEMENT_3D('',#51726,#37092,#37093);
#32157=AXIS2_PLACEMENT_3D('',#51750,#37095,#37096);
#32158=AXIS2_PLACEMENT_3D('',#51775,#37098,#37099);
#32159=AXIS2_PLACEMENT_3D('',#51800,#37101,#37102);
#32160=AXIS2_PLACEMENT_3D('',#51824,#37104,#37105);
#32161=AXIS2_PLACEMENT_3D('',#51849,#37107,#37108);
#32162=AXIS2_PLACEMENT_3D('',#51874,#37110,#37111);
#32163=AXIS2_PLACEMENT_3D('',#51898,#37113,#37114);
#32164=AXIS2_PLACEMENT_3D('',#51922,#37116,#37117);
#32165=AXIS2_PLACEMENT_3D('',#51947,#37119,#37120);
#32166=AXIS2_PLACEMENT_3D('',#51972,#37122,#37123);
#32167=AXIS2_PLACEMENT_3D('',#51996,#37125,#37126);
#32168=AXIS2_PLACEMENT_3D('',#52021,#37128,#37129);
#32169=AXIS2_PLACEMENT_3D('',#52046,#37131,#37132);
#32170=AXIS2_PLACEMENT_3D('',#52070,#37134,#37135);
#32171=AXIS2_PLACEMENT_3D('',#52095,#37137,#37138);
#32172=AXIS2_PLACEMENT_3D('',#52120,#37140,#37141);
#32173=AXIS2_PLACEMENT_3D('',#52144,#37143,#37144);
#32174=AXIS2_PLACEMENT_3D('',#52168,#37146,#37147);
#32175=AXIS2_PLACEMENT_3D('',#52193,#37149,#37150);
#32176=AXIS2_PLACEMENT_3D('',#52218,#37152,#37153);
#32177=AXIS2_PLACEMENT_3D('',#52242,#37155,#37156);
#32178=AXIS2_PLACEMENT_3D('',#52267,#37158,#37159);
#32179=AXIS2_PLACEMENT_3D('',#52292,#37161,#37162);
#32180=AXIS2_PLACEMENT_3D('',#52316,#37164,#37165);
#32181=AXIS2_PLACEMENT_3D('',#52341,#37167,#37168);
#32182=AXIS2_PLACEMENT_3D('',#52366,#37170,#37171);
#32183=AXIS2_PLACEMENT_3D('',#52390,#37173,#37174);
#32184=AXIS2_PLACEMENT_3D('',#52414,#37176,#37177);
#32185=AXIS2_PLACEMENT_3D('',#52439,#37179,#37180);
#32186=AXIS2_PLACEMENT_3D('',#52464,#37182,#37183);
#32187=AXIS2_PLACEMENT_3D('',#52488,#37185,#37186);
#32188=AXIS2_PLACEMENT_3D('',#52513,#37188,#37189);
#32189=AXIS2_PLACEMENT_3D('',#52538,#37191,#37192);
#32190=AXIS2_PLACEMENT_3D('',#52562,#37194,#37195);
#32191=AXIS2_PLACEMENT_3D('',#52587,#37197,#37198);
#32192=AXIS2_PLACEMENT_3D('',#52611,#37200,#37201);
#32193=AXIS2_PLACEMENT_3D('',#52636,#37203,#37204);
#32194=AXIS2_PLACEMENT_3D('',#52660,#37206,#37207);
#32195=AXIS2_PLACEMENT_3D('',#52748,#37208,#37209);
#32196=AXIS2_PLACEMENT_3D('',#54028,#37210,#37211);
#32197=AXIS2_PLACEMENT_3D('',#54030,#37212,#37213);
#32198=AXIS2_PLACEMENT_3D('',#54031,#37214,#37215);
#32199=AXIS2_PLACEMENT_3D('',#54118,#37216,#37217);
#32200=AXIS2_PLACEMENT_3D('',#54119,#37218,#37219);
#32201=AXIS2_PLACEMENT_3D('',#55224,#37220,#37221);
#32202=AXIS2_PLACEMENT_3D('',#55226,#37222,#37223);
#32203=AXIS2_PLACEMENT_3D('',#55228,#37224,#37225);
#32204=AXIS2_PLACEMENT_3D('',#55229,#37226,#37227);
#32205=AXIS2_PLACEMENT_3D('',#55230,#37228,#37229);
#32206=AXIS2_PLACEMENT_3D('',#55231,#37230,#37231);
#32207=AXIS2_PLACEMENT_3D('',#55232,#37232,#37233);
#32208=AXIS2_PLACEMENT_3D('',#55234,#37234,#37235);
#32209=AXIS2_PLACEMENT_3D('',#55235,#37236,#37237);
#32210=AXIS2_PLACEMENT_3D('',#55244,#37242,#37243);
#32211=AXIS2_PLACEMENT_3D('',#55246,#37244,#37245);
#32212=AXIS2_PLACEMENT_3D('',#55248,#37247,#37248);
#32213=AXIS2_PLACEMENT_3D('',#55252,#37251,#37252);
#32214=AXIS2_PLACEMENT_3D('',#55253,#37253,#37254);
#32215=AXIS2_PLACEMENT_3D('',#55254,#37255,#37256);
#32216=AXIS2_PLACEMENT_3D('',#55263,#37261,#37262);
#32217=AXIS2_PLACEMENT_3D('',#55265,#37263,#37264);
#32218=AXIS2_PLACEMENT_3D('',#55267,#37266,#37267);
#32219=AXIS2_PLACEMENT_3D('',#55271,#37270,#37271);
#32220=AXIS2_PLACEMENT_3D('',#55272,#37272,#37273);
#32221=AXIS2_PLACEMENT_3D('',#55273,#37274,#37275);
#32222=AXIS2_PLACEMENT_3D('',#55282,#37280,#37281);
#32223=AXIS2_PLACEMENT_3D('',#55284,#37282,#37283);
#32224=AXIS2_PLACEMENT_3D('',#55286,#37285,#37286);
#32225=AXIS2_PLACEMENT_3D('',#55290,#37289,#37290);
#32226=AXIS2_PLACEMENT_3D('',#55291,#37291,#37292);
#32227=AXIS2_PLACEMENT_3D('',#55292,#37293,#37294);
#32228=AXIS2_PLACEMENT_3D('',#55301,#37299,#37300);
#32229=AXIS2_PLACEMENT_3D('',#55303,#37301,#37302);
#32230=AXIS2_PLACEMENT_3D('',#55305,#37304,#37305);
#32231=AXIS2_PLACEMENT_3D('',#55309,#37308,#37309);
#32232=AXIS2_PLACEMENT_3D('',#55310,#37310,#37311);
#32233=AXIS2_PLACEMENT_3D('',#55311,#37312,#37313);
#32234=AXIS2_PLACEMENT_3D('',#55320,#37318,#37319);
#32235=AXIS2_PLACEMENT_3D('',#55322,#37320,#37321);
#32236=AXIS2_PLACEMENT_3D('',#55324,#37323,#37324);
#32237=AXIS2_PLACEMENT_3D('',#55328,#37327,#37328);
#32238=AXIS2_PLACEMENT_3D('',#55329,#37329,#37330);
#32239=AXIS2_PLACEMENT_3D('',#55330,#37331,#37332);
#32240=AXIS2_PLACEMENT_3D('',#55339,#37337,#37338);
#32241=AXIS2_PLACEMENT_3D('',#55341,#37339,#37340);
#32242=AXIS2_PLACEMENT_3D('',#55343,#37342,#37343);
#32243=AXIS2_PLACEMENT_3D('',#55347,#37346,#37347);
#32244=AXIS2_PLACEMENT_3D('',#55348,#37348,#37349);
#32245=AXIS2_PLACEMENT_3D('',#55349,#37350,#37351);
#32246=AXIS2_PLACEMENT_3D('',#55358,#37356,#37357);
#32247=AXIS2_PLACEMENT_3D('',#55360,#37358,#37359);
#32248=AXIS2_PLACEMENT_3D('',#55362,#37361,#37362);
#32249=AXIS2_PLACEMENT_3D('',#55366,#37365,#37366);
#32250=AXIS2_PLACEMENT_3D('',#55367,#37367,#37368);
#32251=AXIS2_PLACEMENT_3D('',#55368,#37369,#37370);
#32252=AXIS2_PLACEMENT_3D('',#55377,#37375,#37376);
#32253=AXIS2_PLACEMENT_3D('',#55379,#37377,#37378);
#32254=AXIS2_PLACEMENT_3D('',#55381,#37380,#37381);
#32255=AXIS2_PLACEMENT_3D('',#55385,#37384,#37385);
#32256=AXIS2_PLACEMENT_3D('',#55386,#37386,#37387);
#32257=AXIS2_PLACEMENT_3D('',#55387,#37388,#37389);
#32258=AXIS2_PLACEMENT_3D('',#55396,#37394,#37395);
#32259=AXIS2_PLACEMENT_3D('',#55398,#37396,#37397);
#32260=AXIS2_PLACEMENT_3D('',#55400,#37399,#37400);
#32261=AXIS2_PLACEMENT_3D('',#55404,#37403,#37404);
#32262=AXIS2_PLACEMENT_3D('',#55405,#37405,#37406);
#32263=AXIS2_PLACEMENT_3D('',#55406,#37407,#37408);
#32264=AXIS2_PLACEMENT_3D('',#55415,#37413,#37414);
#32265=AXIS2_PLACEMENT_3D('',#55417,#37415,#37416);
#32266=AXIS2_PLACEMENT_3D('',#55419,#37418,#37419);
#32267=AXIS2_PLACEMENT_3D('',#55423,#37422,#37423);
#32268=AXIS2_PLACEMENT_3D('',#55424,#37424,#37425);
#32269=AXIS2_PLACEMENT_3D('',#55425,#37426,#37427);
#32270=AXIS2_PLACEMENT_3D('',#55434,#37432,#37433);
#32271=AXIS2_PLACEMENT_3D('',#55436,#37434,#37435);
#32272=AXIS2_PLACEMENT_3D('',#55438,#37437,#37438);
#32273=AXIS2_PLACEMENT_3D('',#55442,#37441,#37442);
#32274=AXIS2_PLACEMENT_3D('',#55443,#37443,#37444);
#32275=AXIS2_PLACEMENT_3D('',#55444,#37445,#37446);
#32276=AXIS2_PLACEMENT_3D('',#55453,#37451,#37452);
#32277=AXIS2_PLACEMENT_3D('',#55455,#37453,#37454);
#32278=AXIS2_PLACEMENT_3D('',#55457,#37456,#37457);
#32279=AXIS2_PLACEMENT_3D('',#55461,#37460,#37461);
#32280=AXIS2_PLACEMENT_3D('',#55462,#37462,#37463);
#32281=AXIS2_PLACEMENT_3D('',#55463,#37464,#37465);
#32282=AXIS2_PLACEMENT_3D('',#55472,#37470,#37471);
#32283=AXIS2_PLACEMENT_3D('',#55474,#37472,#37473);
#32284=AXIS2_PLACEMENT_3D('',#55476,#37475,#37476);
#32285=AXIS2_PLACEMENT_3D('',#55480,#37479,#37480);
#32286=AXIS2_PLACEMENT_3D('',#55481,#37481,#37482);
#32287=AXIS2_PLACEMENT_3D('',#55482,#37483,#37484);
#32288=AXIS2_PLACEMENT_3D('',#55491,#37489,#37490);
#32289=AXIS2_PLACEMENT_3D('',#55493,#37491,#37492);
#32290=AXIS2_PLACEMENT_3D('',#55495,#37494,#37495);
#32291=AXIS2_PLACEMENT_3D('',#55499,#37498,#37499);
#32292=AXIS2_PLACEMENT_3D('',#55500,#37500,#37501);
#32293=AXIS2_PLACEMENT_3D('',#55501,#37502,#37503);
#32294=AXIS2_PLACEMENT_3D('',#55510,#37508,#37509);
#32295=AXIS2_PLACEMENT_3D('',#55512,#37510,#37511);
#32296=AXIS2_PLACEMENT_3D('',#55514,#37513,#37514);
#32297=AXIS2_PLACEMENT_3D('',#55518,#37517,#37518);
#32298=AXIS2_PLACEMENT_3D('',#55519,#37519,#37520);
#32299=AXIS2_PLACEMENT_3D('',#55520,#37521,#37522);
#32300=AXIS2_PLACEMENT_3D('',#55529,#37527,#37528);
#32301=AXIS2_PLACEMENT_3D('',#55531,#37529,#37530);
#32302=AXIS2_PLACEMENT_3D('',#55533,#37532,#37533);
#32303=AXIS2_PLACEMENT_3D('',#55537,#37536,#37537);
#32304=AXIS2_PLACEMENT_3D('',#55538,#37538,#37539);
#32305=AXIS2_PLACEMENT_3D('',#55539,#37540,#37541);
#32306=AXIS2_PLACEMENT_3D('',#55548,#37546,#37547);
#32307=AXIS2_PLACEMENT_3D('',#55550,#37548,#37549);
#32308=AXIS2_PLACEMENT_3D('',#55552,#37551,#37552);
#32309=AXIS2_PLACEMENT_3D('',#55556,#37555,#37556);
#32310=AXIS2_PLACEMENT_3D('',#55557,#37557,#37558);
#32311=AXIS2_PLACEMENT_3D('',#55558,#37559,#37560);
#32312=AXIS2_PLACEMENT_3D('',#55567,#37565,#37566);
#32313=AXIS2_PLACEMENT_3D('',#55569,#37567,#37568);
#32314=AXIS2_PLACEMENT_3D('',#55572,#37570,#37571);
#32315=AXIS2_PLACEMENT_3D('',#55573,#37572,#37573);
#32316=AXIS2_PLACEMENT_3D('',#55577,#37576,#37577);
#32317=AXIS2_PLACEMENT_3D('',#55579,#37578,#37579);
#32318=AXIS2_PLACEMENT_3D('',#55580,#37580,#37581);
#32319=AXIS2_PLACEMENT_3D('',#55581,#37582,#37583);
#32320=AXIS2_PLACEMENT_3D('',#55590,#37588,#37589);
#32321=AXIS2_PLACEMENT_3D('',#55592,#37590,#37591);
#32322=AXIS2_PLACEMENT_3D('',#55594,#37593,#37594);
#32323=AXIS2_PLACEMENT_3D('',#55598,#37597,#37598);
#32324=AXIS2_PLACEMENT_3D('',#55599,#37599,#37600);
#32325=AXIS2_PLACEMENT_3D('',#55600,#37601,#37602);
#32326=AXIS2_PLACEMENT_3D('',#55609,#37607,#37608);
#32327=AXIS2_PLACEMENT_3D('',#55611,#37609,#37610);
#32328=AXIS2_PLACEMENT_3D('',#55613,#37612,#37613);
#32329=AXIS2_PLACEMENT_3D('',#55617,#37616,#37617);
#32330=AXIS2_PLACEMENT_3D('',#55618,#37618,#37619);
#32331=AXIS2_PLACEMENT_3D('',#55619,#37620,#37621);
#32332=AXIS2_PLACEMENT_3D('',#55628,#37626,#37627);
#32333=AXIS2_PLACEMENT_3D('',#55630,#37628,#37629);
#32334=AXIS2_PLACEMENT_3D('',#55632,#37631,#37632);
#32335=AXIS2_PLACEMENT_3D('',#55636,#37635,#37636);
#32336=AXIS2_PLACEMENT_3D('',#55637,#37637,#37638);
#32337=AXIS2_PLACEMENT_3D('',#55638,#37639,#37640);
#32338=AXIS2_PLACEMENT_3D('',#55647,#37645,#37646);
#32339=AXIS2_PLACEMENT_3D('',#55649,#37647,#37648);
#32340=AXIS2_PLACEMENT_3D('',#55651,#37650,#37651);
#32341=AXIS2_PLACEMENT_3D('',#55655,#37654,#37655);
#32342=AXIS2_PLACEMENT_3D('',#55656,#37656,#37657);
#32343=AXIS2_PLACEMENT_3D('',#55657,#37658,#37659);
#32344=AXIS2_PLACEMENT_3D('',#55666,#37664,#37665);
#32345=AXIS2_PLACEMENT_3D('',#55668,#37666,#37667);
#32346=AXIS2_PLACEMENT_3D('',#55670,#37669,#37670);
#32347=AXIS2_PLACEMENT_3D('',#55674,#37673,#37674);
#32348=AXIS2_PLACEMENT_3D('',#55675,#37675,#37676);
#32349=AXIS2_PLACEMENT_3D('',#55676,#37677,#37678);
#32350=AXIS2_PLACEMENT_3D('',#55685,#37683,#37684);
#32351=AXIS2_PLACEMENT_3D('',#55687,#37685,#37686);
#32352=AXIS2_PLACEMENT_3D('',#55689,#37688,#37689);
#32353=AXIS2_PLACEMENT_3D('',#55693,#37692,#37693);
#32354=AXIS2_PLACEMENT_3D('',#55694,#37694,#37695);
#32355=AXIS2_PLACEMENT_3D('',#55695,#37696,#37697);
#32356=AXIS2_PLACEMENT_3D('',#55704,#37702,#37703);
#32357=AXIS2_PLACEMENT_3D('',#55706,#37704,#37705);
#32358=AXIS2_PLACEMENT_3D('',#55708,#37707,#37708);
#32359=AXIS2_PLACEMENT_3D('',#55712,#37711,#37712);
#32360=AXIS2_PLACEMENT_3D('',#55713,#37713,#37714);
#32361=AXIS2_PLACEMENT_3D('',#55714,#37715,#37716);
#32362=AXIS2_PLACEMENT_3D('',#55723,#37721,#37722);
#32363=AXIS2_PLACEMENT_3D('',#55725,#37723,#37724);
#32364=AXIS2_PLACEMENT_3D('',#55727,#37726,#37727);
#32365=AXIS2_PLACEMENT_3D('',#55731,#37730,#37731);
#32366=AXIS2_PLACEMENT_3D('',#55732,#37732,#37733);
#32367=AXIS2_PLACEMENT_3D('',#55733,#37734,#37735);
#32368=AXIS2_PLACEMENT_3D('',#55742,#37740,#37741);
#32369=AXIS2_PLACEMENT_3D('',#55744,#37742,#37743);
#32370=AXIS2_PLACEMENT_3D('',#55746,#37745,#37746);
#32371=AXIS2_PLACEMENT_3D('',#55750,#37749,#37750);
#32372=AXIS2_PLACEMENT_3D('',#55751,#37751,#37752);
#32373=AXIS2_PLACEMENT_3D('',#55752,#37753,#37754);
#32374=AXIS2_PLACEMENT_3D('',#55761,#37759,#37760);
#32375=AXIS2_PLACEMENT_3D('',#55763,#37761,#37762);
#32376=AXIS2_PLACEMENT_3D('',#55765,#37764,#37765);
#32377=AXIS2_PLACEMENT_3D('',#55769,#37768,#37769);
#32378=AXIS2_PLACEMENT_3D('',#55770,#37770,#37771);
#32379=AXIS2_PLACEMENT_3D('',#55771,#37772,#37773);
#32380=AXIS2_PLACEMENT_3D('',#55780,#37778,#37779);
#32381=AXIS2_PLACEMENT_3D('',#55782,#37780,#37781);
#32382=AXIS2_PLACEMENT_3D('',#55784,#37783,#37784);
#32383=AXIS2_PLACEMENT_3D('',#55788,#37787,#37788);
#32384=AXIS2_PLACEMENT_3D('',#55789,#37789,#37790);
#32385=AXIS2_PLACEMENT_3D('',#55790,#37791,#37792);
#32386=AXIS2_PLACEMENT_3D('',#55799,#37797,#37798);
#32387=AXIS2_PLACEMENT_3D('',#55801,#37799,#37800);
#32388=AXIS2_PLACEMENT_3D('',#55803,#37802,#37803);
#32389=AXIS2_PLACEMENT_3D('',#55807,#37806,#37807);
#32390=AXIS2_PLACEMENT_3D('',#55808,#37808,#37809);
#32391=AXIS2_PLACEMENT_3D('',#55809,#37810,#37811);
#32392=AXIS2_PLACEMENT_3D('',#55818,#37816,#37817);
#32393=AXIS2_PLACEMENT_3D('',#55820,#37818,#37819);
#32394=AXIS2_PLACEMENT_3D('',#55822,#37821,#37822);
#32395=AXIS2_PLACEMENT_3D('',#55826,#37825,#37826);
#32396=AXIS2_PLACEMENT_3D('',#55827,#37827,#37828);
#32397=AXIS2_PLACEMENT_3D('',#55828,#37829,#37830);
#32398=AXIS2_PLACEMENT_3D('',#55837,#37835,#37836);
#32399=AXIS2_PLACEMENT_3D('',#55839,#37837,#37838);
#32400=AXIS2_PLACEMENT_3D('',#55841,#37840,#37841);
#32401=AXIS2_PLACEMENT_3D('',#55845,#37844,#37845);
#32402=AXIS2_PLACEMENT_3D('',#55846,#37846,#37847);
#32403=AXIS2_PLACEMENT_3D('',#55847,#37848,#37849);
#32404=AXIS2_PLACEMENT_3D('',#55856,#37854,#37855);
#32405=AXIS2_PLACEMENT_3D('',#55858,#37856,#37857);
#32406=AXIS2_PLACEMENT_3D('',#55860,#37859,#37860);
#32407=AXIS2_PLACEMENT_3D('',#55864,#37863,#37864);
#32408=AXIS2_PLACEMENT_3D('',#55865,#37865,#37866);
#32409=AXIS2_PLACEMENT_3D('',#55866,#37867,#37868);
#32410=AXIS2_PLACEMENT_3D('',#55875,#37873,#37874);
#32411=AXIS2_PLACEMENT_3D('',#55877,#37875,#37876);
#32412=AXIS2_PLACEMENT_3D('',#55879,#37878,#37879);
#32413=AXIS2_PLACEMENT_3D('',#55883,#37882,#37883);
#32414=AXIS2_PLACEMENT_3D('',#55884,#37884,#37885);
#32415=AXIS2_PLACEMENT_3D('',#55885,#37886,#37887);
#32416=AXIS2_PLACEMENT_3D('',#55894,#37892,#37893);
#32417=AXIS2_PLACEMENT_3D('',#55896,#37894,#37895);
#32418=AXIS2_PLACEMENT_3D('',#55898,#37897,#37898);
#32419=AXIS2_PLACEMENT_3D('',#55902,#37901,#37902);
#32420=AXIS2_PLACEMENT_3D('',#55903,#37903,#37904);
#32421=AXIS2_PLACEMENT_3D('',#55904,#37905,#37906);
#32422=AXIS2_PLACEMENT_3D('',#55913,#37911,#37912);
#32423=AXIS2_PLACEMENT_3D('',#55915,#37913,#37914);
#32424=AXIS2_PLACEMENT_3D('',#55917,#37916,#37917);
#32425=AXIS2_PLACEMENT_3D('',#55921,#37920,#37921);
#32426=AXIS2_PLACEMENT_3D('',#55922,#37922,#37923);
#32427=AXIS2_PLACEMENT_3D('',#55923,#37924,#37925);
#32428=AXIS2_PLACEMENT_3D('',#55927,#37927,#37928);
#32429=AXIS2_PLACEMENT_3D('',#55928,#37929,#37930);
#32430=AXIS2_PLACEMENT_3D('',#55937,#37935,#37936);
#32431=AXIS2_PLACEMENT_3D('',#55943,#37940,#37941);
#32432=AXIS2_PLACEMENT_3D('',#55949,#37945,#37946);
#32433=AXIS2_PLACEMENT_3D('',#55955,#37950,#37951);
#32434=AXIS2_PLACEMENT_3D('',#55961,#37955,#37956);
#32435=AXIS2_PLACEMENT_3D('',#55964,#37959,#37960);
#32436=AXIS2_PLACEMENT_3D('',#55965,#37961,#37962);
#32437=AXIS2_PLACEMENT_3D('',#55967,#37963,#37964);
#32438=AXIS2_PLACEMENT_3D('',#55968,#37965,#37966);
#32439=AXIS2_PLACEMENT_3D('',#55970,#37968,#37969);
#32440=AXIS2_PLACEMENT_3D('',#55972,#37970,#37971);
#32441=AXIS2_PLACEMENT_3D('',#55975,#37974,#37975);
#32442=AXIS2_PLACEMENT_3D('',#55977,#37976,#37977);
#32443=AXIS2_PLACEMENT_3D('',#55979,#37979,#37980);
#36948=DIRECTION('axis',(0.,0.,1.));
#36949=DIRECTION('refdir',(1.,0.,0.));
#36950=DIRECTION('center_axis',(1.,0.,0.));
#36951=DIRECTION('ref_axis',(0.,1.,0.));
#36952=DIRECTION('',(-1.,0.,0.));
#36953=DIRECTION('center_axis',(1.,0.,0.));
#36954=DIRECTION('ref_axis',(0.,1.,0.));
#36955=DIRECTION('center_axis',(1.,0.,0.));
#36956=DIRECTION('ref_axis',(0.,1.,0.));
#36957=DIRECTION('',(-1.,0.,0.));
#36958=DIRECTION('center_axis',(1.,0.,0.));
#36959=DIRECTION('ref_axis',(0.,1.,0.));
#36960=DIRECTION('',(-1.,0.,0.));
#36961=DIRECTION('center_axis',(1.,0.,0.));
#36962=DIRECTION('ref_axis',(0.,1.,0.));
#36963=DIRECTION('',(-1.,0.,0.));
#36964=DIRECTION('center_axis',(1.,0.,0.));
#36965=DIRECTION('ref_axis',(0.,1.,0.));
#36966=DIRECTION('',(-1.,0.,0.));
#36967=DIRECTION('center_axis',(1.,0.,0.));
#36968=DIRECTION('ref_axis',(0.,1.,0.));
#36969=DIRECTION('',(-1.,0.,0.));
#36970=DIRECTION('center_axis',(1.,0.,0.));
#36971=DIRECTION('ref_axis',(0.,1.,0.));
#36972=DIRECTION('',(-1.,0.,0.));
#36973=DIRECTION('center_axis',(1.,0.,0.));
#36974=DIRECTION('ref_axis',(0.,1.,0.));
#36975=DIRECTION('',(-1.,0.,0.));
#36976=DIRECTION('center_axis',(1.,0.,0.));
#36977=DIRECTION('ref_axis',(0.,1.,0.));
#36978=DIRECTION('',(-1.,0.,0.));
#36979=DIRECTION('center_axis',(1.,0.,0.));
#36980=DIRECTION('ref_axis',(0.,1.,0.));
#36981=DIRECTION('',(-1.,0.,0.));
#36982=DIRECTION('center_axis',(1.,0.,0.));
#36983=DIRECTION('ref_axis',(0.,1.,0.));
#36984=DIRECTION('',(-1.,0.,0.));
#36985=DIRECTION('center_axis',(1.,0.,0.));
#36986=DIRECTION('ref_axis',(0.,1.,0.));
#36987=DIRECTION('',(-1.,0.,0.));
#36988=DIRECTION('center_axis',(1.,0.,0.));
#36989=DIRECTION('ref_axis',(0.,1.,0.));
#36990=DIRECTION('',(-1.,0.,0.));
#36991=DIRECTION('center_axis',(1.,0.,0.));
#36992=DIRECTION('ref_axis',(0.,1.,0.));
#36993=DIRECTION('',(-1.,0.,0.));
#36994=DIRECTION('center_axis',(1.,0.,0.));
#36995=DIRECTION('ref_axis',(0.,1.,0.));
#36996=DIRECTION('',(-1.,0.,0.));
#36997=DIRECTION('center_axis',(1.,0.,0.));
#36998=DIRECTION('ref_axis',(0.,1.,0.));
#36999=DIRECTION('',(-1.,0.,0.));
#37000=DIRECTION('center_axis',(1.,0.,0.));
#37001=DIRECTION('ref_axis',(0.,1.,0.));
#37002=DIRECTION('',(-1.,0.,0.));
#37003=DIRECTION('center_axis',(1.,0.,0.));
#37004=DIRECTION('ref_axis',(0.,1.,0.));
#37005=DIRECTION('',(-1.,0.,0.));
#37006=DIRECTION('center_axis',(1.,0.,0.));
#37007=DIRECTION('ref_axis',(0.,1.,0.));
#37008=DIRECTION('',(-1.,0.,0.));
#37009=DIRECTION('center_axis',(1.,0.,0.));
#37010=DIRECTION('ref_axis',(0.,1.,0.));
#37011=DIRECTION('',(-1.,0.,0.));
#37012=DIRECTION('center_axis',(1.,0.,0.));
#37013=DIRECTION('ref_axis',(0.,1.,0.));
#37014=DIRECTION('',(-1.,0.,0.));
#37015=DIRECTION('center_axis',(1.,0.,0.));
#37016=DIRECTION('ref_axis',(0.,1.,0.));
#37017=DIRECTION('',(-1.,0.,0.));
#37018=DIRECTION('center_axis',(1.,0.,0.));
#37019=DIRECTION('ref_axis',(0.,1.,0.));
#37020=DIRECTION('',(-1.,0.,0.));
#37021=DIRECTION('center_axis',(1.,0.,0.));
#37022=DIRECTION('ref_axis',(0.,1.,0.));
#37023=DIRECTION('',(-1.,0.,0.));
#37024=DIRECTION('center_axis',(1.,0.,0.));
#37025=DIRECTION('ref_axis',(0.,1.,0.));
#37026=DIRECTION('',(-1.,0.,0.));
#37027=DIRECTION('center_axis',(1.,0.,0.));
#37028=DIRECTION('ref_axis',(0.,1.,0.));
#37029=DIRECTION('',(-1.,0.,0.));
#37030=DIRECTION('center_axis',(1.,0.,0.));
#37031=DIRECTION('ref_axis',(0.,1.,0.));
#37032=DIRECTION('',(-1.,0.,0.));
#37033=DIRECTION('center_axis',(1.,0.,0.));
#37034=DIRECTION('ref_axis',(0.,1.,0.));
#37035=DIRECTION('',(-1.,0.,0.));
#37036=DIRECTION('center_axis',(1.,0.,0.));
#37037=DIRECTION('ref_axis',(0.,1.,0.));
#37038=DIRECTION('',(-1.,0.,0.));
#37039=DIRECTION('center_axis',(1.,0.,0.));
#37040=DIRECTION('ref_axis',(0.,1.,0.));
#37041=DIRECTION('',(-1.,0.,0.));
#37042=DIRECTION('center_axis',(1.,0.,0.));
#37043=DIRECTION('ref_axis',(0.,1.,0.));
#37044=DIRECTION('',(-1.,0.,0.));
#37045=DIRECTION('center_axis',(1.,0.,0.));
#37046=DIRECTION('ref_axis',(0.,1.,0.));
#37047=DIRECTION('',(-1.,0.,0.));
#37048=DIRECTION('center_axis',(1.,0.,0.));
#37049=DIRECTION('ref_axis',(0.,1.,0.));
#37050=DIRECTION('',(-1.,0.,0.));
#37051=DIRECTION('center_axis',(1.,0.,0.));
#37052=DIRECTION('ref_axis',(0.,1.,0.));
#37053=DIRECTION('',(-1.,0.,0.));
#37054=DIRECTION('center_axis',(1.,0.,0.));
#37055=DIRECTION('ref_axis',(0.,1.,0.));
#37056=DIRECTION('',(-1.,0.,0.));
#37057=DIRECTION('center_axis',(1.,0.,0.));
#37058=DIRECTION('ref_axis',(0.,1.,0.));
#37059=DIRECTION('',(-1.,0.,0.));
#37060=DIRECTION('center_axis',(1.,0.,0.));
#37061=DIRECTION('ref_axis',(0.,1.,0.));
#37062=DIRECTION('',(-1.,0.,0.));
#37063=DIRECTION('center_axis',(1.,0.,0.));
#37064=DIRECTION('ref_axis',(0.,1.,0.));
#37065=DIRECTION('',(-1.,0.,0.));
#37066=DIRECTION('center_axis',(1.,0.,0.));
#37067=DIRECTION('ref_axis',(0.,1.,0.));
#37068=DIRECTION('',(-1.,0.,0.));
#37069=DIRECTION('center_axis',(1.,0.,0.));
#37070=DIRECTION('ref_axis',(0.,1.,0.));
#37071=DIRECTION('',(-1.,0.,0.));
#37072=DIRECTION('center_axis',(1.,0.,0.));
#37073=DIRECTION('ref_axis',(0.,1.,0.));
#37074=DIRECTION('',(-1.,0.,0.));
#37075=DIRECTION('center_axis',(1.,0.,0.));
#37076=DIRECTION('ref_axis',(0.,1.,0.));
#37077=DIRECTION('',(-1.,0.,0.));
#37078=DIRECTION('center_axis',(1.,0.,0.));
#37079=DIRECTION('ref_axis',(0.,-0.266010612903804,-0.963970100066668));
#37080=DIRECTION('',(1.,0.,0.));
#37081=DIRECTION('center_axis',(1.,0.,0.));
#37082=DIRECTION('ref_axis',(0.,1.,-4.74988542142691E-13));
#37083=DIRECTION('center_axis',(1.,0.,0.));
#37084=DIRECTION('ref_axis',(0.,1.,-4.74988542142691E-13));
#37085=DIRECTION('',(1.,0.,0.));
#37086=DIRECTION('center_axis',(1.,0.,0.));
#37087=DIRECTION('ref_axis',(0.,1.,-4.74988542142691E-13));
#37088=DIRECTION('',(1.,0.,0.));
#37089=DIRECTION('center_axis',(1.,0.,0.));
#37090=DIRECTION('ref_axis',(0.,1.,-4.74988542142691E-13));
#37091=DIRECTION('',(1.,0.,0.));
#37092=DIRECTION('center_axis',(1.,0.,0.));
#37093=DIRECTION('ref_axis',(0.,1.,-4.74988542142691E-13));
#37094=DIRECTION('',(1.,0.,0.));
#37095=DIRECTION('center_axis',(1.,0.,0.));
#37096=DIRECTION('ref_axis',(0.,1.,-4.74988542142691E-13));
#37097=DIRECTION('',(1.,0.,0.));
#37098=DIRECTION('center_axis',(1.,0.,0.));
#37099=DIRECTION('ref_axis',(0.,1.,-4.74988542142691E-13));
#37100=DIRECTION('',(1.,0.,0.));
#37101=DIRECTION('center_axis',(1.,0.,0.));
#37102=DIRECTION('ref_axis',(0.,1.,-4.74988542142691E-13));
#37103=DIRECTION('',(1.,0.,0.));
#37104=DIRECTION('center_axis',(1.,0.,0.));
#37105=DIRECTION('ref_axis',(0.,1.,-4.74988542142691E-13));
#37106=DIRECTION('',(1.,0.,0.));
#37107=DIRECTION('center_axis',(1.,0.,0.));
#37108=DIRECTION('ref_axis',(0.,1.,-4.74988542142691E-13));
#37109=DIRECTION('',(1.,0.,0.));
#37110=DIRECTION('center_axis',(1.,0.,0.));
#37111=DIRECTION('ref_axis',(0.,1.,-4.74988542142691E-13));
#37112=DIRECTION('',(1.,0.,0.));
#37113=DIRECTION('center_axis',(1.,0.,0.));
#37114=DIRECTION('ref_axis',(0.,1.,-4.74988542142691E-13));
#37115=DIRECTION('',(1.,0.,0.));
#37116=DIRECTION('center_axis',(1.,0.,0.));
#37117=DIRECTION('ref_axis',(0.,1.,-4.74988542142691E-13));
#37118=DIRECTION('',(1.,0.,0.));
#37119=DIRECTION('center_axis',(1.,0.,0.));
#37120=DIRECTION('ref_axis',(0.,1.,-4.74988542142691E-13));
#37121=DIRECTION('',(1.,0.,0.));
#37122=DIRECTION('center_axis',(1.,0.,0.));
#37123=DIRECTION('ref_axis',(0.,1.,-4.74988542142691E-13));
#37124=DIRECTION('',(1.,0.,0.));
#37125=DIRECTION('center_axis',(1.,0.,0.));
#37126=DIRECTION('ref_axis',(0.,1.,-4.74988542142691E-13));
#37127=DIRECTION('',(1.,0.,0.));
#37128=DIRECTION('center_axis',(1.,0.,0.));
#37129=DIRECTION('ref_axis',(0.,1.,-4.74988542142691E-13));
#37130=DIRECTION('',(1.,0.,0.));
#37131=DIRECTION('center_axis',(1.,0.,0.));
#37132=DIRECTION('ref_axis',(0.,1.,-4.74988542142691E-13));
#37133=DIRECTION('',(1.,0.,0.));
#37134=DIRECTION('center_axis',(1.,0.,0.));
#37135=DIRECTION('ref_axis',(0.,1.,-4.74988542142691E-13));
#37136=DIRECTION('',(1.,0.,0.));
#37137=DIRECTION('center_axis',(1.,0.,0.));
#37138=DIRECTION('ref_axis',(0.,1.,-4.74988542142691E-13));
#37139=DIRECTION('',(1.,0.,0.));
#37140=DIRECTION('center_axis',(1.,0.,0.));
#37141=DIRECTION('ref_axis',(0.,1.,-4.74988542142691E-13));
#37142=DIRECTION('',(1.,0.,0.));
#37143=DIRECTION('center_axis',(1.,0.,0.));
#37144=DIRECTION('ref_axis',(0.,1.,-4.74988542142691E-13));
#37145=DIRECTION('',(1.,0.,0.));
#37146=DIRECTION('center_axis',(1.,0.,0.));
#37147=DIRECTION('ref_axis',(0.,1.,-4.74988542142691E-13));
#37148=DIRECTION('',(1.,0.,0.));
#37149=DIRECTION('center_axis',(1.,0.,0.));
#37150=DIRECTION('ref_axis',(0.,1.,-4.74988542142691E-13));
#37151=DIRECTION('',(1.,0.,0.));
#37152=DIRECTION('center_axis',(1.,0.,0.));
#37153=DIRECTION('ref_axis',(0.,1.,-4.74988542142691E-13));
#37154=DIRECTION('',(1.,0.,0.));
#37155=DIRECTION('center_axis',(1.,0.,0.));
#37156=DIRECTION('ref_axis',(0.,1.,-4.74988542142691E-13));
#37157=DIRECTION('',(1.,0.,0.));
#37158=DIRECTION('center_axis',(1.,0.,0.));
#37159=DIRECTION('ref_axis',(0.,1.,-4.74988542142691E-13));
#37160=DIRECTION('',(1.,0.,0.));
#37161=DIRECTION('center_axis',(1.,0.,0.));
#37162=DIRECTION('ref_axis',(0.,1.,-4.74988542142691E-13));
#37163=DIRECTION('',(1.,0.,0.));
#37164=DIRECTION('center_axis',(1.,0.,0.));
#37165=DIRECTION('ref_axis',(0.,1.,-4.74988542142691E-13));
#37166=DIRECTION('',(1.,0.,0.));
#37167=DIRECTION('center_axis',(1.,0.,0.));
#37168=DIRECTION('ref_axis',(0.,1.,-4.74988542142691E-13));
#37169=DIRECTION('',(1.,0.,0.));
#37170=DIRECTION('center_axis',(1.,0.,0.));
#37171=DIRECTION('ref_axis',(0.,1.,-4.74988542142691E-13));
#37172=DIRECTION('',(1.,0.,0.));
#37173=DIRECTION('center_axis',(1.,0.,0.));
#37174=DIRECTION('ref_axis',(0.,1.,-4.74988542142691E-13));
#37175=DIRECTION('',(1.,0.,0.));
#37176=DIRECTION('center_axis',(1.,0.,0.));
#37177=DIRECTION('ref_axis',(0.,1.,-4.74988542142691E-13));
#37178=DIRECTION('',(1.,0.,0.));
#37179=DIRECTION('center_axis',(1.,0.,0.));
#37180=DIRECTION('ref_axis',(0.,1.,-4.74988542142691E-13));
#37181=DIRECTION('',(1.,0.,0.));
#37182=DIRECTION('center_axis',(1.,0.,0.));
#37183=DIRECTION('ref_axis',(0.,1.,-4.74988542142691E-13));
#37184=DIRECTION('',(1.,0.,0.));
#37185=DIRECTION('center_axis',(1.,0.,0.));
#37186=DIRECTION('ref_axis',(0.,1.,-4.74988542142691E-13));
#37187=DIRECTION('',(1.,0.,0.));
#37188=DIRECTION('center_axis',(1.,0.,0.));
#37189=DIRECTION('ref_axis',(0.,1.,-4.74988542142691E-13));
#37190=DIRECTION('',(1.,0.,0.));
#37191=DIRECTION('center_axis',(1.,0.,0.));
#37192=DIRECTION('ref_axis',(0.,1.,-4.74988542142691E-13));
#37193=DIRECTION('',(1.,0.,0.));
#37194=DIRECTION('center_axis',(1.,0.,0.));
#37195=DIRECTION('ref_axis',(0.,1.,-4.74988542142691E-13));
#37196=DIRECTION('',(1.,0.,0.));
#37197=DIRECTION('center_axis',(1.,0.,0.));
#37198=DIRECTION('ref_axis',(0.,1.,-4.74988542142691E-13));
#37199=DIRECTION('',(1.,0.,0.));
#37200=DIRECTION('center_axis',(1.,0.,0.));
#37201=DIRECTION('ref_axis',(0.,1.,-4.74988542142691E-13));
#37202=DIRECTION('',(1.,0.,0.));
#37203=DIRECTION('center_axis',(1.,0.,0.));
#37204=DIRECTION('ref_axis',(0.,1.,-4.74988542142691E-13));
#37205=DIRECTION('',(1.,0.,0.));
#37206=DIRECTION('center_axis',(1.,0.,0.));
#37207=DIRECTION('ref_axis',(0.,0.,-1.));
#37208=DIRECTION('center_axis',(1.,0.,0.));
#37209=DIRECTION('ref_axis',(0.,1.,0.));
#37210=DIRECTION('center_axis',(1.,0.,0.));
#37211=DIRECTION('ref_axis',(0.,0.,-1.));
#37212=DIRECTION('center_axis',(1.,0.,0.));
#37213=DIRECTION('ref_axis',(0.,1.,0.));
#37214=DIRECTION('center_axis',(1.,0.,0.));
#37215=DIRECTION('ref_axis',(0.,1.,0.));
#37216=DIRECTION('center_axis',(-1.,0.,0.));
#37217=DIRECTION('ref_axis',(0.,1.,-4.74988542142691E-13));
#37218=DIRECTION('center_axis',(1.,0.,0.));
#37219=DIRECTION('ref_axis',(0.,1.,-4.74988542142691E-13));
#37220=DIRECTION('center_axis',(1.,0.,0.));
#37221=DIRECTION('ref_axis',(0.,0.,-1.));
#37222=DIRECTION('center_axis',(1.,0.,0.));
#37223=DIRECTION('ref_axis',(0.,1.,0.));
#37224=DIRECTION('center_axis',(0.,-1.,-1.22464679914735E-16));
#37225=DIRECTION('ref_axis',(0.,-1.22464679914735E-16,1.));
#37226=DIRECTION('center_axis',(-1.,0.,0.));
#37227=DIRECTION('ref_axis',(0.,1.,0.));
#37228=DIRECTION('center_axis',(1.,0.,0.));
#37229=DIRECTION('ref_axis',(0.,1.,0.));
#37230=DIRECTION('center_axis',(1.,0.,0.));
#37231=DIRECTION('ref_axis',(0.,0.939072950732287,-0.343717897705305));
#37232=DIRECTION('center_axis',(-1.,0.,0.));
#37233=DIRECTION('ref_axis',(0.,0.,1.));
#37234=DIRECTION('center_axis',(1.,0.,0.));
#37235=DIRECTION('ref_axis',(0.,0.,-1.));
#37236=DIRECTION('center_axis',(0.,-0.443490878258564,0.896278885672003));
#37237=DIRECTION('ref_axis',(0.,-0.896278885672003,-0.443490878258564));
#37238=DIRECTION('',(-1.,0.,0.));
#37239=DIRECTION('',(0.,-0.896278885672003,-0.443490878258564));
#37240=DIRECTION('',(1.,0.,0.));
#37241=DIRECTION('',(0.,-0.896278885672003,-0.443490878258564));
#37242=DIRECTION('center_axis',(1.,0.,0.));
#37243=DIRECTION('ref_axis',(0.,-0.17364817766693,-0.984807753012208));
#37244=DIRECTION('center_axis',(-1.,0.,0.));
#37245=DIRECTION('ref_axis',(0.,1.,0.));
#37246=DIRECTION('',(0.,0.690543841286577,-0.723290538622744));
#37247=DIRECTION('center_axis',(0.,-0.723290538622744,-0.690543841286577));
#37248=DIRECTION('ref_axis',(0.,0.690543841286577,-0.723290538622744));
#37249=DIRECTION('',(1.,0.,0.));
#37250=DIRECTION('',(0.,0.690543841286577,-0.723290538622744));
#37251=DIRECTION('center_axis',(1.,0.,0.));
#37252=DIRECTION('ref_axis',(0.,-0.17364817766693,-0.984807753012208));
#37253=DIRECTION('center_axis',(1.,0.,0.));
#37254=DIRECTION('ref_axis',(0.,1.,0.));
#37255=DIRECTION('center_axis',(0.,-0.281116060120936,0.959673778292437));
#37256=DIRECTION('ref_axis',(0.,-0.959673778292437,-0.281116060120936));
#37257=DIRECTION('',(-1.,0.,0.));
#37258=DIRECTION('',(0.,-0.959673778292437,-0.281116060120936));
#37259=DIRECTION('',(1.,0.,0.));
#37260=DIRECTION('',(0.,-0.959673778292437,-0.281116060120936));
#37261=DIRECTION('center_axis',(1.,0.,0.));
#37262=DIRECTION('ref_axis',(0.,-0.342020143325669,-0.939692620785908));
#37263=DIRECTION('center_axis',(-1.,0.,0.));
#37264=DIRECTION('ref_axis',(0.,1.,0.));
#37265=DIRECTION('',(0.,0.55445484473828,-0.83221380975459));
#37266=DIRECTION('center_axis',(0.,-0.83221380975459,-0.55445484473828));
#37267=DIRECTION('ref_axis',(0.,0.55445484473828,-0.83221380975459));
#37268=DIRECTION('',(1.,0.,0.));
#37269=DIRECTION('',(0.,0.55445484473828,-0.83221380975459));
#37270=DIRECTION('center_axis',(1.,0.,0.));
#37271=DIRECTION('ref_axis',(0.,-0.342020143325669,-0.939692620785908));
#37272=DIRECTION('center_axis',(1.,0.,0.));
#37273=DIRECTION('ref_axis',(0.,1.,0.));
#37274=DIRECTION('center_axis',(0.,-0.110199672748125,0.993909468777819));
#37275=DIRECTION('ref_axis',(0.,-0.993909468777819,-0.110199672748125));
#37276=DIRECTION('',(-1.,0.,0.));
#37277=DIRECTION('',(0.,-0.993909468777819,-0.110199672748125));
#37278=DIRECTION('',(1.,0.,0.));
#37279=DIRECTION('',(0.,-0.993909468777819,-0.110199672748125));
#37280=DIRECTION('center_axis',(1.,0.,0.));
#37281=DIRECTION('ref_axis',(0.,-0.5,-0.866025403784438));
#37282=DIRECTION('center_axis',(-1.,0.,0.));
#37283=DIRECTION('ref_axis',(0.,1.,0.));
#37284=DIRECTION('',(0.,0.401519018300301,-0.91585068539755));
#37285=DIRECTION('center_axis',(0.,-0.91585068539755,-0.401519018300301));
#37286=DIRECTION('ref_axis',(0.,0.401519018300301,-0.91585068539755));
#37287=DIRECTION('',(1.,0.,0.));
#37288=DIRECTION('',(0.,0.401519018300301,-0.91585068539755));
#37289=DIRECTION('center_axis',(1.,0.,0.));
#37290=DIRECTION('ref_axis',(0.,-0.5,-0.866025403784438));
#37291=DIRECTION('center_axis',(1.,0.,0.));
#37292=DIRECTION('ref_axis',(0.,1.,0.));
#37293=DIRECTION('center_axis',(0.,0.0640650759174134,0.997945722996845));
#37294=DIRECTION('ref_axis',(0.,-0.997945722996845,0.0640650759174133));
#37295=DIRECTION('',(-1.,0.,0.));
#37296=DIRECTION('',(0.,-0.997945722996845,0.0640650759174133));
#37297=DIRECTION('',(1.,0.,0.));
#37298=DIRECTION('',(0.,-0.997945722996845,0.0640650759174133));
#37299=DIRECTION('center_axis',(1.,0.,0.));
#37300=DIRECTION('ref_axis',(0.,-0.64278760968654,-0.766044443118978));
#37301=DIRECTION('center_axis',(-1.,0.,0.));
#37302=DIRECTION('ref_axis',(0.,1.,0.));
#37303=DIRECTION('',(0.,0.236383239669693,-0.971659901407514));
#37304=DIRECTION('center_axis',(0.,-0.971659901407514,-0.236383239669693));
#37305=DIRECTION('ref_axis',(0.,0.236383239669693,-0.971659901407514));
#37306=DIRECTION('',(1.,0.,0.));
#37307=DIRECTION('',(0.,0.236383239669693,-0.971659901407514));
#37308=DIRECTION('center_axis',(1.,0.,0.));
#37309=DIRECTION('ref_axis',(0.,-0.64278760968654,-0.766044443118978));
#37310=DIRECTION('center_axis',(1.,0.,0.));
#37311=DIRECTION('ref_axis',(0.,1.,0.));
#37312=DIRECTION('center_axis',(0.,0.236383239669694,0.971659901407514));
#37313=DIRECTION('ref_axis',(0.,-0.971659901407514,0.236383239669694));
#37314=DIRECTION('',(-1.,0.,0.));
#37315=DIRECTION('',(0.,-0.971659901407514,0.236383239669694));
#37316=DIRECTION('',(1.,0.,0.));
#37317=DIRECTION('',(0.,-0.971659901407514,0.236383239669694));
#37318=DIRECTION('center_axis',(1.,0.,0.));
#37319=DIRECTION('ref_axis',(0.,-0.766044443118978,-0.642787609686539));
#37320=DIRECTION('center_axis',(-1.,0.,0.));
#37321=DIRECTION('ref_axis',(0.,1.,0.));
#37322=DIRECTION('',(0.,0.0640650759174129,-0.997945722996845));
#37323=DIRECTION('center_axis',(0.,-0.997945722996845,-0.0640650759174129));
#37324=DIRECTION('ref_axis',(0.,0.0640650759174129,-0.997945722996845));
#37325=DIRECTION('',(1.,0.,0.));
#37326=DIRECTION('',(0.,0.0640650759174129,-0.997945722996845));
#37327=DIRECTION('center_axis',(1.,0.,0.));
#37328=DIRECTION('ref_axis',(0.,-0.766044443118978,-0.642787609686539));
#37329=DIRECTION('center_axis',(1.,0.,0.));
#37330=DIRECTION('ref_axis',(0.,1.,0.));
#37331=DIRECTION('center_axis',(0.,0.401519018300301,0.91585068539755));
#37332=DIRECTION('ref_axis',(0.,-0.91585068539755,0.401519018300301));
#37333=DIRECTION('',(-1.,0.,0.));
#37334=DIRECTION('',(0.,-0.91585068539755,0.401519018300301));
#37335=DIRECTION('',(1.,0.,0.));
#37336=DIRECTION('',(0.,-0.91585068539755,0.401519018300301));
#37337=DIRECTION('center_axis',(1.,0.,0.));
#37338=DIRECTION('ref_axis',(0.,-0.866025403784439,-0.5));
#37339=DIRECTION('center_axis',(-1.,0.,0.));
#37340=DIRECTION('ref_axis',(0.,1.,0.));
#37341=DIRECTION('',(0.,-0.110199672748125,-0.993909468777819));
#37342=DIRECTION('center_axis',(0.,-0.993909468777819,0.110199672748125));
#37343=DIRECTION('ref_axis',(0.,-0.110199672748125,-0.993909468777819));
#37344=DIRECTION('',(1.,0.,0.));
#37345=DIRECTION('',(0.,-0.110199672748125,-0.993909468777819));
#37346=DIRECTION('center_axis',(1.,0.,0.));
#37347=DIRECTION('ref_axis',(0.,-0.866025403784439,-0.5));
#37348=DIRECTION('center_axis',(1.,0.,0.));
#37349=DIRECTION('ref_axis',(0.,1.,0.));
#37350=DIRECTION('center_axis',(0.,0.554454844738281,0.83221380975459));
#37351=DIRECTION('ref_axis',(0.,-0.83221380975459,0.554454844738281));
#37352=DIRECTION('',(-1.,0.,0.));
#37353=DIRECTION('',(0.,-0.83221380975459,0.554454844738281));
#37354=DIRECTION('',(1.,0.,0.));
#37355=DIRECTION('',(0.,-0.83221380975459,0.554454844738281));
#37356=DIRECTION('center_axis',(1.,0.,0.));
#37357=DIRECTION('ref_axis',(0.,-0.939692620785909,-0.342020143325668));
#37358=DIRECTION('center_axis',(-1.,0.,0.));
#37359=DIRECTION('ref_axis',(0.,1.,0.));
#37360=DIRECTION('',(0.,-0.281116060120938,-0.959673778292437));
#37361=DIRECTION('center_axis',(0.,-0.959673778292437,0.281116060120938));
#37362=DIRECTION('ref_axis',(0.,-0.281116060120938,-0.959673778292437));
#37363=DIRECTION('',(1.,0.,0.));
#37364=DIRECTION('',(0.,-0.281116060120938,-0.959673778292437));
#37365=DIRECTION('center_axis',(1.,0.,0.));
#37366=DIRECTION('ref_axis',(0.,-0.939692620785909,-0.342020143325668));
#37367=DIRECTION('center_axis',(1.,0.,0.));
#37368=DIRECTION('ref_axis',(0.,1.,0.));
#37369=DIRECTION('center_axis',(0.,0.690543841286578,0.723290538622743));
#37370=DIRECTION('ref_axis',(0.,-0.723290538622743,0.690543841286577));
#37371=DIRECTION('',(-1.,0.,0.));
#37372=DIRECTION('',(0.,-0.723290538622743,0.690543841286577));
#37373=DIRECTION('',(1.,0.,0.));
#37374=DIRECTION('',(0.,-0.723290538622743,0.690543841286577));
#37375=DIRECTION('center_axis',(1.,0.,0.));
#37376=DIRECTION('ref_axis',(0.,-0.984807753012208,-0.17364817766693));
#37377=DIRECTION('center_axis',(-1.,0.,0.));
#37378=DIRECTION('ref_axis',(0.,1.,0.));
#37379=DIRECTION('',(0.,-0.443490878258565,-0.896278885672003));
#37380=DIRECTION('center_axis',(0.,-0.896278885672003,0.443490878258565));
#37381=DIRECTION('ref_axis',(0.,-0.443490878258565,-0.896278885672003));
#37382=DIRECTION('',(1.,0.,0.));
#37383=DIRECTION('',(0.,-0.443490878258565,-0.896278885672003));
#37384=DIRECTION('center_axis',(1.,0.,0.));
#37385=DIRECTION('ref_axis',(0.,-0.984807753012208,-0.17364817766693));
#37386=DIRECTION('center_axis',(1.,0.,0.));
#37387=DIRECTION('ref_axis',(0.,1.,0.));
#37388=DIRECTION('center_axis',(0.,0.805651012649425,0.592390450477518));
#37389=DIRECTION('ref_axis',(0.,-0.592390450477518,0.805651012649425));
#37390=DIRECTION('',(-1.,0.,0.));
#37391=DIRECTION('',(0.,-0.592390450477518,0.805651012649425));
#37392=DIRECTION('',(1.,0.,0.));
#37393=DIRECTION('',(0.,-0.592390450477518,0.805651012649425));
#37394=DIRECTION('center_axis',(1.,0.,0.));
#37395=DIRECTION('ref_axis',(0.,-1.,1.83697019872103E-16));
#37396=DIRECTION('center_axis',(-1.,0.,0.));
#37397=DIRECTION('ref_axis',(0.,1.,0.));
#37398=DIRECTION('',(0.,-0.592390450477518,-0.805651012649425));
#37399=DIRECTION('center_axis',(0.,-0.805651012649425,0.592390450477518));
#37400=DIRECTION('ref_axis',(0.,-0.592390450477518,-0.805651012649425));
#37401=DIRECTION('',(1.,0.,0.));
#37402=DIRECTION('',(0.,-0.592390450477518,-0.805651012649425));
#37403=DIRECTION('center_axis',(1.,0.,0.));
#37404=DIRECTION('ref_axis',(0.,-1.,1.83697019872103E-16));
#37405=DIRECTION('center_axis',(1.,0.,0.));
#37406=DIRECTION('ref_axis',(0.,1.,0.));
#37407=DIRECTION('center_axis',(0.,0.896278885672003,0.443490878258564));
#37408=DIRECTION('ref_axis',(0.,-0.443490878258564,0.896278885672003));
#37409=DIRECTION('',(-1.,0.,0.));
#37410=DIRECTION('',(0.,-0.443490878258564,0.896278885672003));
#37411=DIRECTION('',(1.,0.,0.));
#37412=DIRECTION('',(0.,-0.443490878258564,0.896278885672003));
#37413=DIRECTION('center_axis',(1.,0.,0.));
#37414=DIRECTION('ref_axis',(0.,-0.984807753012208,0.17364817766693));
#37415=DIRECTION('center_axis',(-1.,0.,0.));
#37416=DIRECTION('ref_axis',(0.,1.,0.));
#37417=DIRECTION('',(0.,-0.723290538622744,-0.690543841286577));
#37418=DIRECTION('center_axis',(0.,-0.690543841286577,0.723290538622744));
#37419=DIRECTION('ref_axis',(0.,-0.723290538622744,-0.690543841286577));
#37420=DIRECTION('',(1.,0.,0.));
#37421=DIRECTION('',(0.,-0.723290538622744,-0.690543841286577));
#37422=DIRECTION('center_axis',(1.,0.,0.));
#37423=DIRECTION('ref_axis',(0.,-0.984807753012208,0.17364817766693));
#37424=DIRECTION('center_axis',(1.,0.,0.));
#37425=DIRECTION('ref_axis',(0.,1.,0.));
#37426=DIRECTION('center_axis',(0.,0.959673778292437,0.281116060120936));
#37427=DIRECTION('ref_axis',(0.,-0.281116060120936,0.959673778292437));
#37428=DIRECTION('',(-1.,0.,0.));
#37429=DIRECTION('',(0.,-0.281116060120936,0.959673778292437));
#37430=DIRECTION('',(1.,0.,0.));
#37431=DIRECTION('',(0.,-0.281116060120936,0.959673778292437));
#37432=DIRECTION('center_axis',(1.,0.,0.));
#37433=DIRECTION('ref_axis',(0.,-0.939692620785908,0.342020143325669));
#37434=DIRECTION('center_axis',(-1.,0.,0.));
#37435=DIRECTION('ref_axis',(0.,1.,0.));
#37436=DIRECTION('',(0.,-0.83221380975459,-0.55445484473828));
#37437=DIRECTION('center_axis',(0.,-0.55445484473828,0.83221380975459));
#37438=DIRECTION('ref_axis',(0.,-0.83221380975459,-0.55445484473828));
#37439=DIRECTION('',(1.,0.,0.));
#37440=DIRECTION('',(0.,-0.83221380975459,-0.55445484473828));
#37441=DIRECTION('center_axis',(1.,0.,0.));
#37442=DIRECTION('ref_axis',(0.,-0.939692620785908,0.342020143325669));
#37443=DIRECTION('center_axis',(1.,0.,0.));
#37444=DIRECTION('ref_axis',(0.,1.,0.));
#37445=DIRECTION('center_axis',(0.,0.993909468777819,0.110199672748125));
#37446=DIRECTION('ref_axis',(0.,-0.110199672748125,0.993909468777819));
#37447=DIRECTION('',(-1.,0.,0.));
#37448=DIRECTION('',(0.,-0.110199672748125,0.993909468777819));
#37449=DIRECTION('',(1.,0.,0.));
#37450=DIRECTION('',(0.,-0.110199672748125,0.993909468777819));
#37451=DIRECTION('center_axis',(1.,0.,0.));
#37452=DIRECTION('ref_axis',(0.,-0.866025403784438,0.5));
#37453=DIRECTION('center_axis',(-1.,0.,0.));
#37454=DIRECTION('ref_axis',(0.,1.,0.));
#37455=DIRECTION('',(0.,-0.91585068539755,-0.401519018300301));
#37456=DIRECTION('center_axis',(0.,-0.401519018300301,0.91585068539755));
#37457=DIRECTION('ref_axis',(0.,-0.91585068539755,-0.401519018300301));
#37458=DIRECTION('',(1.,0.,0.));
#37459=DIRECTION('',(0.,-0.91585068539755,-0.401519018300301));
#37460=DIRECTION('center_axis',(1.,0.,0.));
#37461=DIRECTION('ref_axis',(0.,-0.866025403784438,0.5));
#37462=DIRECTION('center_axis',(1.,0.,0.));
#37463=DIRECTION('ref_axis',(0.,1.,0.));
#37464=DIRECTION('center_axis',(0.,0.997945722996845,-0.0640650759174131));
#37465=DIRECTION('ref_axis',(0.,0.0640650759174131,0.997945722996845));
#37466=DIRECTION('',(-1.,0.,0.));
#37467=DIRECTION('',(0.,0.0640650759174131,0.997945722996845));
#37468=DIRECTION('',(1.,0.,0.));
#37469=DIRECTION('',(0.,0.0640650759174131,0.997945722996845));
#37470=DIRECTION('center_axis',(1.,0.,0.));
#37471=DIRECTION('ref_axis',(0.,-0.766044443118978,0.642787609686539));
#37472=DIRECTION('center_axis',(-1.,0.,0.));
#37473=DIRECTION('ref_axis',(0.,1.,0.));
#37474=DIRECTION('',(0.,-0.971659901407514,-0.236383239669693));
#37475=DIRECTION('center_axis',(0.,-0.236383239669693,0.971659901407514));
#37476=DIRECTION('ref_axis',(0.,-0.971659901407514,-0.236383239669693));
#37477=DIRECTION('',(1.,0.,0.));
#37478=DIRECTION('',(0.,-0.971659901407514,-0.236383239669693));
#37479=DIRECTION('center_axis',(1.,0.,0.));
#37480=DIRECTION('ref_axis',(0.,-0.766044443118978,0.642787609686539));
#37481=DIRECTION('center_axis',(1.,0.,0.));
#37482=DIRECTION('ref_axis',(0.,1.,0.));
#37483=DIRECTION('center_axis',(0.,0.971659901407514,-0.236383239669694));
#37484=DIRECTION('ref_axis',(0.,0.236383239669694,0.971659901407514));
#37485=DIRECTION('',(-1.,0.,0.));
#37486=DIRECTION('',(0.,0.236383239669694,0.971659901407514));
#37487=DIRECTION('',(1.,0.,0.));
#37488=DIRECTION('',(0.,0.236383239669694,0.971659901407514));
#37489=DIRECTION('center_axis',(1.,0.,0.));
#37490=DIRECTION('ref_axis',(0.,-0.642787609686539,0.766044443118978));
#37491=DIRECTION('center_axis',(-1.,0.,0.));
#37492=DIRECTION('ref_axis',(0.,1.,0.));
#37493=DIRECTION('',(0.,-0.997945722996845,-0.064065075917413));
#37494=DIRECTION('center_axis',(0.,-0.064065075917413,0.997945722996845));
#37495=DIRECTION('ref_axis',(0.,-0.997945722996845,-0.064065075917413));
#37496=DIRECTION('',(1.,0.,0.));
#37497=DIRECTION('',(0.,-0.997945722996845,-0.064065075917413));
#37498=DIRECTION('center_axis',(1.,0.,0.));
#37499=DIRECTION('ref_axis',(0.,-0.642787609686539,0.766044443118978));
#37500=DIRECTION('center_axis',(1.,0.,0.));
#37501=DIRECTION('ref_axis',(0.,1.,0.));
#37502=DIRECTION('center_axis',(0.,0.91585068539755,-0.401519018300301));
#37503=DIRECTION('ref_axis',(0.,0.401519018300301,0.91585068539755));
#37504=DIRECTION('',(-1.,0.,0.));
#37505=DIRECTION('',(0.,0.401519018300301,0.91585068539755));
#37506=DIRECTION('',(1.,0.,0.));
#37507=DIRECTION('',(0.,0.401519018300301,0.91585068539755));
#37508=DIRECTION('center_axis',(1.,0.,0.));
#37509=DIRECTION('ref_axis',(0.,-0.5,0.866025403784439));
#37510=DIRECTION('center_axis',(-1.,0.,0.));
#37511=DIRECTION('ref_axis',(0.,1.,0.));
#37512=DIRECTION('',(0.,-0.993909468777819,0.110199672748126));
#37513=DIRECTION('center_axis',(0.,0.110199672748126,0.993909468777819));
#37514=DIRECTION('ref_axis',(0.,-0.993909468777819,0.110199672748126));
#37515=DIRECTION('',(1.,0.,0.));
#37516=DIRECTION('',(0.,-0.993909468777819,0.110199672748126));
#37517=DIRECTION('center_axis',(1.,0.,0.));
#37518=DIRECTION('ref_axis',(0.,-0.5,0.866025403784439));
#37519=DIRECTION('center_axis',(1.,0.,0.));
#37520=DIRECTION('ref_axis',(0.,1.,0.));
#37521=DIRECTION('center_axis',(0.,0.83221380975459,-0.554454844738281));
#37522=DIRECTION('ref_axis',(0.,0.554454844738281,0.83221380975459));
#37523=DIRECTION('',(-1.,0.,0.));
#37524=DIRECTION('',(0.,0.554454844738281,0.83221380975459));
#37525=DIRECTION('',(1.,0.,0.));
#37526=DIRECTION('',(0.,0.554454844738281,0.83221380975459));
#37527=DIRECTION('center_axis',(1.,0.,0.));
#37528=DIRECTION('ref_axis',(0.,-0.342020143325669,0.939692620785909));
#37529=DIRECTION('center_axis',(-1.,0.,0.));
#37530=DIRECTION('ref_axis',(0.,1.,0.));
#37531=DIRECTION('',(0.,-0.959673778292437,0.281116060120937));
#37532=DIRECTION('center_axis',(0.,0.281116060120937,0.959673778292437));
#37533=DIRECTION('ref_axis',(0.,-0.959673778292437,0.281116060120937));
#37534=DIRECTION('',(1.,0.,0.));
#37535=DIRECTION('',(0.,-0.959673778292437,0.281116060120937));
#37536=DIRECTION('center_axis',(1.,0.,0.));
#37537=DIRECTION('ref_axis',(0.,-0.342020143325669,0.939692620785909));
#37538=DIRECTION('center_axis',(1.,0.,0.));
#37539=DIRECTION('ref_axis',(0.,1.,0.));
#37540=DIRECTION('center_axis',(0.,0.723290538622743,-0.690543841286577));
#37541=DIRECTION('ref_axis',(0.,0.690543841286577,0.723290538622743));
#37542=DIRECTION('',(-1.,0.,0.));
#37543=DIRECTION('',(0.,0.690543841286577,0.723290538622743));
#37544=DIRECTION('',(1.,0.,0.));
#37545=DIRECTION('',(0.,0.690543841286577,0.723290538622743));
#37546=DIRECTION('center_axis',(1.,0.,0.));
#37547=DIRECTION('ref_axis',(0.,-0.17364817766693,0.984807753012208));
#37548=DIRECTION('center_axis',(-1.,0.,0.));
#37549=DIRECTION('ref_axis',(0.,1.,0.));
#37550=DIRECTION('',(0.,-0.896278885672003,0.443490878258565));
#37551=DIRECTION('center_axis',(0.,0.443490878258565,0.896278885672003));
#37552=DIRECTION('ref_axis',(0.,-0.896278885672003,0.443490878258565));
#37553=DIRECTION('',(1.,0.,0.));
#37554=DIRECTION('',(0.,-0.896278885672003,0.443490878258565));
#37555=DIRECTION('center_axis',(1.,0.,0.));
#37556=DIRECTION('ref_axis',(0.,-0.17364817766693,0.984807753012208));
#37557=DIRECTION('center_axis',(1.,0.,0.));
#37558=DIRECTION('ref_axis',(0.,1.,0.));
#37559=DIRECTION('center_axis',(0.,0.592390450477518,-0.805651012649425));
#37560=DIRECTION('ref_axis',(0.,0.805651012649425,0.592390450477518));
#37561=DIRECTION('',(-1.,0.,0.));
#37562=DIRECTION('',(0.,0.805651012649425,0.592390450477518));
#37563=DIRECTION('',(1.,0.,0.));
#37564=DIRECTION('',(0.,0.805651012649425,0.592390450477518));
#37565=DIRECTION('center_axis',(1.,0.,0.));
#37566=DIRECTION('ref_axis',(0.,1.22464679914735E-16,1.));
#37567=DIRECTION('center_axis',(-1.,0.,0.));
#37568=DIRECTION('ref_axis',(0.,1.,0.));
#37569=DIRECTION('',(0.,-0.805651012649425,0.592390450477518));
#37570=DIRECTION('center_axis',(-1.,0.,0.));
#37571=DIRECTION('ref_axis',(0.,1.,0.));
#37572=DIRECTION('center_axis',(0.,0.592390450477518,0.805651012649425));
#37573=DIRECTION('ref_axis',(0.,-0.805651012649425,0.592390450477518));
#37574=DIRECTION('',(1.,0.,0.));
#37575=DIRECTION('',(0.,-0.805651012649425,0.592390450477518));
#37576=DIRECTION('center_axis',(1.,0.,0.));
#37577=DIRECTION('ref_axis',(0.,1.22464679914735E-16,1.));
#37578=DIRECTION('center_axis',(1.,0.,0.));
#37579=DIRECTION('ref_axis',(0.,1.,0.));
#37580=DIRECTION('center_axis',(1.,0.,0.));
#37581=DIRECTION('ref_axis',(0.,1.,0.));
#37582=DIRECTION('center_axis',(0.,0.443490878258564,-0.896278885672003));
#37583=DIRECTION('ref_axis',(0.,0.896278885672003,0.443490878258564));
#37584=DIRECTION('',(-1.,0.,0.));
#37585=DIRECTION('',(0.,0.896278885672003,0.443490878258564));
#37586=DIRECTION('',(1.,0.,0.));
#37587=DIRECTION('',(0.,0.896278885672003,0.443490878258564));
#37588=DIRECTION('center_axis',(1.,0.,0.));
#37589=DIRECTION('ref_axis',(0.,0.173648177666931,0.984807753012208));
#37590=DIRECTION('center_axis',(-1.,0.,0.));
#37591=DIRECTION('ref_axis',(0.,1.,0.));
#37592=DIRECTION('',(0.,-0.690543841286577,0.723290538622744));
#37593=DIRECTION('center_axis',(0.,0.723290538622744,0.690543841286577));
#37594=DIRECTION('ref_axis',(0.,-0.690543841286577,0.723290538622744));
#37595=DIRECTION('',(1.,0.,0.));
#37596=DIRECTION('',(0.,-0.690543841286577,0.723290538622744));
#37597=DIRECTION('center_axis',(1.,0.,0.));
#37598=DIRECTION('ref_axis',(0.,0.173648177666931,0.984807753012208));
#37599=DIRECTION('center_axis',(1.,0.,0.));
#37600=DIRECTION('ref_axis',(0.,1.,0.));
#37601=DIRECTION('center_axis',(0.,0.281116060120937,-0.959673778292437));
#37602=DIRECTION('ref_axis',(0.,0.959673778292437,0.281116060120937));
#37603=DIRECTION('',(-1.,0.,0.));
#37604=DIRECTION('',(0.,0.959673778292437,0.281116060120937));
#37605=DIRECTION('',(1.,0.,0.));
#37606=DIRECTION('',(0.,0.959673778292437,0.281116060120937));
#37607=DIRECTION('center_axis',(1.,0.,0.));
#37608=DIRECTION('ref_axis',(0.,0.342020143325669,0.939692620785908));
#37609=DIRECTION('center_axis',(-1.,0.,0.));
#37610=DIRECTION('ref_axis',(0.,1.,0.));
#37611=DIRECTION('',(0.,-0.554454844738281,0.83221380975459));
#37612=DIRECTION('center_axis',(0.,0.83221380975459,0.554454844738281));
#37613=DIRECTION('ref_axis',(0.,-0.554454844738281,0.83221380975459));
#37614=DIRECTION('',(1.,0.,0.));
#37615=DIRECTION('',(0.,-0.554454844738281,0.83221380975459));
#37616=DIRECTION('center_axis',(1.,0.,0.));
#37617=DIRECTION('ref_axis',(0.,0.342020143325669,0.939692620785908));
#37618=DIRECTION('center_axis',(1.,0.,0.));
#37619=DIRECTION('ref_axis',(0.,1.,0.));
#37620=DIRECTION('center_axis',(0.,0.110199672748126,-0.993909468777819));
#37621=DIRECTION('ref_axis',(0.,0.993909468777819,0.110199672748126));
#37622=DIRECTION('',(-1.,0.,0.));
#37623=DIRECTION('',(0.,0.993909468777819,0.110199672748126));
#37624=DIRECTION('',(1.,0.,0.));
#37625=DIRECTION('',(0.,0.993909468777819,0.110199672748126));
#37626=DIRECTION('center_axis',(1.,0.,0.));
#37627=DIRECTION('ref_axis',(0.,0.5,0.866025403784439));
#37628=DIRECTION('center_axis',(-1.,0.,0.));
#37629=DIRECTION('ref_axis',(0.,1.,0.));
#37630=DIRECTION('',(0.,-0.401519018300301,0.91585068539755));
#37631=DIRECTION('center_axis',(0.,0.91585068539755,0.401519018300301));
#37632=DIRECTION('ref_axis',(0.,-0.401519018300301,0.91585068539755));
#37633=DIRECTION('',(1.,0.,0.));
#37634=DIRECTION('',(0.,-0.401519018300301,0.91585068539755));
#37635=DIRECTION('center_axis',(1.,0.,0.));
#37636=DIRECTION('ref_axis',(0.,0.5,0.866025403784439));
#37637=DIRECTION('center_axis',(1.,0.,0.));
#37638=DIRECTION('ref_axis',(0.,1.,0.));
#37639=DIRECTION('center_axis',(0.,-0.0640650759174131,-0.997945722996845));
#37640=DIRECTION('ref_axis',(0.,0.997945722996845,-0.0640650759174131));
#37641=DIRECTION('',(-1.,0.,0.));
#37642=DIRECTION('',(0.,0.997945722996845,-0.0640650759174131));
#37643=DIRECTION('',(1.,0.,0.));
#37644=DIRECTION('',(0.,0.997945722996845,-0.0640650759174131));
#37645=DIRECTION('center_axis',(1.,0.,0.));
#37646=DIRECTION('ref_axis',(0.,0.642787609686539,0.766044443118978));
#37647=DIRECTION('center_axis',(-1.,0.,0.));
#37648=DIRECTION('ref_axis',(0.,1.,0.));
#37649=DIRECTION('',(0.,-0.236383239669693,0.971659901407514));
#37650=DIRECTION('center_axis',(0.,0.971659901407514,0.236383239669693));
#37651=DIRECTION('ref_axis',(0.,-0.236383239669693,0.971659901407514));
#37652=DIRECTION('',(1.,0.,0.));
#37653=DIRECTION('',(0.,-0.236383239669693,0.971659901407514));
#37654=DIRECTION('center_axis',(1.,0.,0.));
#37655=DIRECTION('ref_axis',(0.,0.642787609686539,0.766044443118978));
#37656=DIRECTION('center_axis',(1.,0.,0.));
#37657=DIRECTION('ref_axis',(0.,1.,0.));
#37658=DIRECTION('center_axis',(0.,-0.236383239669693,-0.971659901407514));
#37659=DIRECTION('ref_axis',(0.,0.971659901407514,-0.236383239669693));
#37660=DIRECTION('',(-1.,0.,0.));
#37661=DIRECTION('',(0.,0.971659901407514,-0.236383239669693));
#37662=DIRECTION('',(1.,0.,0.));
#37663=DIRECTION('',(0.,0.971659901407514,-0.236383239669693));
#37664=DIRECTION('center_axis',(1.,0.,0.));
#37665=DIRECTION('ref_axis',(0.,0.766044443118978,0.642787609686539));
#37666=DIRECTION('center_axis',(-1.,0.,0.));
#37667=DIRECTION('ref_axis',(0.,1.,0.));
#37668=DIRECTION('',(0.,-0.0640650759174131,0.997945722996845));
#37669=DIRECTION('center_axis',(0.,0.997945722996845,0.0640650759174131));
#37670=DIRECTION('ref_axis',(0.,-0.0640650759174131,0.997945722996845));
#37671=DIRECTION('',(1.,0.,0.));
#37672=DIRECTION('',(0.,-0.0640650759174131,0.997945722996845));
#37673=DIRECTION('center_axis',(1.,0.,0.));
#37674=DIRECTION('ref_axis',(0.,0.766044443118978,0.642787609686539));
#37675=DIRECTION('center_axis',(1.,0.,0.));
#37676=DIRECTION('ref_axis',(0.,1.,0.));
#37677=DIRECTION('center_axis',(0.,-0.401519018300301,-0.91585068539755));
#37678=DIRECTION('ref_axis',(0.,0.91585068539755,-0.401519018300301));
#37679=DIRECTION('',(-1.,0.,0.));
#37680=DIRECTION('',(0.,0.91585068539755,-0.401519018300301));
#37681=DIRECTION('',(1.,0.,0.));
#37682=DIRECTION('',(0.,0.91585068539755,-0.401519018300301));
#37683=DIRECTION('center_axis',(1.,0.,0.));
#37684=DIRECTION('ref_axis',(0.,0.866025403784439,0.5));
#37685=DIRECTION('center_axis',(-1.,0.,0.));
#37686=DIRECTION('ref_axis',(0.,1.,0.));
#37687=DIRECTION('',(0.,0.110199672748126,0.993909468777819));
#37688=DIRECTION('center_axis',(0.,0.993909468777819,-0.110199672748126));
#37689=DIRECTION('ref_axis',(0.,0.110199672748126,0.993909468777819));
#37690=DIRECTION('',(1.,0.,0.));
#37691=DIRECTION('',(0.,0.110199672748126,0.993909468777819));
#37692=DIRECTION('center_axis',(1.,0.,0.));
#37693=DIRECTION('ref_axis',(0.,0.866025403784439,0.5));
#37694=DIRECTION('center_axis',(1.,0.,0.));
#37695=DIRECTION('ref_axis',(0.,1.,0.));
#37696=DIRECTION('center_axis',(0.,-0.554454844738281,-0.83221380975459));
#37697=DIRECTION('ref_axis',(0.,0.83221380975459,-0.554454844738281));
#37698=DIRECTION('',(-1.,0.,0.));
#37699=DIRECTION('',(0.,0.83221380975459,-0.554454844738281));
#37700=DIRECTION('',(1.,0.,0.));
#37701=DIRECTION('',(0.,0.83221380975459,-0.554454844738281));
#37702=DIRECTION('center_axis',(1.,0.,0.));
#37703=DIRECTION('ref_axis',(0.,0.939692620785908,0.342020143325669));
#37704=DIRECTION('center_axis',(-1.,0.,0.));
#37705=DIRECTION('ref_axis',(0.,1.,0.));
#37706=DIRECTION('',(0.,0.281116060120937,0.959673778292437));
#37707=DIRECTION('center_axis',(0.,0.959673778292437,-0.281116060120937));
#37708=DIRECTION('ref_axis',(0.,0.281116060120937,0.959673778292437));
#37709=DIRECTION('',(1.,0.,0.));
#37710=DIRECTION('',(0.,0.281116060120937,0.959673778292437));
#37711=DIRECTION('center_axis',(1.,0.,0.));
#37712=DIRECTION('ref_axis',(0.,0.939692620785908,0.342020143325669));
#37713=DIRECTION('center_axis',(1.,0.,0.));
#37714=DIRECTION('ref_axis',(0.,1.,0.));
#37715=DIRECTION('center_axis',(0.,-0.690543841286577,-0.723290538622744));
#37716=DIRECTION('ref_axis',(0.,0.723290538622744,-0.690543841286577));
#37717=DIRECTION('',(-1.,0.,0.));
#37718=DIRECTION('',(0.,0.723290538622744,-0.690543841286577));
#37719=DIRECTION('',(1.,0.,0.));
#37720=DIRECTION('',(0.,0.723290538622744,-0.690543841286577));
#37721=DIRECTION('center_axis',(1.,0.,0.));
#37722=DIRECTION('ref_axis',(0.,0.984807753012208,0.17364817766693));
#37723=DIRECTION('center_axis',(-1.,0.,0.));
#37724=DIRECTION('ref_axis',(0.,1.,0.));
#37725=DIRECTION('',(0.,0.443490878258564,0.896278885672003));
#37726=DIRECTION('center_axis',(0.,0.896278885672003,-0.443490878258564));
#37727=DIRECTION('ref_axis',(0.,0.443490878258564,0.896278885672003));
#37728=DIRECTION('',(1.,0.,0.));
#37729=DIRECTION('',(0.,0.443490878258564,0.896278885672003));
#37730=DIRECTION('center_axis',(1.,0.,0.));
#37731=DIRECTION('ref_axis',(0.,0.984807753012208,0.17364817766693));
#37732=DIRECTION('center_axis',(1.,0.,0.));
#37733=DIRECTION('ref_axis',(0.,1.,0.));
#37734=DIRECTION('center_axis',(0.,-0.805651012649425,-0.592390450477518));
#37735=DIRECTION('ref_axis',(0.,0.592390450477518,-0.805651012649425));
#37736=DIRECTION('',(-1.,0.,0.));
#37737=DIRECTION('',(0.,0.592390450477518,-0.805651012649425));
#37738=DIRECTION('',(1.,0.,0.));
#37739=DIRECTION('',(0.,0.592390450477518,-0.805651012649425));
#37740=DIRECTION('center_axis',(1.,0.,0.));
#37741=DIRECTION('ref_axis',(0.,1.,-6.12323399573677E-17));
#37742=DIRECTION('center_axis',(-1.,0.,0.));
#37743=DIRECTION('ref_axis',(0.,1.,0.));
#37744=DIRECTION('',(0.,0.592390450477518,0.805651012649425));
#37745=DIRECTION('center_axis',(0.,0.805651012649425,-0.592390450477518));
#37746=DIRECTION('ref_axis',(0.,0.592390450477518,0.805651012649425));
#37747=DIRECTION('',(1.,0.,0.));
#37748=DIRECTION('',(0.,0.592390450477518,0.805651012649425));
#37749=DIRECTION('center_axis',(1.,0.,0.));
#37750=DIRECTION('ref_axis',(0.,1.,-6.12323399573677E-17));
#37751=DIRECTION('center_axis',(1.,0.,0.));
#37752=DIRECTION('ref_axis',(0.,1.,0.));
#37753=DIRECTION('center_axis',(0.,-0.896278885672003,-0.443490878258564));
#37754=DIRECTION('ref_axis',(0.,0.443490878258564,-0.896278885672003));
#37755=DIRECTION('',(-1.,0.,0.));
#37756=DIRECTION('',(0.,0.443490878258564,-0.896278885672003));
#37757=DIRECTION('',(1.,0.,0.));
#37758=DIRECTION('',(0.,0.443490878258564,-0.896278885672003));
#37759=DIRECTION('center_axis',(1.,0.,0.));
#37760=DIRECTION('ref_axis',(0.,0.984807753012208,-0.17364817766693));
#37761=DIRECTION('center_axis',(-1.,0.,0.));
#37762=DIRECTION('ref_axis',(0.,1.,0.));
#37763=DIRECTION('',(0.,0.723290538622744,0.690543841286577));
#37764=DIRECTION('center_axis',(0.,0.690543841286577,-0.723290538622744));
#37765=DIRECTION('ref_axis',(0.,0.723290538622744,0.690543841286577));
#37766=DIRECTION('',(1.,0.,0.));
#37767=DIRECTION('',(0.,0.723290538622744,0.690543841286577));
#37768=DIRECTION('center_axis',(1.,0.,0.));
#37769=DIRECTION('ref_axis',(0.,0.984807753012208,-0.17364817766693));
#37770=DIRECTION('center_axis',(1.,0.,0.));
#37771=DIRECTION('ref_axis',(0.,1.,0.));
#37772=DIRECTION('center_axis',(0.,-0.959673778292437,-0.281116060120937));
#37773=DIRECTION('ref_axis',(0.,0.281116060120937,-0.959673778292437));
#37774=DIRECTION('',(-1.,0.,0.));
#37775=DIRECTION('',(0.,0.281116060120937,-0.959673778292437));
#37776=DIRECTION('',(1.,0.,0.));
#37777=DIRECTION('',(0.,0.281116060120937,-0.959673778292437));
#37778=DIRECTION('center_axis',(1.,0.,0.));
#37779=DIRECTION('ref_axis',(0.,0.939692620785908,-0.342020143325669));
#37780=DIRECTION('center_axis',(-1.,0.,0.));
#37781=DIRECTION('ref_axis',(0.,1.,0.));
#37782=DIRECTION('',(0.,0.83221380975459,0.554454844738281));
#37783=DIRECTION('center_axis',(0.,0.554454844738281,-0.83221380975459));
#37784=DIRECTION('ref_axis',(0.,0.83221380975459,0.554454844738281));
#37785=DIRECTION('',(1.,0.,0.));
#37786=DIRECTION('',(0.,0.83221380975459,0.554454844738281));
#37787=DIRECTION('center_axis',(1.,0.,0.));
#37788=DIRECTION('ref_axis',(0.,0.939692620785908,-0.342020143325669));
#37789=DIRECTION('center_axis',(1.,0.,0.));
#37790=DIRECTION('ref_axis',(0.,1.,0.));
#37791=DIRECTION('center_axis',(0.,-0.993909468777819,-0.110199672748125));
#37792=DIRECTION('ref_axis',(0.,0.110199672748125,-0.993909468777819));
#37793=DIRECTION('',(-1.,0.,0.));
#37794=DIRECTION('',(0.,0.110199672748125,-0.993909468777819));
#37795=DIRECTION('',(1.,0.,0.));
#37796=DIRECTION('',(0.,0.110199672748125,-0.993909468777819));
#37797=DIRECTION('center_axis',(1.,0.,0.));
#37798=DIRECTION('ref_axis',(0.,0.866025403784439,-0.5));
#37799=DIRECTION('center_axis',(-1.,0.,0.));
#37800=DIRECTION('ref_axis',(0.,1.,0.));
#37801=DIRECTION('',(0.,0.91585068539755,0.401519018300301));
#37802=DIRECTION('center_axis',(0.,0.401519018300301,-0.91585068539755));
#37803=DIRECTION('ref_axis',(0.,0.91585068539755,0.401519018300301));
#37804=DIRECTION('',(1.,0.,0.));
#37805=DIRECTION('',(0.,0.91585068539755,0.401519018300301));
#37806=DIRECTION('center_axis',(1.,0.,0.));
#37807=DIRECTION('ref_axis',(0.,0.866025403784439,-0.5));
#37808=DIRECTION('center_axis',(1.,0.,0.));
#37809=DIRECTION('ref_axis',(0.,1.,0.));
#37810=DIRECTION('center_axis',(0.,-0.997945722996845,0.0640650759174131));
#37811=DIRECTION('ref_axis',(0.,-0.0640650759174131,-0.997945722996845));
#37812=DIRECTION('',(-1.,0.,0.));
#37813=DIRECTION('',(0.,-0.0640650759174131,-0.997945722996845));
#37814=DIRECTION('',(1.,0.,0.));
#37815=DIRECTION('',(0.,-0.0640650759174131,-0.997945722996845));
#37816=DIRECTION('center_axis',(1.,0.,0.));
#37817=DIRECTION('ref_axis',(0.,0.766044443118978,-0.642787609686539));
#37818=DIRECTION('center_axis',(-1.,0.,0.));
#37819=DIRECTION('ref_axis',(0.,1.,0.));
#37820=DIRECTION('',(0.,0.971659901407514,0.236383239669693));
#37821=DIRECTION('center_axis',(0.,0.236383239669693,-0.971659901407514));
#37822=DIRECTION('ref_axis',(0.,0.971659901407514,0.236383239669693));
#37823=DIRECTION('',(1.,0.,0.));
#37824=DIRECTION('',(0.,0.971659901407514,0.236383239669693));
#37825=DIRECTION('center_axis',(1.,0.,0.));
#37826=DIRECTION('ref_axis',(0.,0.766044443118978,-0.642787609686539));
#37827=DIRECTION('center_axis',(1.,0.,0.));
#37828=DIRECTION('ref_axis',(0.,1.,0.));
#37829=DIRECTION('center_axis',(0.,-0.971659901407514,0.236383239669694));
#37830=DIRECTION('ref_axis',(0.,-0.236383239669694,-0.971659901407514));
#37831=DIRECTION('',(-1.,0.,0.));
#37832=DIRECTION('',(0.,-0.236383239669694,-0.971659901407514));
#37833=DIRECTION('',(1.,0.,0.));
#37834=DIRECTION('',(0.,-0.236383239669694,-0.971659901407514));
#37835=DIRECTION('center_axis',(1.,0.,0.));
#37836=DIRECTION('ref_axis',(0.,0.642787609686539,-0.766044443118978));
#37837=DIRECTION('center_axis',(-1.,0.,0.));
#37838=DIRECTION('ref_axis',(0.,1.,0.));
#37839=DIRECTION('',(0.,0.997945722996845,0.064065075917413));
#37840=DIRECTION('center_axis',(0.,0.064065075917413,-0.997945722996845));
#37841=DIRECTION('ref_axis',(0.,0.997945722996845,0.064065075917413));
#37842=DIRECTION('',(1.,0.,0.));
#37843=DIRECTION('',(0.,0.997945722996845,0.064065075917413));
#37844=DIRECTION('center_axis',(1.,0.,0.));
#37845=DIRECTION('ref_axis',(0.,0.642787609686539,-0.766044443118978));
#37846=DIRECTION('center_axis',(1.,0.,0.));
#37847=DIRECTION('ref_axis',(0.,1.,0.));
#37848=DIRECTION('center_axis',(0.,-0.91585068539755,0.401519018300301));
#37849=DIRECTION('ref_axis',(0.,-0.401519018300301,-0.91585068539755));
#37850=DIRECTION('',(-1.,0.,0.));
#37851=DIRECTION('',(0.,-0.401519018300301,-0.91585068539755));
#37852=DIRECTION('',(1.,0.,0.));
#37853=DIRECTION('',(0.,-0.401519018300301,-0.91585068539755));
#37854=DIRECTION('center_axis',(1.,0.,0.));
#37855=DIRECTION('ref_axis',(0.,0.5,-0.866025403784439));
#37856=DIRECTION('center_axis',(-1.,0.,0.));
#37857=DIRECTION('ref_axis',(0.,1.,0.));
#37858=DIRECTION('',(0.,0.993909468777819,-0.110199672748126));
#37859=DIRECTION('center_axis',(0.,-0.110199672748126,-0.993909468777819));
#37860=DIRECTION('ref_axis',(0.,0.993909468777819,-0.110199672748126));
#37861=DIRECTION('',(1.,0.,0.));
#37862=DIRECTION('',(0.,0.993909468777819,-0.110199672748126));
#37863=DIRECTION('center_axis',(1.,0.,0.));
#37864=DIRECTION('ref_axis',(0.,0.5,-0.866025403784439));
#37865=DIRECTION('center_axis',(1.,0.,0.));
#37866=DIRECTION('ref_axis',(0.,1.,0.));
#37867=DIRECTION('center_axis',(0.,-0.83221380975459,0.554454844738281));
#37868=DIRECTION('ref_axis',(0.,-0.554454844738281,-0.83221380975459));
#37869=DIRECTION('',(-1.,0.,0.));
#37870=DIRECTION('',(0.,-0.554454844738281,-0.83221380975459));
#37871=DIRECTION('',(1.,0.,0.));
#37872=DIRECTION('',(0.,-0.554454844738281,-0.83221380975459));
#37873=DIRECTION('center_axis',(1.,0.,0.));
#37874=DIRECTION('ref_axis',(0.,0.342020143325669,-0.939692620785908));
#37875=DIRECTION('center_axis',(-1.,0.,0.));
#37876=DIRECTION('ref_axis',(0.,1.,0.));
#37877=DIRECTION('',(0.,0.959673778292437,-0.281116060120937));
#37878=DIRECTION('center_axis',(0.,-0.281116060120937,-0.959673778292437));
#37879=DIRECTION('ref_axis',(0.,0.959673778292437,-0.281116060120937));
#37880=DIRECTION('',(1.,0.,0.));
#37881=DIRECTION('',(0.,0.959673778292437,-0.281116060120937));
#37882=DIRECTION('center_axis',(1.,0.,0.));
#37883=DIRECTION('ref_axis',(0.,0.342020143325669,-0.939692620785908));
#37884=DIRECTION('center_axis',(1.,0.,0.));
#37885=DIRECTION('ref_axis',(0.,1.,0.));
#37886=DIRECTION('center_axis',(0.,-0.723290538622744,0.690543841286577));
#37887=DIRECTION('ref_axis',(0.,-0.690543841286577,-0.723290538622744));
#37888=DIRECTION('',(-1.,0.,0.));
#37889=DIRECTION('',(0.,-0.690543841286577,-0.723290538622744));
#37890=DIRECTION('',(1.,0.,0.));
#37891=DIRECTION('',(0.,-0.690543841286577,-0.723290538622744));
#37892=DIRECTION('center_axis',(1.,0.,0.));
#37893=DIRECTION('ref_axis',(0.,0.17364817766693,-0.984807753012208));
#37894=DIRECTION('center_axis',(-1.,0.,0.));
#37895=DIRECTION('ref_axis',(0.,1.,0.));
#37896=DIRECTION('',(0.,0.896278885672003,-0.443490878258564));
#37897=DIRECTION('center_axis',(0.,-0.443490878258564,-0.896278885672003));
#37898=DIRECTION('ref_axis',(0.,0.896278885672003,-0.443490878258564));
#37899=DIRECTION('',(1.,0.,0.));
#37900=DIRECTION('',(0.,0.896278885672003,-0.443490878258564));
#37901=DIRECTION('center_axis',(1.,0.,0.));
#37902=DIRECTION('ref_axis',(0.,0.17364817766693,-0.984807753012208));
#37903=DIRECTION('center_axis',(1.,0.,0.));
#37904=DIRECTION('ref_axis',(0.,1.,0.));
#37905=DIRECTION('center_axis',(0.,-0.592390450477518,0.805651012649425));
#37906=DIRECTION('ref_axis',(0.,-0.805651012649425,-0.592390450477518));
#37907=DIRECTION('',(-1.,0.,0.));
#37908=DIRECTION('',(0.,-0.805651012649425,-0.592390450477518));
#37909=DIRECTION('',(1.,0.,0.));
#37910=DIRECTION('',(0.,-0.805651012649425,-0.592390450477518));
#37911=DIRECTION('center_axis',(1.,0.,0.));
#37912=DIRECTION('ref_axis',(0.,0.,-1.));
#37913=DIRECTION('center_axis',(-1.,0.,0.));
#37914=DIRECTION('ref_axis',(0.,1.,0.));
#37915=DIRECTION('',(0.,0.805651012649425,-0.592390450477518));
#37916=DIRECTION('center_axis',(0.,-0.592390450477518,-0.805651012649425));
#37917=DIRECTION('ref_axis',(0.,0.805651012649425,-0.592390450477518));
#37918=DIRECTION('',(1.,0.,0.));
#37919=DIRECTION('',(0.,0.805651012649425,-0.592390450477518));
#37920=DIRECTION('center_axis',(1.,0.,0.));
#37921=DIRECTION('ref_axis',(0.,0.,-1.));
#37922=DIRECTION('center_axis',(1.,0.,0.));
#37923=DIRECTION('ref_axis',(0.,1.,0.));
#37924=DIRECTION('center_axis',(1.,0.,0.));
#37925=DIRECTION('ref_axis',(0.,1.,0.));
#37926=DIRECTION('',(0.519218171713667,-0.854641732050523,-1.04663426157342E-16));
#37927=DIRECTION('center_axis',(-1.,0.,0.));
#37928=DIRECTION('ref_axis',(0.,1.,0.));
#37929=DIRECTION('center_axis',(0.,0.5,0.866025403784439));
#37930=DIRECTION('ref_axis',(0.,0.866025403784439,-0.5));
#37931=DIRECTION('',(0.,0.866025403784439,-0.5));
#37932=DIRECTION('',(-1.,0.,0.));
#37933=DIRECTION('',(0.,0.866025403784439,-0.5));
#37934=DIRECTION('',(-1.,0.,0.));
#37935=DIRECTION('center_axis',(0.,-0.5,0.866025403784439));
#37936=DIRECTION('ref_axis',(0.,0.866025403784439,0.5));
#37937=DIRECTION('',(0.,0.866025403784439,0.5));
#37938=DIRECTION('',(-1.,0.,0.));
#37939=DIRECTION('',(0.,0.866025403784439,0.5));
#37940=DIRECTION('center_axis',(0.,-1.,-1.60246890531964E-16));
#37941=DIRECTION('ref_axis',(0.,-1.60246890531964E-16,1.));
#37942=DIRECTION('',(0.,-1.60246890531964E-16,1.));
#37943=DIRECTION('',(-1.,0.,0.));
#37944=DIRECTION('',(0.,-1.60246890531964E-16,1.));
#37945=DIRECTION('center_axis',(0.,-0.5,-0.866025403784439));
#37946=DIRECTION('ref_axis',(0.,-0.866025403784439,0.5));
#37947=DIRECTION('',(0.,-0.866025403784439,0.5));
#37948=DIRECTION('',(-1.,0.,0.));
#37949=DIRECTION('',(0.,-0.866025403784439,0.5));
#37950=DIRECTION('center_axis',(0.,0.5,-0.866025403784439));
#37951=DIRECTION('ref_axis',(0.,-0.866025403784439,-0.5));
#37952=DIRECTION('',(0.,-0.866025403784439,-0.5));
#37953=DIRECTION('',(-1.,0.,0.));
#37954=DIRECTION('',(0.,-0.866025403784439,-0.5));
#37955=DIRECTION('center_axis',(0.,1.,-3.20493781063927E-16));
#37956=DIRECTION('ref_axis',(0.,-3.20493781063927E-16,-1.));
#37957=DIRECTION('',(0.,-3.20493781063927E-16,-1.));
#37958=DIRECTION('',(0.,-3.20493781063927E-16,-1.));
#37959=DIRECTION('center_axis',(-1.,0.,0.));
#37960=DIRECTION('ref_axis',(0.,0.,1.));
#37961=DIRECTION('center_axis',(-1.,0.,0.));
#37962=DIRECTION('ref_axis',(0.,0.,1.));
#37963=DIRECTION('center_axis',(1.,0.,0.));
#37964=DIRECTION('ref_axis',(0.,0.,-1.));
#37965=DIRECTION('center_axis',(1.,0.,0.));
#37966=DIRECTION('ref_axis',(0.,1.,0.));
#37967=DIRECTION('',(-0.707106781186548,0.707106781186547,8.65956056235493E-17));
#37968=DIRECTION('center_axis',(1.,0.,0.));
#37969=DIRECTION('ref_axis',(0.,1.,0.));
#37970=DIRECTION('center_axis',(1.,0.,0.));
#37971=DIRECTION('ref_axis',(0.,0.,-1.));
#37972=DIRECTION('',(-1.,0.,0.));
#37973=DIRECTION('',(-1.,0.,0.));
#37974=DIRECTION('center_axis',(-1.,0.,0.));
#37975=DIRECTION('ref_axis',(0.,1.,0.));
#37976=DIRECTION('center_axis',(1.,0.,0.));
#37977=DIRECTION('ref_axis',(0.,0.,-1.));
#37978=DIRECTION('',(-0.707106781186548,-0.707106781186547,-8.65956056235493E-17));
#37979=DIRECTION('center_axis',(1.,0.,0.));
#37980=DIRECTION('ref_axis',(0.,0.,-1.));
#49569=CARTESIAN_POINT('',(0.,0.,0.));
#49570=CARTESIAN_POINT('Origin',(-14.8,0.,0.));
#49571=CARTESIAN_POINT('',(-29.4201303078758,-1.95635727925632,0.00126400008466199));
#49572=CARTESIAN_POINT('',(-29.5218696921242,-1.95587002060241,0.00207606461394834));
#49573=CARTESIAN_POINT('',(-14.8,-1.954,-2.39295984553393E-16));
#49574=CARTESIAN_POINT('',(-29.646,0.862546263840124,1.75512488719095));
#49575=CARTESIAN_POINT('Ctrl Pts',(-29.4201303078758,-1.95635727925632,
0.00126400008466199));
#49576=CARTESIAN_POINT('Ctrl Pts',(-29.4239164395046,-1.95681317725995,
0.0674360876992789));
#49577=CARTESIAN_POINT('Ctrl Pts',(-29.4277025711335,-1.95374769504203,
0.133562632555316));
#49578=CARTESIAN_POINT('Ctrl Pts',(-29.4314887027624,-1.94702183852209,
0.199311248981777));
#49579=CARTESIAN_POINT('Ctrl Pts',(-29.4685374843882,-1.88120669687356,
0.84268722503347));
#49580=CARTESIAN_POINT('Ctrl Pts',(-29.505586266014,-1.46489646277197,1.44987508234769));
#49581=CARTESIAN_POINT('Ctrl Pts',(-29.5426350476398,-0.888515909042488,
1.74370487454672));
#49582=CARTESIAN_POINT('Ctrl Pts',(-29.5770900317598,-0.352487949298946,
2.0169635454113));
#49583=CARTESIAN_POINT('Ctrl Pts',(-29.6115450158799,0.321981753721779,
2.01920484775088));
#49584=CARTESIAN_POINT('Ctrl Pts',(-29.646,0.86356666800971,1.75642846275437));
#49585=CARTESIAN_POINT('',(-29.646,-0.86152585967032,1.75382131162765));
#49586=CARTESIAN_POINT('Origin',(-29.646,0.,0.));
#49587=CARTESIAN_POINT('Ctrl Pts',(-29.646,-0.861525859670322,1.75382131162764));
#49588=CARTESIAN_POINT('Ctrl Pts',(-29.6089512183742,-1.44475753426074,
1.46732167423177));
#49589=CARTESIAN_POINT('Ctrl Pts',(-29.5719024367484,-1.86881203157243,
0.869533272325591));
#49590=CARTESIAN_POINT('Ctrl Pts',(-29.5348536551226,-1.94371535502012,
0.228137491017513));
#49591=CARTESIAN_POINT('Ctrl Pts',(-29.5305256674564,-1.95246545814925,
0.153210518825829));
#49592=CARTESIAN_POINT('Ctrl Pts',(-29.5261976797903,-1.9564508380952,0.0776884545733211));
#49593=CARTESIAN_POINT('Ctrl Pts',(-29.5218696921242,-1.95587002060241,
0.00207606461394834));
#49594=CARTESIAN_POINT('Origin',(-14.8,0.,0.));
#49595=CARTESIAN_POINT('',(-28.7201303078758,-1.95131029814799,0.00101044981481321));
#49596=CARTESIAN_POINT('',(-28.8218696921242,-1.95116704690989,0.000889418674697316));
#49597=CARTESIAN_POINT('',(-14.8,-1.954,-2.39295984553393E-16));
#49598=CARTESIAN_POINT('Ctrl Pts',(-28.7201303078758,-1.95131029814799,
0.00101044981481321));
#49599=CARTESIAN_POINT('Ctrl Pts',(-28.7349570830831,-1.95252967038394,
0.261887710632697));
#49600=CARTESIAN_POINT('Ctrl Pts',(-28.7497838582905,-1.90389966119072,
0.522328508406575));
#49601=CARTESIAN_POINT('Ctrl Pts',(-28.7646106334978,-1.80327229746782,
0.760829685636639));
#49602=CARTESIAN_POINT('Ctrl Pts',(-28.8016594151236,-1.55182711319731,
1.35679056783254));
#49603=CARTESIAN_POINT('Ctrl Pts',(-28.8387081967495,-0.975716756591996,
1.81576312150198));
#49604=CARTESIAN_POINT('Ctrl Pts',(-28.8757569783753,-0.338635417708894,
1.92768240089395));
#49605=CARTESIAN_POINT('Ctrl Pts',(-28.9128057600011,0.298445921174204,
2.03960168028592));
#49606=CARTESIAN_POINT('Ctrl Pts',(-28.9498545416268,0.996498242335083,
1.80446768540043));
#49607=CARTESIAN_POINT('Ctrl Pts',(-28.9869033232527,1.43600427644337,1.32987593120208));
#49608=CARTESIAN_POINT('Ctrl Pts',(-29.0239521048785,1.87551031055165,0.855284177003728));
#49609=CARTESIAN_POINT('Ctrl Pts',(-29.0610008865043,2.05647005760734,0.14123466349252));
#49610=CARTESIAN_POINT('Ctrl Pts',(-29.0980496681301,1.89606454202561,-0.485381428782411));
#49611=CARTESIAN_POINT('Ctrl Pts',(-29.1350984497559,1.73565902644388,-1.11199752105734));
#49612=CARTESIAN_POINT('Ctrl Pts',(-29.1721472313817,1.23388824822474,-1.65118019209599));
#49613=CARTESIAN_POINT('Ctrl Pts',(-29.2091960130075,0.62040376768731,-1.85624320320092));
#49614=CARTESIAN_POINT('Ctrl Pts',(-29.2462447946333,0.0069192871498789,
-2.06130621430585));
#49615=CARTESIAN_POINT('Ctrl Pts',(-29.2832935762591,-0.718278895705847,
-1.93224956547705));
#49616=CARTESIAN_POINT('Ctrl Pts',(-29.320342357885,-1.22321796253597,-1.52793919366807));
#49617=CARTESIAN_POINT('Ctrl Pts',(-29.3536050078819,-1.67655571651092,
-1.16494657157745));
#49618=CARTESIAN_POINT('Ctrl Pts',(-29.3868676578788,-1.95235203664581,
-0.580083719870375));
#49619=CARTESIAN_POINT('Ctrl Pts',(-29.4201303078758,-1.95635727925632,
0.00126400008466199));
#49620=CARTESIAN_POINT('Ctrl Pts',(-29.5218696921242,-1.95587002060241,
0.00207606461394834));
#49621=CARTESIAN_POINT('Ctrl Pts',(-29.4891488981645,-1.95147887834975,
-0.569574694009445));
#49622=CARTESIAN_POINT('Ctrl Pts',(-29.4564281042048,-1.68609385625763,
-1.14638827290075));
#49623=CARTESIAN_POINT('Ctrl Pts',(-29.4237073102451,-1.24550369432567,
-1.51024047045956));
#49624=CARTESIAN_POINT('Ctrl Pts',(-29.3866585286193,-0.746636560599803,
-1.92221948991858));
#49625=CARTESIAN_POINT('Ctrl Pts',(-29.3496097469935,-0.0231501435643523,
-2.06117436812664));
#49626=CARTESIAN_POINT('Ctrl Pts',(-29.3125609653677,0.593320342234026,
-1.86492298541111));
#49627=CARTESIAN_POINT('Ctrl Pts',(-29.2755121837419,1.2097908280324,-1.66867160269558));
#49628=CARTESIAN_POINT('Ctrl Pts',(-29.2384634021161,1.71924538259371,-1.13721395905646));
#49629=CARTESIAN_POINT('Ctrl Pts',(-29.2014146204903,1.88874566918039,-0.513087459649483));
#49630=CARTESIAN_POINT('Ctrl Pts',(-29.1643658388645,2.05824595576708,0.111039039757497));
#49631=CARTESIAN_POINT('Ctrl Pts',(-29.1273170572387,1.88779197437914,0.827834394932333));
#49632=CARTESIAN_POINT('Ctrl Pts',(-29.0902682756129,1.45527344708612,1.30883134527791));
#49633=CARTESIAN_POINT('Ctrl Pts',(-29.0532194939871,1.02275491979311,1.78982829562348));
#49634=CARTESIAN_POINT('Ctrl Pts',(-29.0161707123613,0.328171846595005,
2.03502684113979));
#49635=CARTESIAN_POINT('Ctrl Pts',(-28.9791219307355,-0.310483119724783,
1.93239222026172));
#49636=CARTESIAN_POINT('Ctrl Pts',(-28.9420731491096,-0.949138086044573,
1.82975759938366));
#49637=CARTESIAN_POINT('Ctrl Pts',(-28.9050243674839,-1.53186494548605,
1.37928981211122));
#49638=CARTESIAN_POINT('Ctrl Pts',(-28.867975585858,-1.79197429141891,0.78707299175062));
#49639=CARTESIAN_POINT('Ctrl Pts',(-28.8526069546134,-1.89987324100642,
0.541408720765679));
#49640=CARTESIAN_POINT('Ctrl Pts',(-28.8372383233688,-1.9522571758889,0.271352718622898));
#49641=CARTESIAN_POINT('Ctrl Pts',(-28.8218696921242,-1.95116704690989,
0.000889418674697316));
#49642=CARTESIAN_POINT('Origin',(-14.8,0.,0.));
#49643=CARTESIAN_POINT('',(-28.0201303078758,-1.95270169711206,-0.00166393224656974));
#49644=CARTESIAN_POINT('',(-28.1218696921242,-1.95296243627918,-0.001715799027382));
#49645=CARTESIAN_POINT('',(-14.8,-1.954,-2.39295984553393E-16));
#49646=CARTESIAN_POINT('Ctrl Pts',(-28.0201303078758,-1.95270169711206,
-0.00166393224656974));
#49647=CARTESIAN_POINT('Ctrl Pts',(-28.0459977266616,-1.94902264159807,
0.452657212652301));
#49648=CARTESIAN_POINT('Ctrl Pts',(-28.0718651454474,-1.79103646858732,
0.909285351732831));
#49649=CARTESIAN_POINT('Ctrl Pts',(-28.0977325642333,-1.50128604242506,
1.25570336172352));
#49650=CARTESIAN_POINT('Ctrl Pts',(-28.1347813458591,-1.08628907833883,
1.75186284750948));
#49651=CARTESIAN_POINT('Ctrl Pts',(-28.1718301274849,-0.400996326824849,
2.0219417923873));
#49652=CARTESIAN_POINT('Ctrl Pts',(-28.2088789091107,0.240920463268404,
1.94232014777131));
#49653=CARTESIAN_POINT('Ctrl Pts',(-28.2459276907365,0.882837253361657,
1.86269850315532));
#49654=CARTESIAN_POINT('Ctrl Pts',(-28.2829764723623,1.48137808203418,1.43337626904552));
#49655=CARTESIAN_POINT('Ctrl Pts',(-28.3200252539881,1.76257907476627,0.850861942132011));
#49656=CARTESIAN_POINT('Ctrl Pts',(-28.3570740356139,2.04378006749835,0.268347615218507));
#49657=CARTESIAN_POINT('Ctrl Pts',(-28.3941228172398,2.00764122428999,-0.467358804498699));
#49658=CARTESIAN_POINT('Ctrl Pts',(-28.4311715988656,1.67070420294189,-1.01950899589596));
#49659=CARTESIAN_POINT('Ctrl Pts',(-28.4682203804914,1.3337671815938,-1.57165918729322));
#49660=CARTESIAN_POINT('Ctrl Pts',(-28.5052691621172,0.696031982105959,
-1.94025315037054));
#49661=CARTESIAN_POINT('Ctrl Pts',(-28.542317943743,0.0494020009907347,
-1.95658054933522));
#49662=CARTESIAN_POINT('Ctrl Pts',(-28.5793667253688,-0.597227980124488,
-1.9729079482999));
#49663=CARTESIAN_POINT('Ctrl Pts',(-28.6164155069946,-1.2527527428671,-1.63696878315194));
#49664=CARTESIAN_POINT('Ctrl Pts',(-28.6534642886204,-1.61712511827056,
-1.10252459521678));
#49665=CARTESIAN_POINT('Ctrl Pts',(-28.6756862950389,-1.83567711673311,
-0.781962847881812));
#49666=CARTESIAN_POINT('Ctrl Pts',(-28.6979083014573,-1.94948273299814,
-0.389985979499672));
#49667=CARTESIAN_POINT('Ctrl Pts',(-28.7201303078758,-1.95131029814799,
0.00101044981481321));
#49668=CARTESIAN_POINT('Ctrl Pts',(-28.8218696921242,-1.95116704690989,
0.000889418674697316));
#49669=CARTESIAN_POINT('Ctrl Pts',(-28.800189541743,-1.94962922875134,-0.380646511372493));
#49670=CARTESIAN_POINT('Ctrl Pts',(-28.7785093913618,-1.84167774817481,
-0.762992966149612));
#49671=CARTESIAN_POINT('Ctrl Pts',(-28.7568292409806,-1.63304206720153,
-1.07881961262616));
#49672=CARTESIAN_POINT('Ctrl Pts',(-28.7197804593548,-1.27650866462705,
-1.61852954319356));
#49673=CARTESIAN_POINT('Ctrl Pts',(-28.682731677729,-0.625950027053866,
-1.96398355087959));
#49674=CARTESIAN_POINT('Ctrl Pts',(-28.6456828961032,0.0208505694140376,
-1.95708928963784));
#49675=CARTESIAN_POINT('Ctrl Pts',(-28.6086341144774,0.667651165881941,
-1.9501950283961));
#49676=CARTESIAN_POINT('Ctrl Pts',(-28.5715853328516,1.31069372124456,-1.59095249822659));
#49677=CARTESIAN_POINT('Ctrl Pts',(-28.5345365512257,1.65565039527921,-1.04377891490295));
#49678=CARTESIAN_POINT('Ctrl Pts',(-28.4974877695999,2.00060706931387,-0.496605331579296));
#49679=CARTESIAN_POINT('Ctrl Pts',(-28.4604389879741,2.04747786202056,0.238499304898493));
#49680=CARTESIAN_POINT('Ctrl Pts',(-28.4233902063483,1.77480635131727,0.82505539855511));
#49681=CARTESIAN_POINT('Ctrl Pts',(-28.3863414247225,1.50213484061398,1.41161149221173));
#49682=CARTESIAN_POINT('Ctrl Pts',(-28.3492926430967,0.909921026500707,
1.84961904304717));
#49683=CARTESIAN_POINT('Ctrl Pts',(-28.3122438614709,0.269234122665934,
1.93859765049293));
#49684=CARTESIAN_POINT('Ctrl Pts',(-28.2751950798451,-0.371452781168839,
2.02757625793869));
#49685=CARTESIAN_POINT('Ctrl Pts',(-28.2381462982193,-1.06061277472511,
1.76752592199477));
#49686=CARTESIAN_POINT('Ctrl Pts',(-28.2010975165935,-1.48280470005023,
1.2774745440133));
#49687=CARTESIAN_POINT('Ctrl Pts',(-28.1746882417704,-1.78375339781367,
0.928153973926285));
#49688=CARTESIAN_POINT('Ctrl Pts',(-28.1482789669473,-1.94905065505998,
0.461965596840646));
#49689=CARTESIAN_POINT('Ctrl Pts',(-28.1218696921242,-1.95296243627918,
-0.001715799027382));
#49690=CARTESIAN_POINT('Origin',(-14.8,0.,0.));
#49691=CARTESIAN_POINT('',(-27.3201303078758,-1.95720343110015,-4.59226069798868E-5));
#49692=CARTESIAN_POINT('',(-27.4218696921242,-1.95719380567024,0.000130774435998158));
#49693=CARTESIAN_POINT('',(-14.8,-1.954,-2.39295984553393E-16));
#49694=CARTESIAN_POINT('Ctrl Pts',(-27.3201303078758,-1.95720343110015,
-4.59226069798868E-5));
#49695=CARTESIAN_POINT('Ctrl Pts',(-27.3570383702401,-1.95698081009987,
0.644334435783812));
#49696=CARTESIAN_POINT('Ctrl Pts',(-27.3939464326044,-1.6076554733493,1.28892163264944));
#49697=CARTESIAN_POINT('Ctrl Pts',(-27.4308544949687,-1.06757773856952,
1.64040494610073));
#49698=CARTESIAN_POINT('Ctrl Pts',(-27.4679032765946,-0.525440850989191,
1.9932283589537));
#49699=CARTESIAN_POINT('Ctrl Pts',(-27.5049520582203,0.208905769743558,
2.05070859500226));
#49700=CARTESIAN_POINT('Ctrl Pts',(-27.5420008398462,0.799337409788294,
1.78653584048903));
#49701=CARTESIAN_POINT('Ctrl Pts',(-27.579049621472,1.38976904983303,1.5223630859758));
#49702=CARTESIAN_POINT('Ctrl Pts',(-27.6160984030978,1.83628570918976,0.936537340900787));
#49703=CARTESIAN_POINT('Ctrl Pts',(-27.6531471847236,1.93450803573618,0.297202416780847));
#49704=CARTESIAN_POINT('Ctrl Pts',(-27.6901959663494,2.0327303622826,-0.342132507339095));
#49705=CARTESIAN_POINT('Ctrl Pts',(-27.7272447479752,1.78265835601873,-1.03497661050397));
#49706=CARTESIAN_POINT('Ctrl Pts',(-27.764293529601,1.29875483693254,-1.46420166094053));
#49707=CARTESIAN_POINT('Ctrl Pts',(-27.8013423112268,0.814851317846355,
-1.89342671137708));
#49708=CARTESIAN_POINT('Ctrl Pts',(-27.8383910928526,0.0971162859378687,
-2.05903270908532));
#49709=CARTESIAN_POINT('Ctrl Pts',(-27.8754398744784,-0.52592899899265,
-1.88521861971562));
#49710=CARTESIAN_POINT('Ctrl Pts',(-27.9124886561042,-1.14897428392317,
-1.71140453034592));
#49711=CARTESIAN_POINT('Ctrl Pts',(-27.9495374377301,-1.67732982187572,
-1.19817035389827));
#49712=CARTESIAN_POINT('Ctrl Pts',(-27.9865862193559,-1.86915700252275,
-0.580433252327395));
#49713=CARTESIAN_POINT('Ctrl Pts',(-27.9977675821958,-1.92705065557309,
-0.393999519036611));
#49714=CARTESIAN_POINT('Ctrl Pts',(-28.0089489450358,-1.95429199318879,
-0.198047251704987));
#49715=CARTESIAN_POINT('Ctrl Pts',(-28.0201303078758,-1.95270169711206,
-0.00166393224656974));
#49716=CARTESIAN_POINT('Ctrl Pts',(-28.1218696921242,-1.95296243627918,
-0.001715799027382));
#49717=CARTESIAN_POINT('Ctrl Pts',(-28.1112301853215,-1.95453837591293,
-0.188519162567876));
#49718=CARTESIAN_POINT('Ctrl Pts',(-28.1005906785188,-1.92992075791155,
-0.374915632262465));
#49719=CARTESIAN_POINT('Ctrl Pts',(-28.0899511717161,-1.87742689675453,
-0.553099583238752));
#49720=CARTESIAN_POINT('Ctrl Pts',(-28.0529023900903,-1.69463331103975,
-1.17356991249032));
#49721=CARTESIAN_POINT('Ctrl Pts',(-28.0158536084645,-1.17382228251622,
-1.69445815097443));
#49722=CARTESIAN_POINT('Ctrl Pts',(-27.9788048268387,-0.553379347191945,
-1.8773442373971));
#49723=CARTESIAN_POINT('Ctrl Pts',(-27.9417560452129,0.0670635881323265,
-2.06023032381977));
#49724=CARTESIAN_POINT('Ctrl Pts',(-27.904707263587,0.787138430257349,-1.905114258181));
#49725=CARTESIAN_POINT('Ctrl Pts',(-27.8676584819612,1.27725304489518,-1.48299535913524));
#49726=CARTESIAN_POINT('Ctrl Pts',(-27.8306097003354,1.76736765953301,-1.06087646008947));
#49727=CARTESIAN_POINT('Ctrl Pts',(-27.7935609187096,2.02752204668364,-0.371754727636712));
#49728=CARTESIAN_POINT('Ctrl Pts',(-27.7565121370838,1.93863843106925,0.268945265900702));
#49729=CARTESIAN_POINT('Ctrl Pts',(-27.719463355458,1.84975481545485,0.909645259438115));
#49730=CARTESIAN_POINT('Ctrl Pts',(-27.6824145738322,1.41183319707542,1.50192351406018));
#49731=CARTESIAN_POINT('Ctrl Pts',(-27.6453657922064,0.825318839035808,
1.77468285389483));
#49732=CARTESIAN_POINT('Ctrl Pts',(-27.6083170105806,0.238804480996198,
2.04744219372948));
#49733=CARTESIAN_POINT('Ctrl Pts',(-27.5712682289548,-0.496302616703593,
2.00068261877672));
#49734=CARTESIAN_POINT('Ctrl Pts',(-27.534219447329,-1.04352966997717,1.65580684870039));
#49735=CARTESIAN_POINT('Ctrl Pts',(-27.4971706657032,-1.59075672325075,
1.31093107862406));
#49736=CARTESIAN_POINT('Ctrl Pts',(-27.4601218840773,-1.95010373209812,
0.667939113424155));
#49737=CARTESIAN_POINT('Ctrl Pts',(-27.4230731024515,-1.9570905808131,0.021140891794882));
#49738=CARTESIAN_POINT('Ctrl Pts',(-27.4226719656757,-1.95716622923779,
0.0141378395533869));
#49739=CARTESIAN_POINT('Ctrl Pts',(-27.4222708288999,-1.95720057063946,
0.00713434110616324));
#49740=CARTESIAN_POINT('Ctrl Pts',(-27.4218696921242,-1.95719380567024,
0.000130774435998158));
#49741=CARTESIAN_POINT('Origin',(-14.8,0.,0.));
#49742=CARTESIAN_POINT('',(-26.6201303078758,-1.95283586288168,0.00169258002336921));
#49743=CARTESIAN_POINT('',(-26.7218696921242,-1.95258020183271,0.00163427418135859));
#49744=CARTESIAN_POINT('',(-14.8,-1.954,-2.39295984553393E-16));
#49745=CARTESIAN_POINT('Ctrl Pts',(-26.6201303078758,-1.95283586288168,
0.00169258002336925));
#49746=CARTESIAN_POINT('Ctrl Pts',(-26.6310302321928,-1.95442075370972,
0.193099573221502));
#49747=CARTESIAN_POINT('Ctrl Pts',(-26.6419301565098,-1.92855963518578,
0.384087563662016));
#49748=CARTESIAN_POINT('Ctrl Pts',(-26.6528300808268,-1.87350212627677,
0.566251176395773));
#49749=CARTESIAN_POINT('Ctrl Pts',(-26.6898788624526,-1.68636196226216,
1.18542427448898));
#49750=CARTESIAN_POINT('Ctrl Pts',(-26.7269276440784,-1.16191114472938,
1.70264789965425));
#49751=CARTESIAN_POINT('Ctrl Pts',(-26.7639764257042,-0.540201001802173,
1.88117875005868));
#49752=CARTESIAN_POINT('Ctrl Pts',(-26.80102520733,0.0815091411250285,2.0597096004631));
#49753=CARTESIAN_POINT('Ctrl Pts',(-26.8380739889558,0.800478609446652,
1.89954767610668));
#49754=CARTESIAN_POINT('Ctrl Pts',(-26.8751227705816,1.28762110954235,1.47400220150885));
#49755=CARTESIAN_POINT('Ctrl Pts',(-26.9121715522074,1.77476360963806,1.04845672691101));
#49756=CARTESIAN_POINT('Ctrl Pts',(-26.9492203338332,2.03007914150785,0.357527702071744));
#49757=CARTESIAN_POINT('Ctrl Pts',(-26.986269115459,1.93670482594731,-0.282533235389988));
#49758=CARTESIAN_POINT('Ctrl Pts',(-27.0233178970849,1.84333051038677,-0.922594172851714));
#49759=CARTESIAN_POINT('Ctrl Pts',(-27.0603666787107,1.40126634739592,-1.5117870229359));
#49760=CARTESIAN_POINT('Ctrl Pts',(-27.0974154603365,0.81285369280208,-1.78042677090386));
#49761=CARTESIAN_POINT('Ctrl Pts',(-27.1344642419623,0.224441038208241,
-2.04906651887181));
#49762=CARTESIAN_POINT('Ctrl Pts',(-27.1715130235881,-0.510320107988586,
-1.99715316472352));
#49763=CARTESIAN_POINT('Ctrl Pts',(-27.2085618052139,-1.05511529455704,
-1.64844846023135));
#49764=CARTESIAN_POINT('Ctrl Pts',(-27.2456105868397,-1.5999104811255,-1.29974375573918));
#49765=CARTESIAN_POINT('Ctrl Pts',(-27.2826593684655,-1.95473970806558,
-0.654247700903117));
#49766=CARTESIAN_POINT('Ctrl Pts',(-27.3197081500913,-1.95719074432167,
-0.00741637865638378));
#49767=CARTESIAN_POINT('Ctrl Pts',(-27.3198488693528,-1.95720005388589,
-0.00495957381760083));
#49768=CARTESIAN_POINT('Ctrl Pts',(-27.3199895886143,-1.95720427988659,
-0.0025027497156606));
#49769=CARTESIAN_POINT('Ctrl Pts',(-27.3201303078758,-1.95720343110015,
-4.59226069797758E-5));
#49770=CARTESIAN_POINT('Ctrl Pts',(-27.4218696921242,-1.95719380567024,
0.000130774435998158));
#49771=CARTESIAN_POINT('Ctrl Pts',(-27.3852220472741,-1.95657576164103,
-0.6397113928845));
#49772=CARTESIAN_POINT('Ctrl Pts',(-27.3485744024242,-1.61286119405438,
-1.28012298663609));
#49773=CARTESIAN_POINT('Ctrl Pts',(-27.3119267575741,-1.07905472547464,
-1.6328782457365));
#49774=CARTESIAN_POINT('Ctrl Pts',(-27.2748779759483,-0.539405332838623,
-1.98949468357996));
#49775=CARTESIAN_POINT('Ctrl Pts',(-27.2378291943225,0.194520141016002,
-2.05212308120823));
#49776=CARTESIAN_POINT('Ctrl Pts',(-27.2007804126967,0.786789750479916,
-1.79209719757795));
#49777=CARTESIAN_POINT('Ctrl Pts',(-27.1637316310709,1.37905935994383,-1.53207131394768));
#49778=CARTESIAN_POINT('Ctrl Pts',(-27.1266828494451,1.82967310501703,-0.949391149058858));
#49779=CARTESIAN_POINT('Ctrl Pts',(-27.0896340678193,1.93237631892021,-0.310760738106043));
#49780=CARTESIAN_POINT('Ctrl Pts',(-27.0525852861935,2.03507953282338,0.327869672846779));
#49781=CARTESIAN_POINT('Ctrl Pts',(-27.0155365045676,1.78987221555653,1.0224503298636));
#49782=CARTESIAN_POINT('Ctrl Pts',(-26.9784877229418,1.30899052071573,1.45505817391017));
#49783=CARTESIAN_POINT('Ctrl Pts',(-26.941438941316,0.828108825874929,1.88766601795674));
#49784=CARTESIAN_POINT('Ctrl Pts',(-26.9043901596902,0.11155275346018,2.05830104903307));
#49785=CARTESIAN_POINT('Ctrl Pts',(-26.8673413780644,-0.512696061414957,
1.88886029737629));
#49786=CARTESIAN_POINT('Ctrl Pts',(-26.8302925964386,-1.1369448762901,1.71941954571951));
#49787=CARTESIAN_POINT('Ctrl Pts',(-26.7932438148128,-1.66888643362564,
1.20990301132961));
#49788=CARTESIAN_POINT('Ctrl Pts',(-26.756195033187,-1.86504074799682,0.593526311295277));
#49789=CARTESIAN_POINT('Ctrl Pts',(-26.7447532528327,-1.92561911203712,
0.40317060976334));
#49790=CARTESIAN_POINT('Ctrl Pts',(-26.7333114724784,-1.9541714137465,0.202623007266345));
#49791=CARTESIAN_POINT('Ctrl Pts',(-26.7218696921242,-1.95258020183271,
0.00163427418135859));
#49792=CARTESIAN_POINT('Origin',(-14.8,0.,0.));
#49793=CARTESIAN_POINT('',(-25.9201303078758,-1.95123630633075,-0.000939509159223334));
#49794=CARTESIAN_POINT('',(-26.0218696921242,-1.95138426211563,-0.00106972641374984));
#49795=CARTESIAN_POINT('',(-14.8,-1.954,-2.39295984553393E-16));
#49796=CARTESIAN_POINT('Ctrl Pts',(-25.9201303078758,-1.95123630633075,
-0.000939509159223334));
#49797=CARTESIAN_POINT('Ctrl Pts',(-25.9420708757713,-1.94955826401817,
0.385140851071647));
#49798=CARTESIAN_POINT('Ctrl Pts',(-25.9640114436667,-1.83881330297959,
0.77210885471596));
#49799=CARTESIAN_POINT('Ctrl Pts',(-25.9859520115622,-1.6254339170275,1.09023630159484));
#49800=CARTESIAN_POINT('Ctrl Pts',(-26.023000793188,-1.26512208229091,1.62742541924811));
#49801=CARTESIAN_POINT('Ctrl Pts',(-26.0600495748139,-0.612162500266134,
1.96832529110062));
#49802=CARTESIAN_POINT('Ctrl Pts',(-26.0970983564397,0.0345725427856284,
1.9568994228693));
#49803=CARTESIAN_POINT('Ctrl Pts',(-26.1341471380655,0.681307585837391,
1.94547355463798));
#49804=CARTESIAN_POINT('Ctrl Pts',(-26.1711959196913,1.32181808991614,1.58172194632284));
#49805=CARTESIAN_POINT('Ctrl Pts',(-26.2082447013171,1.66292995359561,1.03214077594632));
#49806=CARTESIAN_POINT('Ctrl Pts',(-26.2452934829429,2.00404181727508,0.482559605569794));
#49807=CARTESIAN_POINT('Ctrl Pts',(-26.2823422645687,2.04575504055526,-0.252851126868104));
#49808=CARTESIAN_POINT('Ctrl Pts',(-26.3193910461945,1.76897667074363,-0.837479641723851));
#49809=CARTESIAN_POINT('Ctrl Pts',(-26.3564398278203,1.492198300932,-1.4221081565796));
#49810=CARTESIAN_POINT('Ctrl Pts',(-26.3934886094461,0.896928338028557,
-1.85595445385319));
#49811=CARTESIAN_POINT('Ctrl Pts',(-26.4305373910719,0.255633408841942,
-1.94043865459214));
#49812=CARTESIAN_POINT('Ctrl Pts',(-26.4675861726977,-0.385661520344672,
-2.02492285533109));
#49813=CARTESIAN_POINT('Ctrl Pts',(-26.5046349543235,-1.07298141581446,
-1.7600449595354));
#49814=CARTESIAN_POINT('Ctrl Pts',(-26.5416837359493,-1.49172660830113,
-1.26704472612698));
#49815=CARTESIAN_POINT('Ctrl Pts',(-26.5678325932581,-1.78727501250166,
-0.919087460303604));
#49816=CARTESIAN_POINT('Ctrl Pts',(-26.593981450567,-1.94903371867341,-0.457491723232458));
#49817=CARTESIAN_POINT('Ctrl Pts',(-26.6201303078758,-1.95283586288168,
0.00169258002336921));
#49818=CARTESIAN_POINT('Ctrl Pts',(-26.7218696921242,-1.95258020183271,
0.00163427418135859));
#49819=CARTESIAN_POINT('Ctrl Pts',(-26.6962626908526,-1.9490190282882,-0.448183724793736));
#49820=CARTESIAN_POINT('Ctrl Pts',(-26.6706556895811,-1.79447622573103,
-0.900211241067141));
#49821=CARTESIAN_POINT('Ctrl Pts',(-26.6450486883096,-1.51005466648862,
-1.24514472168841));
#49822=CARTESIAN_POINT('Ctrl Pts',(-26.6079999066838,-1.09854719920242,
-1.74420218895902));
#49823=CARTESIAN_POINT('Ctrl Pts',(-26.5709511250579,-0.415165193223192,
-2.01908025782145));
#49824=CARTESIAN_POINT('Ctrl Pts',(-26.5339023434321,0.227294130752652,
-1.94396189573941));
#49825=CARTESIAN_POINT('Ctrl Pts',(-26.4968535618063,0.86975345472849,-1.86884353365738));
#49826=CARTESIAN_POINT('Ctrl Pts',(-26.4598047801805,1.47129009670094,-1.44372874063089));
#49827=CARTESIAN_POINT('Ctrl Pts',(-26.4227559985547,1.75656904907977,-0.863200816547895));
#49828=CARTESIAN_POINT('Ctrl Pts',(-26.3857072169289,2.0418480014586,-0.282672892464901));
#49829=CARTESIAN_POINT('Ctrl Pts',(-26.3486584353031,2.01086926424381,0.453268162674601));
#49830=CARTESIAN_POINT('Ctrl Pts',(-26.3116096536773,1.67781240732092,1.00776783025682));
#49831=CARTESIAN_POINT('Ctrl Pts',(-26.2745608720515,1.34475555039803,1.56226749783905));
#49832=CARTESIAN_POINT('Ctrl Pts',(-26.2375120904257,0.709620573767041,
1.93532577786399));
#49833=CARTESIAN_POINT('Ctrl Pts',(-26.2004633087999,0.0631210955000985,
1.95618664784198));
#49834=CARTESIAN_POINT('Ctrl Pts',(-26.1634145271741,-0.583378382766842,
1.97704751781996));
#49835=CARTESIAN_POINT('Ctrl Pts',(-26.1263657455483,-1.24124236266973,
1.645710977751));
#49836=CARTESIAN_POINT('Ctrl Pts',(-26.0893169639225,-1.60935371975343,
1.11383619917551));
#49837=CARTESIAN_POINT('Ctrl Pts',(-26.0668345399897,-1.8327358451903,0.791077022589047));
#49838=CARTESIAN_POINT('Ctrl Pts',(-26.0443521160569,-1.94941763628547,
0.394470379537052));
#49839=CARTESIAN_POINT('Ctrl Pts',(-26.0218696921242,-1.95138426211563,
-0.00106972641374984));
#49840=CARTESIAN_POINT('Origin',(-14.8,0.,0.));
#49841=CARTESIAN_POINT('',(-25.2201303078758,-1.95626804686365,-0.00119577595913939));
#49842=CARTESIAN_POINT('',(-25.3218696921242,-1.95648018646661,-0.00106297053860165));
#49843=CARTESIAN_POINT('',(-14.8,-1.954,-2.39295984553393E-16));
#49844=CARTESIAN_POINT('Ctrl Pts',(-25.2201303078758,-1.95626804686365,
-0.00119577595913939));
#49845=CARTESIAN_POINT('Ctrl Pts',(-25.2531115193497,-1.95211771839792,
0.575356106654941));
#49846=CARTESIAN_POINT('Ctrl Pts',(-25.2860927308237,-1.68152135564075,
1.15529448608977));
#49847=CARTESIAN_POINT('Ctrl Pts',(-25.3190739422977,-1.23475142449969,
1.51856495798993));
#49848=CARTESIAN_POINT('Ctrl Pts',(-25.3561227239235,-0.732881393773812,
1.92663754789925));
#49849=CARTESIAN_POINT('Ctrl Pts',(-25.3931715055493,-0.00870320332811321,
2.06130338198116));
#49850=CARTESIAN_POINT('Ctrl Pts',(-25.4302202871751,0.606312719881358,
1.86092329171546));
#49851=CARTESIAN_POINT('Ctrl Pts',(-25.4672690688009,1.22132864309083,1.66054320144975));
#49852=CARTESIAN_POINT('Ctrl Pts',(-25.5043178504267,1.72718229906407,1.12511718683642));
#49853=CARTESIAN_POINT('Ctrl Pts',(-25.5413666320525,1.89233464183849,0.499720136913584));
#49854=CARTESIAN_POINT('Ctrl Pts',(-25.5784154136783,2.05748698461291,-0.125676913009264));
#49855=CARTESIAN_POINT('Ctrl Pts',(-25.6154641953042,1.8819380141885,-0.841044998241625));
#49856=CARTESIAN_POINT('Ctrl Pts',(-25.65251297693,1.44603990485877,-1.31894624814468));
#49857=CARTESIAN_POINT('Ctrl Pts',(-25.6895617585558,1.01014179552905,-1.79684749804773));
#49858=CARTESIAN_POINT('Ctrl Pts',(-25.7266105401816,0.313894547294022,
-2.03728191262149));
#49859=CARTESIAN_POINT('Ctrl Pts',(-25.7636593218074,-0.324015947776813,
-1.93019798920358));
#49860=CARTESIAN_POINT('Ctrl Pts',(-25.8007081034332,-0.961926442847647,
-1.82311406578568));
#49861=CARTESIAN_POINT('Ctrl Pts',(-25.837756885059,-1.54150018475429,-1.36851180437611));
#49862=CARTESIAN_POINT('Ctrl Pts',(-25.8748056666848,-1.7974550119834,-0.774471491944305));
#49863=CARTESIAN_POINT('Ctrl Pts',(-25.8899138804151,-1.90183146015221,
-0.532226332702917));
#49864=CARTESIAN_POINT('Ctrl Pts',(-25.9050220941455,-1.95239180157717,
-0.266793366143644));
#49865=CARTESIAN_POINT('Ctrl Pts',(-25.9201303078758,-1.95123630633075,
-0.000939509159223334));
#49866=CARTESIAN_POINT('Ctrl Pts',(-26.0218696921242,-1.95138426211563,
-0.00106972641374984));
#49867=CARTESIAN_POINT('Ctrl Pts',(-26.0073033344311,-1.95265843857347,
-0.257340077086639));
#49868=CARTESIAN_POINT('Ctrl Pts',(-25.9927369767381,-1.90577815577188,
-0.513162723070535));
#49869=CARTESIAN_POINT('Ctrl Pts',(-25.978170619045,-1.80856360753824,-0.748163184984166));
#49870=CARTESIAN_POINT('Ctrl Pts',(-25.9411218374192,-1.56130340397485,
-1.34587477348635));
#49871=CARTESIAN_POINT('Ctrl Pts',(-25.9040730557934,-0.988424262583569,
-1.80888493340869));
#49872=CARTESIAN_POINT('Ctrl Pts',(-25.8670242741676,-0.352144096159522,
-1.92526491928297));
#49873=CARTESIAN_POINT('Ctrl Pts',(-25.8299754925418,0.284136070264529,
-2.04164490515726));
#49874=CARTESIAN_POINT('Ctrl Pts',(-25.792926710916,0.98381726172135,-1.81139471698347));
#49875=CARTESIAN_POINT('Ctrl Pts',(-25.7558779292902,1.42664180361434,-1.33990433914493));
#49876=CARTESIAN_POINT('Ctrl Pts',(-25.7188291476644,1.86946634550733,-0.86841396130639));
#49877=CARTESIAN_POINT('Ctrl Pts',(-25.6817803660386,2.0554342378365,-0.155683393803116));
#49878=CARTESIAN_POINT('Ctrl Pts',(-25.6447315844128,1.89942436333606,0.472056735832567));
#49879=CARTESIAN_POINT('Ctrl Pts',(-25.6076828027869,1.74341448883562,1.09979686546825));
#49880=CARTESIAN_POINT('Ctrl Pts',(-25.5706340211611,1.24542684750557,1.64254655723634));
#49881=CARTESIAN_POINT('Ctrl Pts',(-25.5335852395353,0.63340005758682,1.85187873278168));
#49882=CARTESIAN_POINT('Ctrl Pts',(-25.4965364579095,0.021373267668069,
2.06121090832702));
#49883=CARTESIAN_POINT('Ctrl Pts',(-25.4594876762837,-0.704692670839375,
1.93712556764961));
#49884=CARTESIAN_POINT('Ctrl Pts',(-25.4224388946579,-1.21246327201675,
1.53641898188292));
#49885=CARTESIAN_POINT('Ctrl Pts',(-25.3889158271467,-1.67191233880164,
1.17384527939171));
#49886=CARTESIAN_POINT('Ctrl Pts',(-25.3553927596354,-1.95263690100395,
0.584794018605935));
#49887=CARTESIAN_POINT('Ctrl Pts',(-25.3218696921242,-1.95648018646661,
-0.00106297053860165));
#49888=CARTESIAN_POINT('Origin',(-14.8,0.,0.));
#49889=CARTESIAN_POINT('',(-24.5201303078758,-1.95487751651067,0.00168938103890723));
#49890=CARTESIAN_POINT('',(-24.6218696921242,-1.95459134654687,0.00173615845593911));
#49891=CARTESIAN_POINT('',(-14.8,-1.954,-2.39295984553393E-16));
#49892=CARTESIAN_POINT('Ctrl Pts',(-24.5201303078758,-1.95487751651067,
0.00168938103890723));
#49893=CARTESIAN_POINT('Ctrl Pts',(-24.5271033813024,-1.95599066552706,
0.123812897405317));
#49894=CARTESIAN_POINT('Ctrl Pts',(-24.5340764547291,-1.94552840215917,
0.245746288538353));
#49895=CARTESIAN_POINT('Ctrl Pts',(-24.5410495281557,-1.92280272977114,
0.365349523502659));
#49896=CARTESIAN_POINT('Ctrl Pts',(-24.5780983097815,-1.80205848658205,
1.00081596172956));
#49897=CARTESIAN_POINT('Ctrl Pts',(-24.6151470914073,-1.33512736895152,
1.57050383221171));
#49898=CARTESIAN_POINT('Ctrl Pts',(-24.6521958730332,-0.735732820863401,
1.81365592884741));
#49899=CARTESIAN_POINT('Ctrl Pts',(-24.6892446546589,-0.136338272775288,
2.05680802548311));
#49900=CARTESIAN_POINT('Ctrl Pts',(-24.7262934362848,0.595519705770406,
1.97342434827236));
#49901=CARTESIAN_POINT('Ctrl Pts',(-24.7633422179106,1.12485549960288,1.60167122623594));
#49902=CARTESIAN_POINT('Ctrl Pts',(-24.8003909995364,1.65419129343536,1.22991810419951));
#49903=CARTESIAN_POINT('Ctrl Pts',(-24.8374397811622,1.98100490255462,0.569795537337402));
#49904=CARTESIAN_POINT('Ctrl Pts',(-24.874488562788,1.95570738879735,-0.0765455507683978));
#49905=CARTESIAN_POINT('Ctrl Pts',(-24.9115373444138,1.93040987504007,-0.722886638874206));
#49906=CARTESIAN_POINT('Ctrl Pts',(-24.9485861260396,1.55300123840625,-1.35544624822371));
#49907=CARTESIAN_POINT('Ctrl Pts',(-24.9856349076654,0.996228744102698,
-1.68468955637605));
#49908=CARTESIAN_POINT('Ctrl Pts',(-25.0226836892912,0.439456249799152,
-2.01393286452839));
#49909=CARTESIAN_POINT('Ctrl Pts',(-25.059732470917,-0.296680102174122,
-2.03985987148359));
#49910=CARTESIAN_POINT('Ctrl Pts',(-25.0967812525429,-0.875236402009141,
-1.75060328245353));
#49911=CARTESIAN_POINT('Ctrl Pts',(-25.1338300341687,-1.45379270184416,
-1.46134669342348));
#49912=CARTESIAN_POINT('Ctrl Pts',(-25.1708788157945,-1.87476894954092,
-0.856906508408172));
#49913=CARTESIAN_POINT('Ctrl Pts',(-25.2079275974203,-1.94547613788628,
-0.213946743032157));
#49914=CARTESIAN_POINT('Ctrl Pts',(-25.2119951675721,-1.95323905035499,
-0.143356460823001));
#49915=CARTESIAN_POINT('Ctrl Pts',(-25.2160627377239,-1.95677990653869,
-0.0723018731548959));
#49916=CARTESIAN_POINT('Ctrl Pts',(-25.2201303078758,-1.95626804686365,
-0.00119577595913939));
#49917=CARTESIAN_POINT('Ctrl Pts',(-25.3218696921242,-1.95648018646661,
-0.00106297053860165));
#49918=CARTESIAN_POINT('Ctrl Pts',(-25.3183439780096,-1.95688439547276,
-0.0626791772013422));
#49919=CARTESIAN_POINT('Ctrl Pts',(-25.314818263895,-1.95422593398816,-0.124260051025364));
#49920=CARTESIAN_POINT('Ctrl Pts',(-25.3112925497805,-1.94839061142824,
-0.185538403512732));
#49921=CARTESIAN_POINT('Ctrl Pts',(-25.2742437681547,-1.88707208581506,
-0.829461372285711));
#49922=CARTESIAN_POINT('Ctrl Pts',(-25.2371949865289,-1.4749597707414,-1.43997947897568));
#49923=CARTESIAN_POINT('Ctrl Pts',(-25.2001462049031,-0.900685479252096,
-1.7376467251269));
#49924=CARTESIAN_POINT('Ctrl Pts',(-25.1630974232773,-0.326411187762791,
-2.03531397127813));
#49925=CARTESIAN_POINT('Ctrl Pts',(-25.1260486416514,0.41002508014217,-2.02013035689061));
#49926=CARTESIAN_POINT('Ctrl Pts',(-25.0889998600256,0.971542137306138,
-1.69904571725378));
#49927=CARTESIAN_POINT('Ctrl Pts',(-25.0519510783998,1.53305919447011,-1.37796107761694));
#49928=CARTESIAN_POINT('Ctrl Pts',(-25.014902296774,1.91965704089309,-0.750975412730779));
#49929=CARTESIAN_POINT('Ctrl Pts',(-24.9778535151482,1.95438233152165,-0.105072242365784));
#49930=CARTESIAN_POINT('Ctrl Pts',(-24.9408047335224,1.98910762215022,0.540830927999212));
#49931=CARTESIAN_POINT('Ctrl Pts',(-24.9037559518966,1.67196035698436,1.20565160384305));
#49932=CARTESIAN_POINT('Ctrl Pts',(-24.8667071702708,1.14810500076414,1.58508844582887));
#49933=CARTESIAN_POINT('Ctrl Pts',(-24.829658388645,0.624249644543904,1.9645252878147));
#49934=CARTESIAN_POINT('Ctrl Pts',(-24.7926096070192,-0.106313802730695,
2.0585782959425));
#49935=CARTESIAN_POINT('Ctrl Pts',(-24.7555608253934,-0.709192258001544,
1.82419758114917));
#49936=CARTESIAN_POINT('Ctrl Pts',(-24.7185120437676,-1.31207071327239,
1.58981686635583));
#49937=CARTESIAN_POINT('Ctrl Pts',(-24.6814632621418,-1.78726417653948,
1.02700242864135));
#49938=CARTESIAN_POINT('Ctrl Pts',(-24.6444144805159,-1.91726736770191,
0.393365370393976));
#49939=CARTESIAN_POINT('Ctrl Pts',(-24.636899551052,-1.9436370556862,0.264839205983174));
#49940=CARTESIAN_POINT('Ctrl Pts',(-24.6293846215881,-1.95580438407669,
0.133399146235603));
#49941=CARTESIAN_POINT('Ctrl Pts',(-24.6218696921242,-1.95459134654687,
0.00173615845593911));
#49942=CARTESIAN_POINT('Origin',(-14.8,0.,0.));
#49943=CARTESIAN_POINT('',(-23.8201303078758,-1.95080280993935,0.000147472618682448));
#49944=CARTESIAN_POINT('',(-23.9218696921242,-1.95079258945597,-9.01504953382289E-6));
#49945=CARTESIAN_POINT('',(-14.8,-1.954,-2.39295984553393E-16));
#49946=CARTESIAN_POINT('Ctrl Pts',(-23.8201303078758,-1.95080280993935,
0.000147472618682448));
#49947=CARTESIAN_POINT('Ctrl Pts',(-23.8381440248809,-1.95101633693393,
0.317304418787394));
#49948=CARTESIAN_POINT('Ctrl Pts',(-23.856157741886,-1.87806774605225,0.634368765803142));
#49949=CARTESIAN_POINT('Ctrl Pts',(-23.8741714588912,-1.73142413449119,
0.912590312484417));
#49950=CARTESIAN_POINT('Ctrl Pts',(-23.911220240517,-1.42982246394235,1.48480810205256));
#49951=CARTESIAN_POINT('Ctrl Pts',(-23.9482690221428,-0.816490265778046,
1.89272053515694));
#49952=CARTESIAN_POINT('Ctrl Pts',(-23.9853178037686,-0.172161602793372,
1.94961816632452));
#49953=CARTESIAN_POINT('Ctrl Pts',(-24.0223665853944,0.472167060191294,
2.00651579749211));
#49954=CARTESIAN_POINT('Ctrl Pts',(-24.0594153670202,1.14749218799633,1.7123986267229));
#49955=CARTESIAN_POINT('Ctrl Pts',(-24.096464148646,1.54470434954386,1.20188979712753));
#49956=CARTESIAN_POINT('Ctrl Pts',(-24.1335129302718,1.94191651109139,0.691380967532166));
#49957=CARTESIAN_POINT('Ctrl Pts',(-24.1705617118977,2.06101570638141,-0.0355195208893543));
#49958=CARTESIAN_POINT('Ctrl Pts',(-24.2076104935235,1.84748791989433,-0.646095192509194));
#49959=CARTESIAN_POINT('Ctrl Pts',(-24.2446592751493,1.63396013340725,-1.25667086412904));
#49960=CARTESIAN_POINT('Ctrl Pts',(-24.2817080567751,1.08780536514307,-1.75092171894721));
#49961=CARTESIAN_POINT('Ctrl Pts',(-24.3187568384009,0.459009263121902,
-1.90261953850665));
#49962=CARTESIAN_POINT('Ctrl Pts',(-24.3558056200267,-0.169786838899253,
-2.0543173580661));
#49963=CARTESIAN_POINT('Ctrl Pts',(-24.3928544016525,-0.881224274677385,
-1.86346214236683));
#49964=CARTESIAN_POINT('Ctrl Pts',(-24.4299031832783,-1.34966430819263,
-1.41741203153137));
#49965=CARTESIAN_POINT('Ctrl Pts',(-24.4599788914775,-1.72993769745277,
-1.05531448373128));
#49966=CARTESIAN_POINT('Ctrl Pts',(-24.4900545996766,-1.95007637030861,
-0.525044100419769));
#49967=CARTESIAN_POINT('Ctrl Pts',(-24.5201303078758,-1.95487751651067,
0.00168938103890723));
#49968=CARTESIAN_POINT('Ctrl Pts',(-24.6218696921242,-1.95459134654687,
0.00173615845593911));
#49969=CARTESIAN_POINT('Ctrl Pts',(-24.5923358399623,-1.94982408010155,
-0.515702526090927));
#49970=CARTESIAN_POINT('Ctrl Pts',(-24.5628019878004,-1.73839588982394,
-1.03658435362317));
#49971=CARTESIAN_POINT('Ctrl Pts',(-24.5332681356385,-1.37020143243401,
-1.39756878486734));
#49972=CARTESIAN_POINT('Ctrl Pts',(-24.4962193540127,-0.908319386945933,
-1.85040620310102));
#49973=CARTESIAN_POINT('Ctrl Pts',(-24.4591705723869,-0.199742376912028,
-2.05162136078813));
#49974=CARTESIAN_POINT('Ctrl Pts',(-24.4221217907611,0.431200134082752,
-1.90911417108742));
#49975=CARTESIAN_POINT('Ctrl Pts',(-24.3850730091353,1.06214264507754,-1.76660698138671));
#49976=CARTESIAN_POINT('Ctrl Pts',(-24.3480242275095,1.61545065703321,-1.2803774442982));
#49977=CARTESIAN_POINT('Ctrl Pts',(-24.3109754458837,1.83786434332024,-0.672982265317476));
#49978=CARTESIAN_POINT('Ctrl Pts',(-24.2739266642579,2.06027802960727,-0.0655870863367735));
#49979=CARTESIAN_POINT('Ctrl Pts',(-24.236877882632,1.95179739022569,0.662973734536121));
#49980=CARTESIAN_POINT('Ctrl Pts',(-24.1998291010062,1.5620761213606,1.17922375525377));
#49981=CARTESIAN_POINT('Ctrl Pts',(-24.1627803193804,1.17235485249551,1.69547377597143));
#49982=CARTESIAN_POINT('Ctrl Pts',(-24.1257315377547,0.501392954146918,
1.99941299653384));
#49983=CARTESIAN_POINT('Ctrl Pts',(-24.0886827561289,-0.143697277497468,
1.95192253081919));
#49984=CARTESIAN_POINT('Ctrl Pts',(-24.051633974503,-0.788787509141855,
1.90443206510455));
#49985=CARTESIAN_POINT('Ctrl Pts',(-24.0145851928772,-1.40800607408203,
1.50551191311285));
#49986=CARTESIAN_POINT('Ctrl Pts',(-23.9775364112514,-1.71792460509043,
0.937755578551621));
#49987=CARTESIAN_POINT('Ctrl Pts',(-23.958980838209,-1.87314471455058,0.65339955727551));
#49988=CARTESIAN_POINT('Ctrl Pts',(-23.9404252651666,-1.9507792730299,0.326692269225707));
#49989=CARTESIAN_POINT('Ctrl Pts',(-23.9218696921242,-1.95079271425855,
-9.01469875197685E-6));
#49990=CARTESIAN_POINT('Origin',(-14.8,0.,0.));
#49991=CARTESIAN_POINT('',(-23.1201303078758,-1.95433609681919,-0.00176506906220647));
#49992=CARTESIAN_POINT('',(-23.2218696921242,-1.9546244457153,-0.00173153506837734));
#49993=CARTESIAN_POINT('',(-14.8,-1.954,-2.39295984553393E-16));
#49994=CARTESIAN_POINT('Ctrl Pts',(-23.1201303078758,-1.95433609681919,
-0.00176506906220647));
#49995=CARTESIAN_POINT('Ctrl Pts',(-23.1491846684594,-1.94963188416492,
0.507443655012792));
#49996=CARTESIAN_POINT('Ctrl Pts',(-23.178239029043,-1.74573314374161,1.01999030244573));
#49997=CARTESIAN_POINT('Ctrl Pts',(-23.2072933896267,-1.38813175827656,
1.37976115092541));
#49998=CARTESIAN_POINT('Ctrl Pts',(-23.2443421712525,-0.932134951840372,
1.83852435661664));
#49999=CARTESIAN_POINT('Ctrl Pts',(-23.2813909528783,-0.226214953976298,
2.04887143884446));
#50000=CARTESIAN_POINT('Ctrl Pts',(-23.3184397345041,0.406514937820749,
1.91452245149217));
#50001=CARTESIAN_POINT('Ctrl Pts',(-23.3554885161299,1.03924482961779,1.78017346413987));
#50002=CARTESIAN_POINT('Ctrl Pts',(-23.3925372977557,1.59878461534781,1.30112840720746));
#50003=CARTESIAN_POINT('Ctrl Pts',(-23.4295860793815,1.82902206445513,0.696655510044444));
#50004=CARTESIAN_POINT('Ctrl Pts',(-23.4666348610073,2.05925951356244,0.0921826128814311));
#50005=CARTESIAN_POINT('Ctrl Pts',(-23.5036836426331,1.96019462604705,-0.637718124512181));
#50006=CARTESIAN_POINT('Ctrl Pts',(-23.5407324242589,1.57717132553757,-1.15895695426579));
#50007=CARTESIAN_POINT('Ctrl Pts',(-23.5777812058847,1.19414802502809,-1.68019578401941));
#50008=CARTESIAN_POINT('Ctrl Pts',(-23.6148299875105,0.527166311524505,
-1.99277270613302));
#50009=CARTESIAN_POINT('Ctrl Pts',(-23.6518787691363,-0.118483326715247,
-1.9536151906733));
#50010=CARTESIAN_POINT('Ctrl Pts',(-23.6889275507622,-0.76413296495499,
-1.91445767521357));
#50011=CARTESIAN_POINT('Ctrl Pts',(-23.725976332388,-1.3884505279309,-1.52356572218053));
#50012=CARTESIAN_POINT('Ctrl Pts',(-23.7630251140138,-1.70567373795216,
-0.95985817264806));
#50013=CARTESIAN_POINT('Ctrl Pts',(-23.7820601786344,-1.86865789119414,
-0.670234353412065));
#50014=CARTESIAN_POINT('Ctrl Pts',(-23.8010952432551,-1.95057717632143,
-0.334991741763903));
#50015=CARTESIAN_POINT('Ctrl Pts',(-23.8201303078758,-1.95080280993935,
0.000147472618682448));
#50016=CARTESIAN_POINT('Ctrl Pts',(-23.9218696921242,-1.95079271425855,
-9.01469875197685E-6));
#50017=CARTESIAN_POINT('Ctrl Pts',(-23.9033764835408,-1.95080611031183,
-0.325612270080274));
#50018=CARTESIAN_POINT('Ctrl Pts',(-23.8848832749574,-1.87371927457768,
-0.65120956162783));
#50019=CARTESIAN_POINT('Ctrl Pts',(-23.866390066374,-1.71949699819231,-0.934869267377753));
#50020=CARTESIAN_POINT('Ctrl Pts',(-23.8293412847482,-1.41053236320917,
-1.50314526161517));
#50021=CARTESIAN_POINT('Ctrl Pts',(-23.7922925031224,-0.791984596166251,
-1.90310473295927));
#50022=CARTESIAN_POINT('Ctrl Pts',(-23.7552437214965,-0.146975027061406,
-1.95167846104324));
#50023=CARTESIAN_POINT('Ctrl Pts',(-23.7181949398707,0.498034542043438,
-2.0002521891272));
#50024=CARTESIAN_POINT('Ctrl Pts',(-23.681146158245,1.16950591321021,-1.69744017395104));
#50025=CARTESIAN_POINT('Ctrl Pts',(-23.6440973766192,1.56009359464437,-1.18184535783215));
#50026=CARTESIAN_POINT('Ctrl Pts',(-23.6070485949934,1.95068127607854,-0.666250541713246));
#50027=CARTESIAN_POINT('Ctrl Pts',(-23.5699998133675,2.06038526778009,0.0621270753483966));
#50028=CARTESIAN_POINT('Ctrl Pts',(-23.5329510317417,1.83899192144002,0.66989490724899));
#50029=CARTESIAN_POINT('Ctrl Pts',(-23.4959022501159,1.61759857509995,1.27766273914958));
#50030=CARTESIAN_POINT('Ctrl Pts',(-23.4588534684901,1.06510789071826,1.76482078588912));
#50031=CARTESIAN_POINT('Ctrl Pts',(-23.4218046868643,0.434405588214972,
1.90838734506583));
#50032=CARTESIAN_POINT('Ctrl Pts',(-23.3847559052385,-0.196296714288328,
2.05195390424254));
#50033=CARTESIAN_POINT('Ctrl Pts',(-23.3477071236127,-0.905210634913233,
1.85192897585641));
#50034=CARTESIAN_POINT('Ctrl Pts',(-23.3106583419869,-1.36785249955185,
1.39986785567408));
#50035=CARTESIAN_POINT('Ctrl Pts',(-23.281062125366,-1.73743142341591,1.03874130166394));
#50036=CARTESIAN_POINT('Ctrl Pts',(-23.2514659087451,-1.94985119779761,
0.516777199996065));
#50037=CARTESIAN_POINT('Ctrl Pts',(-23.2218696921242,-1.9546244457153,-0.00173153506837734));
#50038=CARTESIAN_POINT('Origin',(-14.8,0.,0.));
#50039=CARTESIAN_POINT('',(-22.4201303078758,-1.95665010086297,0.000936523909256006));
#50040=CARTESIAN_POINT('',(-22.5218696921242,-1.95645680992384,0.00107881945475618));
#50041=CARTESIAN_POINT('',(-14.8,-1.954,-2.39295984553393E-16));
#50042=CARTESIAN_POINT('Ctrl Pts',(-22.4201303078758,-1.95665010086297,
0.000936523909256006));
#50043=CARTESIAN_POINT('Ctrl Pts',(-22.4231765304121,-1.95696499256108,
0.0541608219567786));
#50044=CARTESIAN_POINT('Ctrl Pts',(-22.4262227529484,-1.95498151245914,
0.107361291519809));
#50045=CARTESIAN_POINT('Ctrl Pts',(-22.4292689754847,-1.95062379148406,
0.160366567698355));
#50046=CARTESIAN_POINT('Ctrl Pts',(-22.4663177571105,-1.89762429756401,
0.805027579409392));
#50047=CARTESIAN_POINT('Ctrl Pts',(-22.5033665387363,-1.49342894609215,
1.42081573797912));
#50048=CARTESIAN_POINT('Ctrl Pts',(-22.5404153203621,-0.923045802063583,
1.72587283982099));
#50049=CARTESIAN_POINT('Ctrl Pts',(-22.5774641019879,-0.352662658034998,
2.03092994166288));
#50050=CARTESIAN_POINT('Ctrl Pts',(-22.6145128836137,0.383908278550297,
2.02525598677689));
#50051=CARTESIAN_POINT('Ctrl Pts',(-22.6515616652395,0.949524180064376,
1.71144805454681));
#50052=CARTESIAN_POINT('Ctrl Pts',(-22.6886104468653,1.51514008157843,1.39764012231674));
#50053=CARTESIAN_POINT('Ctrl Pts',(-22.7256592284911,1.90980094802129,0.775698212742586));
#50054=CARTESIAN_POINT('Ctrl Pts',(-22.762708010117,1.95286283342966,0.130297220799477));
#50055=CARTESIAN_POINT('Ctrl Pts',(-22.7997567917428,1.99592471883803,-0.515103771143664));
#50056=CARTESIAN_POINT('Ctrl Pts',(-22.8368055733686,1.68738762321189,-1.18396384545577));
#50057=CARTESIAN_POINT('Ctrl Pts',(-22.8738543549944,1.16847496941632,-1.57013275164443));
#50058=CARTESIAN_POINT('Ctrl Pts',(-22.9109031366202,0.64956231562076,-1.95630165783308));
#50059=CARTESIAN_POINT('Ctrl Pts',(-22.947951918246,-0.0797258963442268,
-2.0597793958983));
#50060=CARTESIAN_POINT('Ctrl Pts',(-22.9850006998718,-0.685580283396735,
-1.83320219478284));
#50061=CARTESIAN_POINT('Ctrl Pts',(-23.0220494814976,-1.29143467044925,
-1.60662499366738));
#50062=CARTESIAN_POINT('Ctrl Pts',(-23.0590982631234,-1.77385523258929,
-1.04999285337124));
#50063=CARTESIAN_POINT('Ctrl Pts',(-23.0961470447492,-1.91202870615516,
-0.418087118645856));
#50064=CARTESIAN_POINT('Ctrl Pts',(-23.1041414657914,-1.94184390860102,
-0.281733903218062));
#50065=CARTESIAN_POINT('Ctrl Pts',(-23.1121358868336,-1.95563047934473,
-0.141875842689035));
#50066=CARTESIAN_POINT('Ctrl Pts',(-23.1201303078758,-1.95433609681919,
-0.00176506906220647));
#50067=CARTESIAN_POINT('Ctrl Pts',(-23.2218696921242,-1.9546244457153,-0.00173153506837734));
#50068=CARTESIAN_POINT('Ctrl Pts',(-23.2144171271193,-1.9558263878705,-0.13229619822038));
#50069=CARTESIAN_POINT('Ctrl Pts',(-23.2069645621144,-1.94386202774871,
-0.262641765960804));
#50070=CARTESIAN_POINT('Ctrl Pts',(-23.1995119971095,-1.91792526049931,
-0.390145061507168));
#50071=CARTESIAN_POINT('Ctrl Pts',(-23.1624632154836,-1.78898634815583,
-1.02399954652756));
#50072=CARTESIAN_POINT('Ctrl Pts',(-23.1254144338578,-1.31473871481652,
-1.58761120458983));
#50073=CARTESIAN_POINT('Ctrl Pts',(-23.088365652232,-0.71225471584897,-1.82300403006431));
#50074=CARTESIAN_POINT('Ctrl Pts',(-23.0513168706062,-0.109770716881404,
-2.05839685553878));
#50075=CARTESIAN_POINT('Ctrl Pts',(-23.0142680889804,0.620949647714409,
-1.96557084842545));
#50076=CARTESIAN_POINT('Ctrl Pts',(-22.9772193073546,1.14544147077387,-1.58701427558519));
#50077=CARTESIAN_POINT('Ctrl Pts',(-22.9401705257288,1.66993329383333,-1.20845770274493));
#50078=CARTESIAN_POINT('Ctrl Pts',(-22.903121744103,1.98819657535644,-0.544170564177744));
#50079=CARTESIAN_POINT('Ctrl Pts',(-22.8660729624772,1.95455602823469,0.101790011156494));
#50080=CARTESIAN_POINT('Ctrl Pts',(-22.8290241808514,1.92091548111294,0.747750586490741));
#50081=CARTESIAN_POINT('Ctrl Pts',(-22.7919753992255,1.53537110534632,1.37538459859205));
#50082=CARTESIAN_POINT('Ctrl Pts',(-22.7549266175997,0.974394052002249,
1.69741176657358));
#50083=CARTESIAN_POINT('Ctrl Pts',(-22.7178778359739,0.413416998658181,
2.0194389345551));
#50084=CARTESIAN_POINT('Ctrl Pts',(-22.6808290543481,-0.322992732263332,
2.03585925841686));
#50085=CARTESIAN_POINT('Ctrl Pts',(-22.6437802727223,-0.897766100098563,
1.73915683691656));
#50086=CARTESIAN_POINT('Ctrl Pts',(-22.6067314910965,-1.4725394679338,1.44245441541625));
#50087=CARTESIAN_POINT('Ctrl Pts',(-22.5696827094707,-1.88567647268274,
0.832629248553874));
#50088=CARTESIAN_POINT('Ctrl Pts',(-22.5326339278449,-1.94807628092868,
0.188810162763719));
#50089=CARTESIAN_POINT('Ctrl Pts',(-22.5290458492713,-1.95411954079142,
0.126457951284427));
#50090=CARTESIAN_POINT('Ctrl Pts',(-22.5254577706977,-1.9568730888356,0.0637868965288276));
#50091=CARTESIAN_POINT('Ctrl Pts',(-22.5218696921242,-1.95645680992384,
0.00107881945475618));
#50092=CARTESIAN_POINT('Origin',(-14.8,0.,0.));
#50093=CARTESIAN_POINT('',(-21.7201303078758,-1.95153139402954,0.00117824056209609));
#50094=CARTESIAN_POINT('',(-21.8218696921242,-1.95136622811345,0.00105513229623864));
#50095=CARTESIAN_POINT('',(-14.8,-1.954,-2.39295984553393E-16));
#50096=CARTESIAN_POINT('Ctrl Pts',(-21.7201303078758,-1.95153139402954,
0.00117824056209609));
#50097=CARTESIAN_POINT('Ctrl Pts',(-21.7342171739906,-1.95289481947734,
0.248965950362388));
#50098=CARTESIAN_POINT('Ctrl Pts',(-21.7483040401054,-1.90914502437453,
0.496290125695869));
#50099=CARTESIAN_POINT('Ctrl Pts',(-21.7623909062202,-1.8180726917492,0.724749818526905));
#50100=CARTESIAN_POINT('Ctrl Pts',(-21.799439687846,-1.57855036392325,1.32560406112565));
#50101=CARTESIAN_POINT('Ctrl Pts',(-21.8364884694718,-1.01169705569096,
1.79597228425755));
#50102=CARTESIAN_POINT('Ctrl Pts',(-21.8735372510976,-0.376972538942942,
1.92055781397538));
#50103=CARTESIAN_POINT('Ctrl Pts',(-21.9105860327234,0.257751977805092,
2.04514334369321));
#50104=CARTESIAN_POINT('Ctrl Pts',(-21.9476348143492,0.960347703068863,
1.82394617999694));
#50105=CARTESIAN_POINT('Ctrl Pts',(-21.984683595975,1.4092229235059,1.35821256208462));
#50106=CARTESIAN_POINT('Ctrl Pts',(-22.0217323776008,1.85809814394294,0.89247894417229));
#50107=CARTESIAN_POINT('Ctrl Pts',(-22.0587811592266,2.05325285955324,0.182208872043921));
#50108=CARTESIAN_POINT('Ctrl Pts',(-22.0958299408524,1.90536096557519,-0.44749324330245));
#50109=CARTESIAN_POINT('Ctrl Pts',(-22.1328787224782,1.75746907159715,-1.0771953586488));
#50110=CARTESIAN_POINT('Ctrl Pts',(-22.169927504104,1.26653056803076,-1.62632951721315));
#50111=CARTESIAN_POINT('Ctrl Pts',(-22.2069762857299,0.657257545813419,
-1.84354634615198));
#50112=CARTESIAN_POINT('Ctrl Pts',(-22.2440250673557,0.0479845235960825,
-2.0607631750908));
#50113=CARTESIAN_POINT('Ctrl Pts',(-22.2810738489815,-0.679623017272208,
-1.94606267440411));
#50114=CARTESIAN_POINT('Ctrl Pts',(-22.3181226306073,-1.19252496952225,
-1.55194549163459));
#50115=CARTESIAN_POINT('Ctrl Pts',(-22.3521251896968,-1.66325513049339,
-1.19023338647936));
#50116=CARTESIAN_POINT('Ctrl Pts',(-22.3861277487863,-1.95313521531399,
-0.593163978528166));
#50117=CARTESIAN_POINT('Ctrl Pts',(-22.4201303078758,-1.95665010086297,
0.000936523909256006));
#50118=CARTESIAN_POINT('Ctrl Pts',(-22.5218696921242,-1.95645680992384,
0.00107881945475618));
#50119=CARTESIAN_POINT('Ctrl Pts',(-22.4884089890719,-1.95257479207838,
-0.583706687029066));
#50120=CARTESIAN_POINT('Ctrl Pts',(-22.4549482860197,-1.67302767328136,
-1.17171185228325));
#50121=CARTESIAN_POINT('Ctrl Pts',(-22.4214875829675,-1.21504174052394,
-1.53438067071518));
#50122=CARTESIAN_POINT('Ctrl Pts',(-22.3844388013417,-0.707944780130278,
-1.935939413686));
#50123=CARTESIAN_POINT('Ctrl Pts',(-22.3473900197159,0.0179117524000019,
-2.06124389490971));
#50124=CARTESIAN_POINT('Ctrl Pts',(-22.3103412380901,0.630289220332262,
-1.85293981893982));
#50125=CARTESIAN_POINT('Ctrl Pts',(-22.2732924564642,1.24266668826453,-1.64463574296993));
#50126=CARTESIAN_POINT('Ctrl Pts',(-22.2362436748384,1.74156509159877,-1.10272310980644));
#50127=CARTESIAN_POINT('Ctrl Pts',(-22.1991948932126,1.89862893863049,-0.475245859818517));
#50128=CARTESIAN_POINT('Ctrl Pts',(-22.1621461115868,2.05569278566222,0.152231390169393));
#50129=CARTESIAN_POINT('Ctrl Pts',(-22.125097329961,1.87092207639144,0.865273256981712));
#50130=CARTESIAN_POINT('Ctrl Pts',(-22.0880485483352,1.42888995413977,1.33750662534367));
#50131=CARTESIAN_POINT('Ctrl Pts',(-22.0509997667094,0.986857831888117,
1.80973999370563));
#50132=CARTESIAN_POINT('Ctrl Pts',(-22.0139509850836,0.287564296655561,
2.04116486361724));
#50133=CARTESIAN_POINT('Ctrl Pts',(-21.9769022034578,-0.348910414746983,
1.92585357604385));
#50134=CARTESIAN_POINT('Ctrl Pts',(-21.939853421832,-0.985385126149545,
1.81054228847046));
#50135=CARTESIAN_POINT('Ctrl Pts',(-21.9028046402062,-1.5590410137221,1.34849484341207));
#50136=CARTESIAN_POINT('Ctrl Pts',(-21.8657558585804,-1.80730463285085,
0.751199333037264));
#50137=CARTESIAN_POINT('Ctrl Pts',(-21.8511271364283,-1.90533159474615,
0.515357027824685));
#50138=CARTESIAN_POINT('Ctrl Pts',(-21.8364984142762,-1.95262770521904,
0.258428636149302));
#50139=CARTESIAN_POINT('Ctrl Pts',(-21.8218696921242,-1.95136622811345,
0.00105513229623864));
#50140=CARTESIAN_POINT('Origin',(-14.8,0.,0.));
#50141=CARTESIAN_POINT('',(-21.0201303078758,-1.95236395582867,-0.0015719214144061));
#50142=CARTESIAN_POINT('',(-21.1218696921242,-1.95260904431355,-0.00164165242779367));
#50143=CARTESIAN_POINT('',(-14.8,-1.954,-2.39295984553393E-16));
#50144=CARTESIAN_POINT('Ctrl Pts',(-21.0201303078758,-1.95236395582867,
-0.0015719214144061));
#50145=CARTESIAN_POINT('Ctrl Pts',(-21.045257817569,-1.94902866231054,0.43994669109059));
#50146=CARTESIAN_POINT('Ctrl Pts',(-21.0703853272623,-1.80070766903344,
0.883494201581255));
#50147=CARTESIAN_POINT('Ctrl Pts',(-21.0955128369556,-1.52600533535847,
1.22554409483969));
#50148=CARTESIAN_POINT('Ctrl Pts',(-21.1325616185814,-1.12097567278332,
1.72987309342132));
#50149=CARTESIAN_POINT('Ctrl Pts',(-21.1696104002072,-0.441199667669119,
2.01355164611284));
#50150=CARTESIAN_POINT('Ctrl Pts',(-21.206659181833,0.202175995891084,1.94673456809716));
#50151=CARTESIAN_POINT('Ctrl Pts',(-21.2437079634588,0.845551659451288,
1.87991749008148));
#50152=CARTESIAN_POINT('Ctrl Pts',(-21.2807567450847,1.4525269814575,1.46260478135859));
#50153=CARTESIAN_POINT('Ctrl Pts',(-21.3178055267105,1.74527756483232,0.885808576178816));
#50154=CARTESIAN_POINT('Ctrl Pts',(-21.3548543083363,2.03802814820715,0.309012370999024));
#50155=CARTESIAN_POINT('Ctrl Pts',(-21.391903089962,2.01655399295056,-0.427267330637652));
#50156=CARTESIAN_POINT('Ctrl Pts',(-21.4289518715879,1.6906842371191,-0.986021004997343));
#50157=CARTESIAN_POINT('Ctrl Pts',(-21.4660006532137,1.36481448128766,-1.54477467935702));
#50158=CARTESIAN_POINT('Ctrl Pts',(-21.5030494348395,0.734549124881337,
-1.9260023264397));
#50159=CARTESIAN_POINT('Ctrl Pts',(-21.5400982164653,0.0883728661966189,
-1.95520864576116));
#50160=CARTESIAN_POINT('Ctrl Pts',(-21.5771469980911,-0.557803392488099,
-1.98441496508261));
#50161=CARTESIAN_POINT('Ctrl Pts',(-21.6141957797169,-1.21989055345123,
-1.66159995664285));
#50162=CARTESIAN_POINT('Ctrl Pts',(-21.6512445613427,-1.59483846022299,
-1.13452232139017));
#50163=CARTESIAN_POINT('Ctrl Pts',(-21.6742064768537,-1.82722186875934,
-0.807852682138515));
#50164=CARTESIAN_POINT('Ctrl Pts',(-21.6971683923647,-1.94930897921542,
-0.402721421061367));
#50165=CARTESIAN_POINT('Ctrl Pts',(-21.7201303078758,-1.95153139402954,
0.00117824056209609));
#50166=CARTESIAN_POINT('Ctrl Pts',(-21.8218696921242,-1.95136622811345,
0.00105513229623864));
#50167=CARTESIAN_POINT('Ctrl Pts',(-21.7994496326504,-1.94943288141113,
-0.393396905507871));
#50168=CARTESIAN_POINT('Ctrl Pts',(-21.7770295731767,-1.83344361255741,
-0.788894458182419));
#50169=CARTESIAN_POINT('Ctrl Pts',(-21.7546095137029,-1.61122196613715,
-1.11113196773242));
#50170=CARTESIAN_POINT('Ctrl Pts',(-21.7175607320771,-1.24400432960976,
-1.6436241824361));
#50171=CARTESIAN_POINT('Ctrl Pts',(-21.6805119504513,-0.586697705870041,
-1.97606503615226));
#50172=CARTESIAN_POINT('Ctrl Pts',(-21.6434631688255,0.0598358933747139,
-1.95628989154058));
#50173=CARTESIAN_POINT('Ctrl Pts',(-21.6064143871997,0.706369492619478,
-1.9365147469289));
#50174=CARTESIAN_POINT('Ctrl Pts',(-21.5693656055739,1.34213006736929,-1.56452360398938));
#50175=CARTESIAN_POINT('Ctrl Pts',(-21.5323168239481,1.67611765113184,-1.01058403581497));
#50176=CARTESIAN_POINT('Ctrl Pts',(-21.4952680423223,2.0101052348944,-0.456644467640561));
#50177=CARTESIAN_POINT('Ctrl Pts',(-21.4582192606965,2.04231982766971,0.279243525768716));
#50178=CARTESIAN_POINT('Ctrl Pts',(-21.4211704790707,1.75801618448586,0.860249713144712));
#50179=CARTESIAN_POINT('Ctrl Pts',(-21.3841216974449,1.47371254130201,1.4412559005207));
#50180=CARTESIAN_POINT('Ctrl Pts',(-21.347072915819,0.872890662159003,1.86738028186339));
#50181=CARTESIAN_POINT('Ctrl Pts',(-21.3100241341932,0.230558393787886,
1.94357744917298));
#50182=CARTESIAN_POINT('Ctrl Pts',(-21.2729753525674,-0.411773874583241,
2.01977461648257));
#50183=CARTESIAN_POINT('Ctrl Pts',(-21.2359265709416,-1.09561653218248,
1.74604456975904));
#50184=CARTESIAN_POINT('Ctrl Pts',(-21.1988777893158,-1.50796150906827,
1.24767886936036));
#50185=CARTESIAN_POINT('Ctrl Pts',(-21.1732084235853,-1.79365603273008,
0.902384614874454));
#50186=CARTESIAN_POINT('Ctrl Pts',(-21.1475390578547,-1.94901931302901,
0.449255022826248));
#50187=CARTESIAN_POINT('Ctrl Pts',(-21.1218696921242,-1.95260904431355,
-0.00164165242779367));
#50188=CARTESIAN_POINT('Origin',(-14.8,0.,0.));
#50189=CARTESIAN_POINT('',(-20.3201303078758,-1.95715316974838,-0.000285904946947801));
#50190=CARTESIAN_POINT('',(-20.4218696921242,-1.95719692349308,-0.00011048144072509));
#50191=CARTESIAN_POINT('',(-14.8,-1.954,-2.39295984553393E-16));
#50192=CARTESIAN_POINT('Ctrl Pts',(-20.3201303078758,-1.95715316974838,
-0.000285904946947801));
#50193=CARTESIAN_POINT('Ctrl Pts',(-20.3562984611475,-1.95586198679419,
0.631220005407538));
#50194=CARTESIAN_POINT('Ctrl Pts',(-20.3924666144193,-1.62233085199216,
1.26389725429215));
#50195=CARTESIAN_POINT('Ctrl Pts',(-20.4286347676911,-1.10004748061862,
1.618810103849));
#50196=CARTESIAN_POINT('Ctrl Pts',(-20.4656835493169,-0.565047464792199,
1.98236443189616));
#50197=CARTESIAN_POINT('Ctrl Pts',(-20.5027323309427,0.168008229422955,
2.05446358282673));
#50198=CARTESIAN_POINT('Ctrl Pts',(-20.5397811125685,0.763585769125162,
1.8021063745319));
#50199=CARTESIAN_POINT('Ctrl Pts',(-20.5768298941943,1.35916330882738,1.54974916623707));
#50200=CARTESIAN_POINT('Ctrl Pts',(-20.6138786758201,1.81726269401663,0.972935598716842));
#50201=CARTESIAN_POINT('Ctrl Pts',(-20.6509274574459,1.92820293622857,0.335684448043843));
#50202=CARTESIAN_POINT('Ctrl Pts',(-20.6879762390717,2.03914317844051,-0.301566702629146));
#50203=CARTESIAN_POINT('Ctrl Pts',(-20.7250250206975,1.80292427767512,-0.999255436454915));
#50204=CARTESIAN_POINT('Ctrl Pts',(-20.7620738023233,1.32766821402631,-1.43803606540419));
#50205=CARTESIAN_POINT('Ctrl Pts',(-20.7991225839491,0.852412150377491,
-1.87681669435347));
#50206=CARTESIAN_POINT('Ctrl Pts',(-20.836171365575,0.138118923845247,-2.05668921842628));
#50207=CARTESIAN_POINT('Ctrl Pts',(-20.8732201472008,-0.488265578640686,
-1.89532248882707));
#50208=CARTESIAN_POINT('Ctrl Pts',(-20.9102689288266,-1.11465008112663,
-1.73395575922787));
#50209=CARTESIAN_POINT('Ctrl Pts',(-20.9473177104524,-1.65312585956624,
-1.23134977595664));
#50210=CARTESIAN_POINT('Ctrl Pts',(-20.9843664920782,-1.85722208876799,
-0.617557062085145));
#50211=CARTESIAN_POINT('Ctrl Pts',(-20.9962877640107,-1.92289460327309,
-0.420055564568475));
#50212=CARTESIAN_POINT('Ctrl Pts',(-21.0082090359432,-1.95394632278384,
-0.211042080104704));
#50213=CARTESIAN_POINT('Ctrl Pts',(-21.0201303078758,-1.95236395582867,
-0.0015719214144061));
#50214=CARTESIAN_POINT('Ctrl Pts',(-21.1218696921242,-1.95260904431355,
-0.00164165242779367));
#50215=CARTESIAN_POINT('Ctrl Pts',(-21.1104902762289,-1.9542003982125,-0.201527416936542));
#50216=CARTESIAN_POINT('Ctrl Pts',(-21.0991108603336,-1.92596501442508,
-0.40097436569691));
#50217=CARTESIAN_POINT('Ctrl Pts',(-21.0877314444384,-1.8660348537741,-0.590393426775798));
#50218=CARTESIAN_POINT('Ctrl Pts',(-21.0506826628126,-1.67091592542181,
-1.20709866843947));
#50219=CARTESIAN_POINT('Ctrl Pts',(-21.0136338811868,-1.13983077254491,
-1.717507797693));
#50220=CARTESIAN_POINT('Ctrl Pts',(-20.976585099561,-0.515867387431277,
-1.88799663995057));
#50221=CARTESIAN_POINT('Ctrl Pts',(-20.9395363179352,0.108095997682367,
-2.05848548220813));
#50222=CARTESIAN_POINT('Ctrl Pts',(-20.9024875363094,0.824937615032749,
-1.88905403746973));
#50223=CARTESIAN_POINT('Ctrl Pts',(-20.8654387546836,1.30654512970301,-1.45725436967234));
#50224=CARTESIAN_POINT('Ctrl Pts',(-20.8283899730577,1.78815264437328,-1.02545470187495));
#50225=CARTESIAN_POINT('Ctrl Pts',(-20.7913411914319,2.03452605636343,-0.331286811018583));
#50226=CARTESIAN_POINT('Ctrl Pts',(-20.7542924098061,1.9328954685122,0.307515173096853));
#50227=CARTESIAN_POINT('Ctrl Pts',(-20.7172436281803,1.83126488066097,0.94631715721227));
#50228=CARTESIAN_POINT('Ctrl Pts',(-20.6801948465545,1.38163029296839,1.52975323458676));
#50229=CARTESIAN_POINT('Ctrl Pts',(-20.6431460649287,0.789798191632178,
1.7907733777266));
#50230=CARTESIAN_POINT('Ctrl Pts',(-20.6060972833029,0.197966090295949,
2.05179352086645));
#50231=CARTESIAN_POINT('Ctrl Pts',(-20.5690485016771,-0.536063524683919,
1.99039772977163));
#50232=CARTESIAN_POINT('Ctrl Pts',(-20.5319997200513,-1.07631103795058,
1.63468805081139));
#50233=CARTESIAN_POINT('Ctrl Pts',(-20.4952897107422,-1.61161855336392,
1.28223096442644));
#50234=CARTESIAN_POINT('Ctrl Pts',(-20.4585797014332,-1.95667163342788,
0.640817766737759));
#50235=CARTESIAN_POINT('Ctrl Pts',(-20.4218696921242,-1.95719692349308,
-0.00011048144072509));
#50236=CARTESIAN_POINT('Origin',(-14.8,0.,0.));
#50237=CARTESIAN_POINT('',(-19.6201303078758,-1.95320120599967,0.00175035074057674));
#50238=CARTESIAN_POINT('',(-19.7218696921242,-1.95293192181713,0.00171055984299888));
#50239=CARTESIAN_POINT('',(-14.8,-1.954,-2.39295984553393E-16));
#50240=CARTESIAN_POINT('Ctrl Pts',(-19.6201303078758,-1.95320120599967,
0.00175035074057674));
#50241=CARTESIAN_POINT('Ctrl Pts',(-19.6302903231002,-1.95475089717379,
0.180079640908608));
#50242=CARTESIAN_POINT('Ctrl Pts',(-19.6404503383247,-1.93233867926486,
0.358026458337075));
#50243=CARTESIAN_POINT('Ctrl Pts',(-19.6506103535491,-1.88441164171196,
0.528813177331473));
#50244=CARTESIAN_POINT('Ctrl Pts',(-19.6876591351749,-1.70964434963189,
1.15159175756291));
#50245=CARTESIAN_POINT('Ctrl Pts',(-19.7247079168007,-1.19560222383916,
1.67916130870918));
#50246=CARTESIAN_POINT('Ctrl Pts',(-19.7617566984265,-0.57757233201673,
1.8700429976949));
#50247=CARTESIAN_POINT('Ctrl Pts',(-19.7988054800523,0.0404575598057107,
2.06092468668063));
#50248=CARTESIAN_POINT('Ctrl Pts',(-19.8358542616782,0.762475217657862,
1.9151185135058));
#50249=CARTESIAN_POINT('Ctrl Pts',(-19.872903043304,1.25799913232614,1.49936279632572));
#50250=CARTESIAN_POINT('Ctrl Pts',(-19.9099518249298,1.7535230469944,1.08360707914564));
#50251=CARTESIAN_POINT('Ctrl Pts',(-19.9470006065556,2.02255321847879,0.397901817960317));
#50252=CARTESIAN_POINT('Ctrl Pts',(-19.9840493881814,1.94194931062656,-0.243892367441067));
#50253=CARTESIAN_POINT('Ctrl Pts',(-20.0210981698072,1.86134540277432,-0.885686552842469));
#50254=CARTESIAN_POINT('Ctrl Pts',(-20.058146951433,1.43110741558543,-1.48356966245993));
#50255=CARTESIAN_POINT('Ctrl Pts',(-20.0951957330588,0.848163634373811,
-1.76387898146806));
#50256=CARTESIAN_POINT('Ctrl Pts',(-20.1322445146846,0.265219853162208,
-2.04418830047618));
#50257=CARTESIAN_POINT('Ctrl Pts',(-20.1692932963104,-0.470429722072116,
-2.00692382887498));
#50258=CARTESIAN_POINT('Ctrl Pts',(-20.2063420779362,-1.0220639886916,-1.66914223928304));
#50259=CARTESIAN_POINT('Ctrl Pts',(-20.243390859562,-1.5736982553111,-1.33136064969109));
#50260=CARTESIAN_POINT('Ctrl Pts',(-20.2804396411878,-1.94131721331576,
-0.693061942108369));
#50261=CARTESIAN_POINT('Ctrl Pts',(-20.3174884228136,-1.95665452359924,
-0.046407835735133));
#50262=CARTESIAN_POINT('Ctrl Pts',(-20.3183690511677,-1.95701908269451,
-0.0310372373959162));
#50263=CARTESIAN_POINT('Ctrl Pts',(-20.3192496795217,-1.95718460769079,
-0.0156619183757309));
#50264=CARTESIAN_POINT('Ctrl Pts',(-20.3201303078758,-1.95715316974838,
-0.000285904946947801));
#50265=CARTESIAN_POINT('Ctrl Pts',(-20.4218696921242,-1.95719692349308,
-0.00011048144072509));
#50266=CARTESIAN_POINT('Ctrl Pts',(-20.4215309198074,-1.95720177104653,
-0.00602518295147257));
#50267=CARTESIAN_POINT('Ctrl Pts',(-20.4211921474906,-1.95717727785765,
-0.0119398431628558));
#50268=CARTESIAN_POINT('Ctrl Pts',(-20.4208533751739,-1.95712332268219,
-0.01785423460159));
#50269=CARTESIAN_POINT('Ctrl Pts',(-20.383804593548,-1.9512226825937,-0.664663274228705));
#50270=CARTESIAN_POINT('Ctrl Pts',(-20.3467558119222,-1.59295599086327,
-1.30825778665728));
#50271=CARTESIAN_POINT('Ctrl Pts',(-20.3097070302964,-1.04630887262954,
-1.65405205992329));
#50272=CARTESIAN_POINT('Ctrl Pts',(-20.2726582486706,-0.499661754395827,
-1.99984633318929));
#50273=CARTESIAN_POINT('Ctrl Pts',(-20.2356094670448,0.235365790341175,
-2.04784036729274));
#50274=CARTESIAN_POINT('Ctrl Pts',(-20.198560685419,0.822337374387208,-1.77606636040598));
#50275=CARTESIAN_POINT('Ctrl Pts',(-20.1615119037932,1.40930895843324,-1.50429235351922));
#50276=CARTESIAN_POINT('Ctrl Pts',(-20.1244631221674,1.8482245817883,-0.91275030564226));
#50277=CARTESIAN_POINT('Ctrl Pts',(-20.0874143405416,1.93818403647784,-0.272200504448977));
#50278=CARTESIAN_POINT('Ctrl Pts',(-20.0503655589158,2.02814349116737,0.368349296744315));
#50279=CARTESIAN_POINT('Ctrl Pts',(-20.01331677729,1.76914677719136,1.05790685125393));
#50280=CARTESIAN_POINT('Ctrl Pts',(-19.9762679956642,1.279741722273,1.48084826979456));
#50281=CARTESIAN_POINT('Ctrl Pts',(-19.9392192140384,0.790336667354642,
1.90378968833517));
#50282=CARTESIAN_POINT('Ctrl Pts',(-19.9021704324125,0.070523271493932,
2.06011497090681));
#50283=CARTESIAN_POINT('Ctrl Pts',(-19.8651216507867,-0.550225889632995,
1.87827099862011));
#50284=CARTESIAN_POINT('Ctrl Pts',(-19.8280728691609,-1.17097505075993,
1.6964270263334));
#50285=CARTESIAN_POINT('Ctrl Pts',(-19.7910240875351,-1.69265997715308,
1.17641379918833));
#50286=CARTESIAN_POINT('Ctrl Pts',(-19.7539753059093,-1.87649534281188,
0.556251473962188));
#50287=CARTESIAN_POINT('Ctrl Pts',(-19.7432734346476,-1.92959782905559,
0.37711205089107));
#50288=CARTESIAN_POINT('Ctrl Pts',(-19.7325715633859,-1.95451032397123,
0.189616239253742));
#50289=CARTESIAN_POINT('Ctrl Pts',(-19.7218696921242,-1.95293192181713,
0.00171055984299888));
#50290=CARTESIAN_POINT('Origin',(-14.8,0.,0.));
#50291=CARTESIAN_POINT('',(-18.9201303078757,-1.95106696972105,-0.00075047970158143));
#50292=CARTESIAN_POINT('',(-19.0218696921242,-1.95118717389941,-0.00089009348416731));
#50293=CARTESIAN_POINT('',(-14.8,-1.954,-2.39295984553393E-16));
#50294=CARTESIAN_POINT('Ctrl Pts',(-18.9201303078757,-1.95106696972105,
-0.00075047970158143));
#50295=CARTESIAN_POINT('Ctrl Pts',(-18.9413309666787,-1.94977826652978,
0.372390924373151));
#50296=CARTESIAN_POINT('Ctrl Pts',(-18.9625316254816,-1.84685029020357,
0.74619065026788));
#50297=CARTESIAN_POINT('Ctrl Pts',(-18.9837322842846,-1.64683197629078,
1.05763654144758));
#50298=CARTESIAN_POINT('Ctrl Pts',(-19.0207810659104,-1.29729402550354,
1.60189749662951));
#50299=CARTESIAN_POINT('Ctrl Pts',(-19.0578298475362,-0.651255759954327,
1.95573855958341));
#50300=CARTESIAN_POINT('Ctrl Pts',(-19.094878629162,-0.0044214448872297,
1.95719980144187));
#50301=CARTESIAN_POINT('Ctrl Pts',(-19.1319274107878,0.642412870179858,
1.95866104330033));
#50302=CARTESIAN_POINT('Ctrl Pts',(-19.1689761924136,1.29004323476483,1.60774246406337));
#50303=CARTESIAN_POINT('Ctrl Pts',(-19.2060249740394,1.64203664896396,1.06506631502371));
#50304=CARTESIAN_POINT('Ctrl Pts',(-19.2430737556652,1.99403006316311,0.522390165984023));
#50305=CARTESIAN_POINT('Ctrl Pts',(-19.280122537291,2.05038652697639,-0.212043552858375));
#50306=CARTESIAN_POINT('Ctrl Pts',(-19.3171713189168,1.78531059203435,-0.802070259957907));
#50307=CARTESIAN_POINT('Ctrl Pts',(-19.3542201005426,1.52023465709232,-1.39209696705742));
#50308=CARTESIAN_POINT('Ctrl Pts',(-19.3912688821684,0.933726323394989,
-1.83771666241408));
#50309=CARTESIAN_POINT('Ctrl Pts',(-19.4283176637943,0.294241849842236,
-1.93496055405282));
#50310=CARTESIAN_POINT('Ctrl Pts',(-19.4653664454201,-0.345242623710509,
-2.03220444569156));
#50311=CARTESIAN_POINT('Ctrl Pts',(-19.5024152270459,-1.03770323711868,
-1.78107253361239));
#50312=CARTESIAN_POINT('Ctrl Pts',(-19.5394640086717,-1.46618731463906,
-1.29651277291452));
#50313=CARTESIAN_POINT('Ctrl Pts',(-19.566352775073,-1.77716672506918,-0.944835507397405));
#50314=CARTESIAN_POINT('Ctrl Pts',(-19.5932415414744,-1.94909990466747,
-0.47020313750915));
#50315=CARTESIAN_POINT('Ctrl Pts',(-19.6201303078758,-1.95320120599967,
0.00175035074057674));
#50316=CARTESIAN_POINT('Ctrl Pts',(-19.7218696921242,-1.95293192181713,
0.00171055984299888));
#50317=CARTESIAN_POINT('Ctrl Pts',(-19.6955227817601,-1.94904605746169,
-0.460893967091506));
#50318=CARTESIAN_POINT('Ctrl Pts',(-19.669175871396,-1.78460047078708,-0.925982677770864));
#50319=CARTESIAN_POINT('Ctrl Pts',(-19.6428289610319,-1.48494804682834,
-1.27498226344545));
#50320=CARTESIAN_POINT('Ctrl Pts',(-19.6057801794061,-1.06357958026152,
-1.76574225231978));
#50321=CARTESIAN_POINT('Ctrl Pts',(-19.5687313977803,-0.374856842203399,
-2.0269508067612));
#50322=CARTESIAN_POINT('Ctrl Pts',(-19.5316826161545,0.265978389769201,
-1.93904769669433));
#50323=CARTESIAN_POINT('Ctrl Pts',(-19.4946338345287,0.9068136217418,-1.85114458662745));
#50324=CARTESIAN_POINT('Ctrl Pts',(-19.4575850529028,1.49976134762888,-1.41412981205228));
#50325=CARTESIAN_POINT('Ctrl Pts',(-19.420536271277,1.77341787362209,-0.828033525527501));
#50326=CARTESIAN_POINT('Ctrl Pts',(-19.3834874896512,2.0470743996153,-0.241937239002725));
#50327=CARTESIAN_POINT('Ctrl Pts',(-19.3464387080254,2.00143972571464,0.493240559471652));
#50328=CARTESIAN_POINT('Ctrl Pts',(-19.3093899263996,1.65740172874576,1.04099470864667));
#50329=CARTESIAN_POINT('Ctrl Pts',(-19.2723411447738,1.31336373177689,1.58874885782166));
#50330=CARTESIAN_POINT('Ctrl Pts',(-19.235292363148,0.670922411739813,1.94907935769732));
#50331=CARTESIAN_POINT('Ctrl Pts',(-19.1982435815222,0.0241356420369828,
1.95705593805166));
#50332=CARTESIAN_POINT('Ctrl Pts',(-19.1611947998964,-0.622651127665885,
1.965032518406));
#50333=CARTESIAN_POINT('Ctrl Pts',(-19.1241460182706,-1.27378334703449,
1.62065517923901));
#50334=CARTESIAN_POINT('Ctrl Pts',(-19.0870972366448,-1.63122514919733,
1.08155211918147));
#50335=CARTESIAN_POINT('Ctrl Pts',(-19.0653547218046,-1.84099409022561,
0.765173124533693));
#50336=CARTESIAN_POINT('Ctrl Pts',(-19.0436122069644,-1.94961406105061,
0.381729271837227));
#50337=CARTESIAN_POINT('Ctrl Pts',(-19.0218696921242,-1.95118717389941,
-0.00089009348416731));
#50338=CARTESIAN_POINT('Origin',(-14.8,0.,0.));
#50339=CARTESIAN_POINT('',(-18.2201303078757,-1.955948595666,-0.0013580538473823));
#50340=CARTESIAN_POINT('',(-18.3218696921242,-1.9561856368743,-0.00124144867156942));
#50341=CARTESIAN_POINT('',(-14.8,-1.954,-2.39295984553393E-16));
#50342=CARTESIAN_POINT('Ctrl Pts',(-18.2201303078757,-1.955948595666,-0.0013580538473823));
#50343=CARTESIAN_POINT('Ctrl Pts',(-18.2523716102572,-1.95148176910926,
0.562500491288516));
#50344=CARTESIAN_POINT('Ctrl Pts',(-18.2846129126386,-1.69434583291202,
1.12991216153671));
#50345=CARTESIAN_POINT('Ctrl Pts',(-18.31685421502,-1.26476057883309,1.49366371388234));
#50346=CARTESIAN_POINT('Ctrl Pts',(-18.3539029966458,-0.771120152036655,
1.91165401928226));
#50347=CARTESIAN_POINT('Ctrl Pts',(-18.3909517782716,-0.0497686319888131,
2.06072085969571));
#50348=CARTESIAN_POINT('Ctrl Pts',(-18.4280005598974,0.569117376311475,
1.87263344622468));
#50349=CARTESIAN_POINT('Ctrl Pts',(-18.4650493415233,1.18800338461177,1.68454603275365));
#50350=CARTESIAN_POINT('Ctrl Pts',(-18.5020981231491,1.70442388116452,1.15930436539812));
#50351=CARTESIAN_POINT('Ctrl Pts',(-18.5391469047749,1.8820031717834,0.537321759596808));
#50352=CARTESIAN_POINT('Ctrl Pts',(-18.5761956864007,2.05958246240227,-0.0846608462045072));
#50353=CARTESIAN_POINT('Ctrl Pts',(-18.6132444680265,1.89832054708729,-0.803384390451597));
#50354=CARTESIAN_POINT('Ctrl Pts',(-18.6502932496523,1.47203013744235,-1.28987514372533));
#50355=CARTESIAN_POINT('Ctrl Pts',(-18.6873420312781,1.04573972779741,-1.77636589699906));
#50356=CARTESIAN_POINT('Ctrl Pts',(-18.7243908129039,0.354420823822513,
-2.03062385929941));
#50357=CARTESIAN_POINT('Ctrl Pts',(-18.7614395945297,-0.285496481327623,
-1.93627022160868));
#50358=CARTESIAN_POINT('Ctrl Pts',(-18.7984883761555,-0.92541378647776,
-1.84191658391795));
#50359=CARTESIAN_POINT('Ctrl Pts',(-18.8355371577813,-1.51392949280315,
-1.39895134623613));
#50360=CARTESIAN_POINT('Ctrl Pts',(-18.8725859394071,-1.78166852795321,
-0.810128303690238));
#50361=CARTESIAN_POINT('Ctrl Pts',(-18.88843406223,-1.89619756041618,-0.558251197623553));
#50362=CARTESIAN_POINT('Ctrl Pts',(-18.9042821850529,-1.95203031367405,
-0.279684774010249));
#50363=CARTESIAN_POINT('Ctrl Pts',(-18.9201303078757,-1.95106696972105,
-0.00075047970158143));
#50364=CARTESIAN_POINT('Ctrl Pts',(-19.0218696921242,-1.95118717389941,
-0.00089009348416731));
#50365=CARTESIAN_POINT('Ctrl Pts',(-19.0065634253386,-1.95229461179813,
-0.270245967263792));
#50366=CARTESIAN_POINT('Ctrl Pts',(-18.991257158553,-1.90035112825074,-0.539193236664031));
#50367=CARTESIAN_POINT('Ctrl Pts',(-18.9759508917673,-1.7932990566245,-0.784046533943919));
#50368=CARTESIAN_POINT('Ctrl Pts',(-18.9389021101415,-1.53417977693178,
-1.37671334606378));
#50369=CARTESIAN_POINT('Ctrl Pts',(-18.9018533285157,-0.952189832589261,
-1.82821818935548));
#50370=CARTESIAN_POINT('Ctrl Pts',(-18.8648045468899,-0.31371732790678,
-1.93189852529858));
#50371=CARTESIAN_POINT('Ctrl Pts',(-18.8277557652641,0.32475517677571,-2.03557886124168));
#50372=CARTESIAN_POINT('Ctrl Pts',(-18.7907069836383,1.01971024179817,-1.7914346898362));
#50373=CARTESIAN_POINT('Ctrl Pts',(-18.7536582020125,1.45305343245182,-1.31121554151855));
#50374=CARTESIAN_POINT('Ctrl Pts',(-18.7166094203867,1.88639662310545,-0.830996393200911));
#50375=CARTESIAN_POINT('Ctrl Pts',(-18.6795606387609,2.05812793939028,-0.114702267971124));
#50376=CARTESIAN_POINT('Ctrl Pts',(-18.6425118571351,1.88964262148106,0.509805097034146));
#50377=CARTESIAN_POINT('Ctrl Pts',(-18.6054630755093,1.72115730357184,1.13431246203942));
#50378=CARTESIAN_POINT('Ctrl Pts',(-18.5684142938834,1.21245535146857,1.66703306682015));
#50379=CARTESIAN_POINT('Ctrl Pts',(-18.5313655122576,0.596379531608711,
1.86413034097886));
#50380=CARTESIAN_POINT('Ctrl Pts',(-18.4943167306318,-0.0196962882511521,
2.06122761513757));
#50381=CARTESIAN_POINT('Ctrl Pts',(-18.457267949006,-0.743145975867633,
1.92270155867423));
#50382=CARTESIAN_POINT('Ctrl Pts',(-18.4202191673802,-1.24283255418279,
1.51195823888865));
#50383=CARTESIAN_POINT('Ctrl Pts',(-18.3874360089615,-1.6849875600356,1.14850598132321));
#50384=CARTESIAN_POINT('Ctrl Pts',(-18.3546528505428,-1.95193929414975,
0.571911551633334));
#50385=CARTESIAN_POINT('Ctrl Pts',(-18.3218696921242,-1.9561856368743,-0.00124144867156942));
#50386=CARTESIAN_POINT('Origin',(-14.8,0.,0.));
#50387=CARTESIAN_POINT('',(-17.5201303078758,-1.95526004210547,0.001601638831479));
#50388=CARTESIAN_POINT('',(-17.6218696921242,-1.95498100154377,0.00166857518573596));
#50389=CARTESIAN_POINT('',(-14.8,-1.954,-2.39295984553393E-16));
#50390=CARTESIAN_POINT('Ctrl Pts',(-17.5201303078758,-1.95526004210547,
0.001601638831479));
#50391=CARTESIAN_POINT('Ctrl Pts',(-17.5263634722099,-1.95622626701164,
0.110711495172787));
#50392=CARTESIAN_POINT('Ctrl Pts',(-17.532596636544,-1.94788014460328,0.219673489375271));
#50393=CARTESIAN_POINT('Ctrl Pts',(-17.5388298008781,-1.92969991498865,
0.32696918819943));
#50394=CARTESIAN_POINT('Ctrl Pts',(-17.5758785825039,-1.82163997612026,
0.964715074887744));
#50395=CARTESIAN_POINT('Ctrl Pts',(-17.6129273641297,-1.36615137395922,
1.54359249860331));
#50396=CARTESIAN_POINT('Ctrl Pts',(-17.6499761457555,-0.771720090856103,
1.79863801619671));
#50397=CARTESIAN_POINT('Ctrl Pts',(-17.6870249273813,-0.177288807752993,
2.0536835337901));
#50398=CARTESIAN_POINT('Ctrl Pts',(-17.7240737090071,0.556085156292187,
1.98489714526133));
#50399=CARTESIAN_POINT('Ctrl Pts',(-17.7611224906329,1.09272229009327,1.6237637170082));
#50400=CARTESIAN_POINT('Ctrl Pts',(-17.7981712722587,1.62935942389434,1.26263028875509));
#50401=CARTESIAN_POINT('Ctrl Pts',(-17.8352200538845,1.96925972745132,0.609149820777612));
#50402=CARTESIAN_POINT('Ctrl Pts',(-17.8722688355103,1.95684422831105,-0.0375669810430752));
#50403=CARTESIAN_POINT('Ctrl Pts',(-17.9093176171361,1.94442872917078,-0.68428378286379));
#50404=CARTESIAN_POINT('Ctrl Pts',(-17.9463663987619,1.57969742733327,-1.3242369185277));
#50405=CARTESIAN_POINT('Ctrl Pts',(-17.9834151803877,1.0295949255763,-1.66450740495995));
#50406=CARTESIAN_POINT('Ctrl Pts',(-18.0204639620136,0.479492423819356,
-2.00477789139219));
#50407=CARTESIAN_POINT('Ctrl Pts',(-18.0575127436394,-0.255981277857039,
-2.04536572859275));
#50408=CARTESIAN_POINT('Ctrl Pts',(-18.0945615252652,-0.840185577559581,
-1.76769307494255));
#50409=CARTESIAN_POINT('Ctrl Pts',(-18.131610306891,-1.42438987726213,-1.49002042129235));
#50410=CARTESIAN_POINT('Ctrl Pts',(-18.1686590885168,-1.85732477499085,
-0.894087276791399));
#50411=CARTESIAN_POINT('Ctrl Pts',(-18.2057078701426,-1.9408275570827,-0.252663819347713));
#50412=CARTESIAN_POINT('Ctrl Pts',(-18.210515349387,-1.95166294421661,-0.169432203537293));
#50413=CARTESIAN_POINT('Ctrl Pts',(-18.2153228286314,-1.95661464121546,
-0.0854346280639692));
#50414=CARTESIAN_POINT('Ctrl Pts',(-18.2201303078757,-1.955948595666,-0.0013580538473823));
#50415=CARTESIAN_POINT('Ctrl Pts',(-18.3218696921242,-1.9561856368743,-0.00124144867156942));
#50416=CARTESIAN_POINT('Ctrl Pts',(-18.317604068917,-1.95673815526926,-0.0758179952051893));
#50417=CARTESIAN_POINT('Ctrl Pts',(-18.3133384457099,-1.95284300545396,
-0.15033627747559));
#50418=CARTESIAN_POINT('Ctrl Pts',(-18.3090728225028,-1.94430742887076,
-0.224319183124746));
#50419=CARTESIAN_POINT('Ctrl Pts',(-18.272024040877,-1.87017225622972,-0.866892702244762));
#50420=CARTESIAN_POINT('Ctrl Pts',(-18.2349752592512,-1.44597844193375,
-1.46907915737697));
#50421=CARTESIAN_POINT('Ctrl Pts',(-18.1979264776254,-0.865887735938719,
-1.75524610884933));
#50422=CARTESIAN_POINT('Ctrl Pts',(-18.1608776959996,-0.285797029943679,
-2.04141306032169));
#50423=CARTESIAN_POINT('Ctrl Pts',(-18.1238289143738,0.450190567750422,
-2.01156050813421));
#50424=CARTESIAN_POINT('Ctrl Pts',(-18.086780132748,1.00519923505916,-1.6793525453925));
#50425=CARTESIAN_POINT('Ctrl Pts',(-18.0497313511221,1.56020790236788,-1.3471445826508));
#50426=CARTESIAN_POINT('Ctrl Pts',(-18.0126825694963,1.93423763929124,-0.712581209354875));
#50427=CARTESIAN_POINT('Ctrl Pts',(-17.9756337878705,1.95608776866446,-0.0661144096325921));
#50428=CARTESIAN_POINT('Ctrl Pts',(-17.9385850062447,1.97793789803769,0.580352390089681));
#50429=CARTESIAN_POINT('Ctrl Pts',(-17.9015362246189,1.64760841986083,1.23872261623831));
#50430=CARTESIAN_POINT('Ctrl Pts',(-17.8644874429931,1.11629755387044,1.60764742562002));
#50431=CARTESIAN_POINT('Ctrl Pts',(-17.8274386613673,0.584986687880032,
1.97657223500173));
#50432=CARTESIAN_POINT('Ctrl Pts',(-17.7903898797415,-0.147305565923918,
2.0560516276165));
#50433=CARTESIAN_POINT('Ctrl Pts',(-17.7533410981157,-0.745394816147864,
1.80970634135478));
#50434=CARTESIAN_POINT('Ctrl Pts',(-17.7162923164899,-1.34348406637179,
1.56336105509306));
#50435=CARTESIAN_POINT('Ctrl Pts',(-17.6792435348641,-1.80737031301573,
0.991191089954906));
#50436=CARTESIAN_POINT('Ctrl Pts',(-17.6421947532383,-1.92472380870155,
0.355089754987665));
#50437=CARTESIAN_POINT('Ctrl Pts',(-17.6354197328669,-1.94618395635101,
0.238767454670661));
#50438=CARTESIAN_POINT('Ctrl Pts',(-17.6286447124955,-1.95605585986643,
0.120307254488911));
#50439=CARTESIAN_POINT('Ctrl Pts',(-17.6218696921242,-1.95498100154377,
0.00166857518573596));
#50440=CARTESIAN_POINT('Origin',(-14.8,0.,0.));
#50441=CARTESIAN_POINT('',(-16.8201303078758,-1.95085314384129,0.000359159457361397));
#50442=CARTESIAN_POINT('',(-16.9218696921242,-1.9508121187761,0.000204457844419397));
#50443=CARTESIAN_POINT('',(-14.8,-1.954,-2.39295984553393E-16));
#50444=CARTESIAN_POINT('Ctrl Pts',(-16.8201303078758,-1.95085314384129,
0.000359159457361397));
#50445=CARTESIAN_POINT('Ctrl Pts',(-16.8374041157883,-1.95135253313437,
0.304469385080169));
#50446=CARTESIAN_POINT('Ctrl Pts',(-16.8546779237009,-1.88453897682348,
0.608371903822219));
#50447=CARTESIAN_POINT('Ctrl Pts',(-16.8719517316135,-1.74926193216667,
0.87791417838619));
#50448=CARTESIAN_POINT('Ctrl Pts',(-16.9090005132393,-1.4591203657074,1.45602717580853));
#50449=CARTESIAN_POINT('Ctrl Pts',(-16.9460492948651,-0.854036703785103,
1.87607800661458));
#50450=CARTESIAN_POINT('Ctrl Pts',(-16.9830980764909,-0.210969493905966,
1.9458012448809));
#50451=CARTESIAN_POINT('Ctrl Pts',(-17.0201468581168,0.432097715973189,
2.01552448314721));
#50452=CARTESIAN_POINT('Ctrl Pts',(-17.0571956397426,1.11314847380918,1.73492012887377));
#50453=CARTESIAN_POINT('Ctrl Pts',(-17.0942444213684,1.52045261642256,1.2324262465368));
#50454=CARTESIAN_POINT('Ctrl Pts',(-17.1312932029942,1.92775675903592,0.72993236419984));
#50455=CARTESIAN_POINT('Ctrl Pts',(-17.16834198462,2.06131428642669,0.00554895379934056));
#50456=CARTESIAN_POINT('Ctrl Pts',(-17.2053907662458,1.85999332357917,-0.609159624548341));
#50457=CARTESIAN_POINT('Ctrl Pts',(-17.2424395478716,1.65867236073165,-1.22386820289605));
#50458=CARTESIAN_POINT('Ctrl Pts',(-17.2794883294974,1.12247290764584,-1.72890194919093));
#50459=CARTESIAN_POINT('Ctrl Pts',(-17.3165371111232,0.496823871174823,
-1.89309710605923));
#50460=CARTESIAN_POINT('Ctrl Pts',(-17.353585892749,-0.128825165296163,
-2.05729226292753));
#50461=CARTESIAN_POINT('Ctrl Pts',(-17.3906346743748,-0.843923785152349,
-1.88064883036924));
#50462=CARTESIAN_POINT('Ctrl Pts',(-17.4276834560006,-1.32115745729256,
-1.44401993925958));
#50463=CARTESIAN_POINT('Ctrl Pts',(-17.4584990732923,-1.71810034054097,
-1.0808504039471));
#50464=CARTESIAN_POINT('Ctrl Pts',(-17.489314690584,-1.95048320399723,-0.537817409912763));
#50465=CARTESIAN_POINT('Ctrl Pts',(-17.5201303078758,-1.95526004210547,
0.001601638831479));
#50466=CARTESIAN_POINT('Ctrl Pts',(-17.6218696921242,-1.95498100154377,
0.00166857518573596));
#50467=CARTESIAN_POINT('Ctrl Pts',(-17.5915959308697,-1.95017806332973,
-0.528461056297915));
#50468=CARTESIAN_POINT('Ctrl Pts',(-17.5613221696153,-1.72680176835567,
-1.06215437001553));
#50469=CARTESIAN_POINT('Ctrl Pts',(-17.5310484083608,-1.34208584047146,
-1.42458979032064));
#50470=CARTESIAN_POINT('Ctrl Pts',(-17.493999626735,-0.871273631827864,
-1.86813529586539));
#50471=CARTESIAN_POINT('Ctrl Pts',(-17.4569508451092,-0.158828469813003,
-2.05519360215856));
#50472=CARTESIAN_POINT('Ctrl Pts',(-17.4199020634834,0.469149653676805,
-1.90014448827839));
#50473=CARTESIAN_POINT('Ctrl Pts',(-17.3828532818576,1.0971277771666,-1.74509537439822));
#50474=CARTESIAN_POINT('Ctrl Pts',(-17.3458045002318,1.64063886213135,-1.24793884034472));
#50475=CARTESIAN_POINT('Ctrl Pts',(-17.308755718606,1.85090732575802,-0.636233090411912));
#50476=CARTESIAN_POINT('Ctrl Pts',(-17.2717069369802,2.06117578938469,-0.0245273404790851));
#50477=CARTESIAN_POINT('Ctrl Pts',(-17.2346581553544,1.9382016316733,0.701727625333045));
#50478=CARTESIAN_POINT('Ctrl Pts',(-17.1976093737286,1.53827251372567,1.21011079963609));
#50479=CARTESIAN_POINT('Ctrl Pts',(-17.1605605921028,1.13834339577805,1.71849397393913));
#50480=CARTESIAN_POINT('Ctrl Pts',(-17.1235118104769,0.461459317594161,
2.00900535673306));
#50481=CARTESIAN_POINT('Ctrl Pts',(-17.0864630288511,-0.18255672787268,
1.94867224411603));
#50482=CARTESIAN_POINT('Ctrl Pts',(-17.0494142472253,-0.826572773339502,
1.88833913149901));
#50483=CARTESIAN_POINT('Ctrl Pts',(-17.0123654655995,-1.4377207860893,1.47716152347106));
#50484=CARTESIAN_POINT('Ctrl Pts',(-16.9753166839737,-1.73626644742514,
0.903343399502911));
#50485=CARTESIAN_POINT('Ctrl Pts',(-16.9575010200239,-1.87982823117732,
0.627411225316896));
#50486=CARTESIAN_POINT('Ctrl Pts',(-16.939685356074,-1.95110497856138,0.313870646854676));
#50487=CARTESIAN_POINT('Ctrl Pts',(-16.9218696921242,-1.9508121187761,0.000204457844419397));
#50488=CARTESIAN_POINT('Origin',(-14.8,0.,0.));
#50489=CARTESIAN_POINT('',(-16.1201303078758,-1.95394212134825,-0.00178662227266063));
#50490=CARTESIAN_POINT('',(-16.2218696921242,-1.95423044051614,-0.00177357873807178));
#50491=CARTESIAN_POINT('',(-14.8,-1.954,-2.39295984553393E-16));
#50492=CARTESIAN_POINT('Ctrl Pts',(-16.1201303078758,-1.95394212134825,
-0.00178662227266063));
#50493=CARTESIAN_POINT('Ctrl Pts',(-16.1484447593668,-1.94939007196124,
0.494710652380524));
#50494=CARTESIAN_POINT('Ctrl Pts',(-16.1767592108579,-1.75678535459633,
0.994349447558111));
#50495=CARTESIAN_POINT('Ctrl Pts',(-16.205073662349,-1.41534509418331,1.35183167454762));
#50496=CARTESIAN_POINT('Ctrl Pts',(-16.2421224439748,-0.968578691158015,
1.8195886066223));
#50497=CARTESIAN_POINT('Ctrl Pts',(-16.2791712256006,-0.266989530277769,
2.04395791762872));
#50498=CARTESIAN_POINT('Ctrl Pts',(-16.3162200072264,0.368291399188672,
1.92224141491713));
#50499=CARTESIAN_POINT('Ctrl Pts',(-16.3532687888522,1.00357232865512,1.80052491220555));
#50500=CARTESIAN_POINT('Ctrl Pts',(-16.390317570478,1.57254502670776,1.33272259577594));
#50501=CARTESIAN_POINT('Ctrl Pts',(-16.4273663521038,1.81477963556009,0.732956674228));
#50502=CARTESIAN_POINT('Ctrl Pts',(-16.4644151337296,2.05701424441242,0.13319075268005));
#50503=CARTESIAN_POINT('Ctrl Pts',(-16.5014639153554,1.97251076406445,-0.598538773986235));
#50504=CARTESIAN_POINT('Ctrl Pts',(-16.5385126969812,1.59994807918817,-1.12730508552081));
#50505=CARTESIAN_POINT('Ctrl Pts',(-16.5755614786071,1.22738539431189,-1.65607139705536));
#50506=CARTESIAN_POINT('Ctrl Pts',(-16.6126102602329,0.566763504907309,
-1.98187449345821));
#50507=CARTESIAN_POINT('Ctrl Pts',(-16.6496590418587,-0.0795381158151578,
-1.95558796786837));
#50508=CARTESIAN_POINT('Ctrl Pts',(-16.6867078234845,-0.725839736537652,
-1.92930144227853));
#50509=CARTESIAN_POINT('Ctrl Pts',(-16.7237566051103,-1.35782108857803,
-1.550925294696));
#50510=CARTESIAN_POINT('Ctrl Pts',(-16.7608053867361,-1.68621202910011,
-0.993649638885402));
#50511=CARTESIAN_POINT('Ctrl Pts',(-16.7805803604493,-1.86149234687336,
-0.69620095201697));
#50512=CARTESIAN_POINT('Ctrl Pts',(-16.8003553341625,-1.95028144533721,
-0.347784790506909));
#50513=CARTESIAN_POINT('Ctrl Pts',(-16.8201303078758,-1.95085314384129,
0.000359159457361397));
#50514=CARTESIAN_POINT('Ctrl Pts',(-16.9218696921242,-1.9508121187761,0.000204457844419397));
#50515=CARTESIAN_POINT('Ctrl Pts',(-16.9026365744482,-1.95049595841696,
-0.338417708648121));
#50516=CARTESIAN_POINT('Ctrl Pts',(-16.8834034567723,-1.86676867152405,
-0.677186268529284));
#50517=CARTESIAN_POINT('Ctrl Pts',(-16.8641703390963,-1.7005303973301,-0.968941092964963));
#50518=CARTESIAN_POINT('Ctrl Pts',(-16.8271215574705,-1.38030537597732,
-1.53094882155632));
#50519=CARTESIAN_POINT('Ctrl Pts',(-16.7900727758447,-0.753912023349896,
-1.91850563883067));
#50520=CARTESIAN_POINT('Ctrl Pts',(-16.7530239942189,-0.108062746390163,
-1.95421926014519));
#50521=CARTESIAN_POINT('Ctrl Pts',(-16.7159752125931,0.537786530569552,
-1.98993288145971));
#50522=CARTESIAN_POINT('Ctrl Pts',(-16.6789264309673,1.20309173186161,-1.67380330681439));
#50523=CARTESIAN_POINT('Ctrl Pts',(-16.6418776493414,1.58332974143817,-1.1505291842266));
#50524=CARTESIAN_POINT('Ctrl Pts',(-16.6048288677156,1.96356775101474,-0.627255061638789));
#50525=CARTESIAN_POINT('Ctrl Pts',(-16.5677800860898,2.05873856887587,0.103163608891498));
#50526=CARTESIAN_POINT('Ctrl Pts',(-16.530731304464,1.8252806627269,0.706400011434759));
#50527=CARTESIAN_POINT('Ctrl Pts',(-16.4936825228382,1.59182275657793,1.30963641397803));
#50528=CARTESIAN_POINT('Ctrl Pts',(-16.4566337412124,1.02973612641886,1.78569054853423));
#50529=CARTESIAN_POINT('Ctrl Pts',(-16.4195849595866,0.396298742980112,
1.91666318903248));
#50530=CARTESIAN_POINT('Ctrl Pts',(-16.3825361779608,-0.237138640458614,
2.04763582953073));
#50531=CARTESIAN_POINT('Ctrl Pts',(-16.345487396335,-0.941926777176993,
1.83352697597105));
#50532=CARTESIAN_POINT('Ctrl Pts',(-16.3084386147092,-1.39547044451608,
1.37233841029168));
#50533=CARTESIAN_POINT('Ctrl Pts',(-16.2795823071808,-1.74872350623489,
1.01313094122532));
#50534=CARTESIAN_POINT('Ctrl Pts',(-16.2507259996525,-1.94956070655241,
0.504034134293982));
#50535=CARTESIAN_POINT('Ctrl Pts',(-16.2218696921242,-1.95423044051614,
-0.00177357873807178));
#50536=CARTESIAN_POINT('Origin',(-14.8,0.,0.));
#50537=CARTESIAN_POINT('',(-15.4201303078757,-1.95687456006756,0.000726948241557314));
#50538=CARTESIAN_POINT('',(-15.5218696921242,-1.95671484857984,0.000882047759029596));
#50539=CARTESIAN_POINT('',(-14.8,-1.954,-2.39295984553393E-16));
#50540=CARTESIAN_POINT('Ctrl Pts',(-15.4201303078757,-1.95687456006756,
0.000726948241557314));
#50541=CARTESIAN_POINT('Ctrl Pts',(-15.4224366213195,-1.95706686879056,
0.0410111310332522));
#50542=CARTESIAN_POINT('Ctrl Pts',(-15.4247429347632,-1.95593068181528,
0.0812842614253603));
#50543=CARTESIAN_POINT('Ctrl Pts',(-15.427049248207,-1.95343159833963,0.121472641147085));
#50544=CARTESIAN_POINT('Ctrl Pts',(-15.4640980298328,-1.913286145342,0.767061604017206));
#50545=CARTESIAN_POINT('Ctrl Pts',(-15.5011468114586,-1.52143930925716,
1.39078028694765));
#50546=CARTESIAN_POINT('Ctrl Pts',(-15.5381955930844,-0.957246999683104,
1.70714053127933));
#50547=CARTESIAN_POINT('Ctrl Pts',(-15.5752443747102,-0.393054690109075,
2.023500775611));
#50548=CARTESIAN_POINT('Ctrl Pts',(-15.6122931563361,0.34348309295417,2.03250258134392));
#50549=CARTESIAN_POINT('Ctrl Pts',(-15.6493419379619,0.915238696889824,
1.73002564710885));
#50550=CARTESIAN_POINT('Ctrl Pts',(-15.6863907195877,1.4869943008255,1.42754871287377));
#50551=CARTESIAN_POINT('Ctrl Pts',(-15.7234395012135,1.89396772563359,0.81359303867069));
#50552=CARTESIAN_POINT('Ctrl Pts',(-15.7604882828393,1.94987932818113,0.169178064390397));
#50553=CARTESIAN_POINT('Ctrl Pts',(-15.7975370644651,2.00579093072867,-0.475236909889895));
#50554=CARTESIAN_POINT('Ctrl Pts',(-15.8345858460909,1.71064071101566,-1.15011118424738));
#50555=CARTESIAN_POINT('Ctrl Pts',(-15.8716346277167,1.19952465872418,-1.54654169198623));
#50556=CARTESIAN_POINT('Ctrl Pts',(-15.9086834093425,0.688408606432718,
-1.94297219972505));
#50557=CARTESIAN_POINT('Ctrl Pts',(-15.9457321909683,-0.0386732784372092,
-2.06095894084525));
#50558=CARTESIAN_POINT('Ctrl Pts',(-15.9827809725941,-0.648921491579182,
-1.84649709171329));
#50559=CARTESIAN_POINT('Ctrl Pts',(-16.0198297542199,-1.25916970472118,
-1.63203524258132));
#50560=CARTESIAN_POINT('Ctrl Pts',(-16.0568785358457,-1.75258424613523,
-1.08512480319718));
#50561=CARTESIAN_POINT('Ctrl Pts',(-16.0939273174715,-1.90331969425709,
-0.456097306933615));
#50562=CARTESIAN_POINT('Ctrl Pts',(-16.1026616476063,-1.93885590109382,
-0.307802718688236));
#50563=CARTESIAN_POINT('Ctrl Pts',(-16.111395977741,-1.95534631955948,-0.154944140057699));
#50564=CARTESIAN_POINT('Ctrl Pts',(-16.1201303078758,-1.95394212134825,
-0.00178662227266063));
#50565=CARTESIAN_POINT('Ctrl Pts',(-16.2218696921242,-1.95423044051614,
-0.00177357873807178));
#50566=CARTESIAN_POINT('Ctrl Pts',(-16.2136772180267,-1.95555620523854,
-0.14537534009457));
#50567=CARTESIAN_POINT('Ctrl Pts',(-16.2054847439292,-1.9410703771609,-0.288711992183037));
#50568=CARTESIAN_POINT('Ctrl Pts',(-16.1972922698318,-1.90977176526088,
-0.428278272262475));
#50569=CARTESIAN_POINT('Ctrl Pts',(-16.160243488206,-1.7682302207068,-1.05943811133816));
#50570=CARTESIAN_POINT('Ctrl Pts',(-16.1231947065801,-1.28284793363885,
-1.61348951169046));
#50571=CARTESIAN_POINT('Ctrl Pts',(-16.0861459249543,-0.675793806758042,
-1.83683238337832));
#50572=CARTESIAN_POINT('Ctrl Pts',(-16.0490971433285,-0.0687396798772465,
-2.06017525506617));
#50573=CARTESIAN_POINT('Ctrl Pts',(-16.0120483617027,0.659986286816407,
-1.9528095980896));
#50574=CARTESIAN_POINT('Ctrl Pts',(-15.9749995800769,1.17683206082491,-1.5638787595253));
#50575=CARTESIAN_POINT('Ctrl Pts',(-15.9379507984511,1.69367783483344,-1.17494792096097));
#50576=CARTESIAN_POINT('Ctrl Pts',(-15.9009020168253,1.9986434161568,-0.504451900808881));
#50577=CARTESIAN_POINT('Ctrl Pts',(-15.8638532351995,1.95214013341295,0.140710246244767));
#50578=CARTESIAN_POINT('Ctrl Pts',(-15.8268044535737,1.9056368506691,0.785872393298378));
#50579=CARTESIAN_POINT('Ctrl Pts',(-15.7897556719479,1.50766470385809,1.40570066725355));
#50580=CARTESIAN_POINT('Ctrl Pts',(-15.7527068903221,0.940383276298581,
1.71648762522126));
#50581=CARTESIAN_POINT('Ctrl Pts',(-15.7156581086963,0.373101848739073,
2.02727458318898));
#50582=CARTESIAN_POINT('Ctrl Pts',(-15.6786093270705,-0.363488859568931,
2.02902022516925));
#50583=CARTESIAN_POINT('Ctrl Pts',(-15.6415605454446,-0.932236971095907,
1.7209255369137));
#50584=CARTESIAN_POINT('Ctrl Pts',(-15.6045117638188,-1.5009850826229,1.41283084865815));
#50585=CARTESIAN_POINT('Ctrl Pts',(-15.567462982193,-1.90189059736886,0.794895830166782));
#50586=CARTESIAN_POINT('Ctrl Pts',(-15.5304142005672,-1.95145127252239,
0.149961344521046));
#50587=CARTESIAN_POINT('Ctrl Pts',(-15.5275660310862,-1.95526130881067,
0.100381233147203));
#50588=CARTESIAN_POINT('Ctrl Pts',(-15.5247178616052,-1.95699491471456,
0.0506415562763195));
#50589=CARTESIAN_POINT('Ctrl Pts',(-15.5218696921242,-1.95671484857984,
0.000882047759029596));
#50590=CARTESIAN_POINT('Origin',(-14.8,0.,0.));
#50591=CARTESIAN_POINT('',(-14.7201303078758,-1.95178645645483,0.00133170247388875));
#50592=CARTESIAN_POINT('',(-14.8218696921242,-1.95159637362084,0.00122105347580572));
#50593=CARTESIAN_POINT('',(-14.8,-1.954,-2.39295984553393E-16));
#50594=CARTESIAN_POINT('Ctrl Pts',(-14.7201303078758,-1.95178645645483,
0.00133170247388875));
#50595=CARTESIAN_POINT('Ctrl Pts',(-14.733477264898,-1.95325840706067,0.236027446913741));
#50596=CARTESIAN_POINT('Ctrl Pts',(-14.7468242219202,-1.91411010663923,
0.470248610705033));
#50597=CARTESIAN_POINT('Ctrl Pts',(-14.7601711789425,-1.83215096261091,
0.688384675993667));
#50598=CARTESIAN_POINT('Ctrl Pts',(-14.7972199605683,-1.60464693871359,
1.29389164167338));
#50599=CARTESIAN_POINT('Ctrl Pts',(-14.8342687421941,-1.04727724246687,
1.77545987161808));
#50600=CARTESIAN_POINT('Ctrl Pts',(-14.8713175238199,-0.415160812309883,
1.91266623117082));
#50601=CARTESIAN_POINT('Ctrl Pts',(-14.9083663054457,0.216955617847083,
2.04987259072355));
#50602=CARTESIAN_POINT('Ctrl Pts',(-14.9454150870715,0.923818781914313,
1.84271707988433));
#50603=CARTESIAN_POINT('Ctrl Pts',(-14.9824638686973,1.38188367690205,1.38601880054011));
#50604=CARTESIAN_POINT('Ctrl Pts',(-15.0195126503231,1.83994857188978,0.929320521195901));
#50605=CARTESIAN_POINT('Ctrl Pts',(-15.0565614319489,2.04921519779803,0.223079473346703));
#50606=CARTESIAN_POINT('Ctrl Pts',(-15.0936102135747,1.91389815435844,-0.409444094697087));
#50607=CARTESIAN_POINT('Ctrl Pts',(-15.1306589952005,1.77858111091886,-1.04196766274089));
#50608=CARTESIAN_POINT('Ctrl Pts',(-15.1677077768263,1.29868039813141,-1.60077375097929));
#50609=CARTESIAN_POINT('Ctrl Pts',(-15.2047565584522,0.693855895654001,
-1.83008595645264));
#50610=CARTESIAN_POINT('Ctrl Pts',(-15.241805340078,0.0890313931765885,
-2.05939816192598));
#50611=CARTESIAN_POINT('Ctrl Pts',(-15.2788541217038,-0.640716898990796,
-1.95921648463428));
#50612=CARTESIAN_POINT('Ctrl Pts',(-15.3159029033296,-1.16136901011926,
-1.57539602458353));
#50613=CARTESIAN_POINT('Ctrl Pts',(-15.3506453715116,-1.64961015088056,
-1.21546866568636));
#50614=CARTESIAN_POINT('Ctrl Pts',(-15.3853878396937,-1.95397760791726,
-0.606116819101585));
#50615=CARTESIAN_POINT('Ctrl Pts',(-15.4201303078757,-1.95687456006756,
0.000726948241557314));
#50616=CARTESIAN_POINT('Ctrl Pts',(-15.5218696921242,-1.95671484857984,
0.000882047759029596));
#50617=CARTESIAN_POINT('Ctrl Pts',(-15.4876690799794,-1.95335183478724,
-0.596626514374143));
#50618=CARTESIAN_POINT('Ctrl Pts',(-15.4534684678346,-1.65963680798056,
-1.19699460792317));
#50619=CARTESIAN_POINT('Ctrl Pts',(-15.4192678556898,-1.18423125427178,
-1.5582832894842));
#50620=CARTESIAN_POINT('Ctrl Pts',(-15.382219074064,-0.66923472530654,-1.9496594850436));
#50621=CARTESIAN_POINT('Ctrl Pts',(-15.3451702924382,0.0589741681850112,
-2.06047792336231));
#50622=CARTESIAN_POINT('Ctrl Pts',(-15.3081215108124,0.667080068155104,
-1.84001485226342));
#50623=CARTESIAN_POINT('Ctrl Pts',(-15.2710727291866,1.27518596812519,-1.61955178116453));
#50624=CARTESIAN_POINT('Ctrl Pts',(-15.2340239475608,1.76318887457379,-1.06780720064803));
#50625=CARTESIAN_POINT('Ctrl Pts',(-15.196975165935,1.90772037639653,-0.437325324399675));
#50626=CARTESIAN_POINT('Ctrl Pts',(-15.1599263843091,2.05225187821928,0.193156551848714));
#50627=CARTESIAN_POINT('Ctrl Pts',(-15.1228776026833,1.85331197541611,0.902375723828967));
#50628=CARTESIAN_POINT('Ctrl Pts',(-15.0858288210575,1.4019593264647,1.36570879795747));
#50629=CARTESIAN_POINT('Ctrl Pts',(-15.0487800394317,0.950606677513312,
1.82904187208595));
#50630=CARTESIAN_POINT('Ctrl Pts',(-15.0117312578059,0.246841282413703,
2.04648884836271));
#50631=CARTESIAN_POINT('Ctrl Pts',(-14.9746824761801,-0.387209764883699,
1.91852002122952));
#50632=CARTESIAN_POINT('Ctrl Pts',(-14.9376336945543,-1.02126081218112,
1.79055119409632));
#50633=CARTESIAN_POINT('Ctrl Pts',(-14.9005849129285,-1.58559751167634,
1.31716656355314));
#50634=CARTESIAN_POINT('Ctrl Pts',(-14.8635361313027,-1.82191199218985,
0.715043471821536));
#50635=CARTESIAN_POINT('Ctrl Pts',(-14.8496473182432,-1.91050134652424,
0.489320122958544));
#50636=CARTESIAN_POINT('Ctrl Pts',(-14.8357585051837,-1.9529923205933,0.245504601690091));
#50637=CARTESIAN_POINT('Ctrl Pts',(-14.8218696921242,-1.95159637362084,
0.00122105347580572));
#50638=CARTESIAN_POINT('Origin',(-14.8,0.,0.));
#50639=CARTESIAN_POINT('',(-14.0201303078758,-1.95205107141426,-0.00145700329680948));
#50640=CARTESIAN_POINT('',(-14.1218696921242,-1.9522775756875,-0.00154333085131984));
#50641=CARTESIAN_POINT('',(-14.8,-1.954,-2.39295984553393E-16));
#50642=CARTESIAN_POINT('Ctrl Pts',(-14.0201303078758,-1.95205107141426,
-0.00145700329680948));
#50643=CARTESIAN_POINT('Ctrl Pts',(-14.0445179084765,-1.94908269934858,
0.427233645472459));
#50644=CARTESIAN_POINT('Ctrl Pts',(-14.0689055090772,-1.81006537290534,
0.857674730656689));
#50645=CARTESIAN_POINT('Ctrl Pts',(-14.0932931096779,-1.55011885390173,
1.19489838510117));
#50646=CARTESIAN_POINT('Ctrl Pts',(-14.1303418913037,-1.15521728180249,
1.70719665245101));
#50647=CARTESIAN_POINT('Ctrl Pts',(-14.1673906729295,-0.481227900675196,
2.00436201468867));
#50648=CARTESIAN_POINT('Ctrl Pts',(-14.2044394545554,0.163351255607294,
1.95037611224874));
#50649=CARTESIAN_POINT('Ctrl Pts',(-14.2414882361812,0.807930411889783,
1.89639020980881));
#50650=CARTESIAN_POINT('Ctrl Pts',(-14.278537017807,1.42309934332747,1.49125304269128));
#50651=CARTESIAN_POINT('Ctrl Pts',(-14.3155857994328,1.72728327862235,0.920403763209719));
#50652=CARTESIAN_POINT('Ctrl Pts',(-14.3526345810586,2.03146721391722,0.349554483728171));
#50653=CARTESIAN_POINT('Ctrl Pts',(-14.3896833626844,2.02466615306931,-0.387006908117411));
#50654=CARTESIAN_POINT('Ctrl Pts',(-14.4267321443102,1.70999307375835,-0.952141953511904));
#50655=CARTESIAN_POINT('Ctrl Pts',(-14.463780925936,1.39531999444738,-1.51727699890641));
#50656=CARTESIAN_POINT('Ctrl Pts',(-14.5008297075618,0.772774896673343,
-1.91098569784982));
#50657=CARTESIAN_POINT('Ctrl Pts',(-14.5378784891876,0.127308766369077,
-1.95305992994188));
#50658=CARTESIAN_POINT('Ctrl Pts',(-14.5749272708134,-0.518157363935189,
-1.99513416203393));
#50659=CARTESIAN_POINT('Ctrl Pts',(-14.6119760524392,-1.18654452676969,
-1.68557392727462));
#50660=CARTESIAN_POINT('Ctrl Pts',(-14.649024834065,-1.57191893241295,-1.16607095918761));
#50661=CARTESIAN_POINT('Ctrl Pts',(-14.6727266586686,-1.8184608203896,-0.833720806489077));
#50662=CARTESIAN_POINT('Ctrl Pts',(-14.6964284832722,-1.94917253366878,
-0.415446246286262));
#50663=CARTESIAN_POINT('Ctrl Pts',(-14.7201303078758,-1.95178645645483,
0.00133170247388875));
#50664=CARTESIAN_POINT('Ctrl Pts',(-14.8218696921242,-1.95159637362084,
0.00122105347580572));
#50665=CARTESIAN_POINT('Ctrl Pts',(-14.7987097235579,-1.94926859457566,
-0.406128319985333));
#50666=CARTESIAN_POINT('Ctrl Pts',(-14.7755497549916,-1.82490683437804,
-0.814779110591518));
#50667=CARTESIAN_POINT('Ctrl Pts',(-14.7523897864253,-1.58876519036178,
-1.14301165513501));
#50668=CARTESIAN_POINT('Ctrl Pts',(-14.7153410047994,-1.2110116464884,-1.66808213743989));
#50669=CARTESIAN_POINT('Ctrl Pts',(-14.6782922231736,-0.547212297209818,
-1.98736154912963));
#50670=CARTESIAN_POINT('Ctrl Pts',(-14.6412434415478,0.09879899914816,-1.95470950057729));
#50671=CARTESIAN_POINT('Ctrl Pts',(-14.604194659922,0.744810295506157,-1.92205745202494));
#50672=CARTESIAN_POINT('Ctrl Pts',(-14.5671458782962,1.37303353894355,-1.5374739432305));
#50673=CARTESIAN_POINT('Ctrl Pts',(-14.5300970966704,1.69591874594352,-0.976990317780662));
#50674=CARTESIAN_POINT('Ctrl Pts',(-14.4930483150446,2.01880395294348,-0.416506692330825));
#50675=CARTESIAN_POINT('Ctrl Pts',(-14.4559995334188,2.03635112350602,0.319877049774405));
#50676=CARTESIAN_POINT('Ctrl Pts',(-14.418950751793,1.74052857676173,0.89510376345739));
#50677=CARTESIAN_POINT('Ctrl Pts',(-14.3819019701672,1.44470603001745,1.47033047714036));
#50678=CARTESIAN_POINT('Ctrl Pts',(-14.3448531885414,0.835513765966365,
1.8844001624011));
#50679=CARTESIAN_POINT('Ctrl Pts',(-14.3078044069156,0.191790919130116,
1.94778507983274));
#50680=CARTESIAN_POINT('Ctrl Pts',(-14.2707556252898,-0.451931927706151,
2.01116999726438));
#50681=CARTESIAN_POINT('Ctrl Pts',(-14.2337068436639,-1.13018535732759,
1.7238701468669));
#50682=CARTESIAN_POINT('Ctrl Pts',(-14.1966580620381,-1.53251959802447,
1.21738825177127));
#50683=CARTESIAN_POINT('Ctrl Pts',(-14.1717286054001,-1.80324304876393,
0.876585723654715));
#50684=CARTESIAN_POINT('Ctrl Pts',(-14.1467991487622,-1.94903853347043,
0.436544113465563));
#50685=CARTESIAN_POINT('Ctrl Pts',(-14.1218696921242,-1.9522775756875,-0.00154333085131984));
#50686=CARTESIAN_POINT('Origin',(-14.8,0.,0.));
#50687=CARTESIAN_POINT('',(-13.3201303078758,-1.95703609937262,-0.000519725096467805));
#50688=CARTESIAN_POINT('',(-13.4218696921242,-1.957128029801,-0.000349295805945385));
#50689=CARTESIAN_POINT('',(-14.8,-1.954,-2.39295984553393E-16));
#50690=CARTESIAN_POINT('Ctrl Pts',(-13.3201303078758,-1.95703609937262,
-0.000519725096467805));
#50691=CARTESIAN_POINT('Ctrl Pts',(-13.355558552055,-1.95484025103045,0.618166309907161));
#50692=CARTESIAN_POINT('Ctrl Pts',(-13.3909867962342,-1.63665153253831,
1.23879689579462));
#50693=CARTESIAN_POINT('Ctrl Pts',(-13.4264150404134,-1.13208054584297,
1.59657265718252));
#50694=CARTESIAN_POINT('Ctrl Pts',(-13.4634638220392,-0.604429776410676,
1.97071358236128));
#50695=CARTESIAN_POINT('Ctrl Pts',(-13.500512603665,0.127043995617411,2.05740302359373));
#50696=CARTESIAN_POINT('Ctrl Pts',(-13.5375613852908,0.727531013857885,
1.81696153944268));
#50697=CARTESIAN_POINT('Ctrl Pts',(-13.5746101669166,1.32801803209836,1.57652005529162));
#50698=CARTESIAN_POINT('Ctrl Pts',(-13.6116589485424,1.79751829655122,1.00894764575704));
#50699=CARTESIAN_POINT('Ctrl Pts',(-13.6487077301682,1.92113241481916,0.374033229366182));
#50700=CARTESIAN_POINT('Ctrl Pts',(-13.685756511794,2.04474653308709,-0.260881187024657));
#50701=CARTESIAN_POINT('Ctrl Pts',(-13.7228052934198,1.82247450517011,-0.963137610271772));
#50702=CARTESIAN_POINT('Ctrl Pts',(-13.7598540750457,1.35605455650233,-1.41129963215763));
#50703=CARTESIAN_POINT('Ctrl Pts',(-13.7969028566715,0.889634607834529,
-1.8594616540435));
#50704=CARTESIAN_POINT('Ctrl Pts',(-13.8339516382973,0.179066738415911,
-2.0535292745681));
#50705=CARTESIAN_POINT('Ctrl Pts',(-13.8710004199231,-0.450408333150168,
-1.90467397351039));
#50706=CARTESIAN_POINT('Ctrl Pts',(-13.9080492015489,-1.07988340471625,
-1.75581867245269));
#50707=CARTESIAN_POINT('Ctrl Pts',(-13.9450979831747,-1.62826567842979,
-1.26404044981269));
#50708=CARTESIAN_POINT('Ctrl Pts',(-13.9821467648005,-1.84454993375096,
-0.65443575226167));
#50709=CARTESIAN_POINT('Ctrl Pts',(-13.9948079458256,-1.91846367637156,
-0.446107297431768));
#50710=CARTESIAN_POINT('Ctrl Pts',(-14.0074691268507,-1.95359214536773,
-0.224018049653602));
#50711=CARTESIAN_POINT('Ctrl Pts',(-14.0201303078758,-1.95205107141426,
-0.00145700329680948));
#50712=CARTESIAN_POINT('Ctrl Pts',(-14.1218696921242,-1.9522775756875,-0.00154333085131984));
#50713=CARTESIAN_POINT('Ctrl Pts',(-14.1097503671363,-1.95385221912429,
-0.214517251135975));
#50714=CARTESIAN_POINT('Ctrl Pts',(-14.0976310421485,-1.92173553791281,
-0.427029330232189));
#50715=CARTESIAN_POINT('Ctrl Pts',(-14.0855117171607,-1.85390212817894,
-0.627453084312592));
#50716=CARTESIAN_POINT('Ctrl Pts',(-14.0484629355349,-1.64653536586419,
-1.24014858550701));
#50717=CARTESIAN_POINT('Ctrl Pts',(-14.0114141539091,-1.10538678946238,
-1.73987564810208));
#50718=CARTESIAN_POINT('Ctrl Pts',(-13.9743653722833,-0.478150615718903,
-1.89789948695062));
#50719=CARTESIAN_POINT('Ctrl Pts',(-13.9373165906575,0.149085558024587,
-2.05592332579916));
#50720=CARTESIAN_POINT('Ctrl Pts',(-13.9002678090317,0.862409329109737,
-1.87224394090116));
#50721=CARTESIAN_POINT('Ctrl Pts',(-13.8632190274059,1.33531854919931,-1.43093495521077));
#50722=CARTESIAN_POINT('Ctrl Pts',(-13.8261702457801,1.80822776928888,-0.989625969520384));
#50723=CARTESIAN_POINT('Ctrl Pts',(-13.7891214641543,2.04072243838287,-0.29068738303762));
#50724=CARTESIAN_POINT('Ctrl Pts',(-13.7520726825284,1.92638522957703,0.345963034365286));
#50725=CARTESIAN_POINT('Ctrl Pts',(-13.7150239009026,1.8120480207712,0.982613451768174));
#50726=CARTESIAN_POINT('Ctrl Pts',(-13.6779751192768,1.35087893406555,1.55697570009121));
#50727=CARTESIAN_POINT('Ctrl Pts',(-13.640926337651,0.753964019946039,1.80615301968205));
#50728=CARTESIAN_POINT('Ctrl Pts',(-13.6038775560252,0.157049105826529,
2.0553303392729));
#50729=CARTESIAN_POINT('Ctrl Pts',(-13.5668287743994,-0.575611635706843,
1.97932273013156));
#50730=CARTESIAN_POINT('Ctrl Pts',(-13.5297799927736,-1.10866514926791,
1.61292035162266));
#50731=CARTESIAN_POINT('Ctrl Pts',(-13.4938098925571,-1.62619872155089,
1.25718583901078));
#50732=CARTESIAN_POINT('Ctrl Pts',(-13.4578397923407,-1.95557905520156,
0.627720175010101));
#50733=CARTESIAN_POINT('Ctrl Pts',(-13.4218696921242,-1.957128029801,-0.000349295805945385));
#50734=CARTESIAN_POINT('Origin',(-14.8,0.,0.));
#50735=CARTESIAN_POINT('',(-12.6201303078758,-1.95358117384718,0.00178179146160605));
#50736=CARTESIAN_POINT('',(-12.7218696921242,-1.95330164162301,0.00176139094907822));
#50737=CARTESIAN_POINT('',(-14.8,-1.954,-2.39295984553393E-16));
#50738=CARTESIAN_POINT('Ctrl Pts',(-12.6201303078758,-1.95358117384718,
0.00178179146160605));
#50739=CARTESIAN_POINT('Ctrl Pts',(-12.6295504140077,-1.95506722451589,
0.167042362152062));
#50740=CARTESIAN_POINT('Ctrl Pts',(-12.6389705201395,-1.93584624707066,
0.331962304665006));
#50741=CARTESIAN_POINT('Ctrl Pts',(-12.6483906262714,-1.89457311803675,
0.491165259715588));
#50742=CARTESIAN_POINT('Ctrl Pts',(-12.6854394078972,-1.73224807379813,
1.11730210289686));
#50743=CARTESIAN_POINT('Ctrl Pts',(-12.722488189523,-1.22881869473678,1.65500815520059));
#50744=CARTESIAN_POINT('Ctrl Pts',(-12.7595369711488,-0.614714388174372,
1.85816491004173));
#50745=CARTESIAN_POINT('Ctrl Pts',(-12.7965857527747,-0.00061008161194781,
2.06132166488287));
#50746=CARTESIAN_POINT('Ctrl Pts',(-12.8336345344005,0.724169152451543,
1.92992912226141));
#50747=CARTESIAN_POINT('Ctrl Pts',(-12.8706833160263,1.22787777771923,1.52412820160322));
#50748=CARTESIAN_POINT('Ctrl Pts',(-12.9077320976521,1.73158640298692,1.11832728094503));
#50749=CARTESIAN_POINT('Ctrl Pts',(-12.9447808792779,2.01422441945881,0.438117982250111));
#50750=CARTESIAN_POINT('Ctrl Pts',(-12.9818296609037,1.94642291596085,-0.205154683498651));
#50751=CARTESIAN_POINT('Ctrl Pts',(-13.0188784425295,1.8786214124629,-0.848427349247394));
#50752=CARTESIAN_POINT('Ctrl Pts',(-13.0559272241553,1.46038038899512,-1.45476338204999));
#50753=CARTESIAN_POINT('Ctrl Pts',(-13.0929760057811,0.883136887501676,
-1.74663099991751));
#50754=CARTESIAN_POINT('Ctrl Pts',(-13.1300247874069,0.305893386008212,
-2.03849861778504));
#50755=CARTESIAN_POINT('Ctrl Pts',(-13.1670735690327,-0.430352593510932,
-2.01589782071748));
#50756=CARTESIAN_POINT('Ctrl Pts',(-13.2041223506585,-0.988606962590199,
-1.68917343261643));
#50757=CARTESIAN_POINT('Ctrl Pts',(-13.2411711322843,-1.54686133166947,
-1.36244904451537));
#50758=CARTESIAN_POINT('Ctrl Pts',(-13.2782199139102,-1.92712409030886,
-0.731601065380813));
#50759=CARTESIAN_POINT('Ctrl Pts',(-13.315268695536,-1.9553415862103,-0.0853808712510157));
#50760=CARTESIAN_POINT('Ctrl Pts',(-13.3168892329826,-1.95657583756084,
-0.0571147859067663));
#50761=CARTESIAN_POINT('Ctrl Pts',(-13.3185097704292,-1.9571365405474,-0.028819289769768));
#50762=CARTESIAN_POINT('Ctrl Pts',(-13.3201303078758,-1.95703609937262,
-0.000519725096467805));
#50763=CARTESIAN_POINT('Ctrl Pts',(-13.4218696921242,-1.957128029801,-0.000349295805945385));
#50764=CARTESIAN_POINT('Ctrl Pts',(-13.4207910107148,-1.95717448088382,
-0.0191840184745534));
#50765=CARTESIAN_POINT('Ctrl Pts',(-13.4197123293055,-1.95692611424454,
-0.0380174855509708));
#50766=CARTESIAN_POINT('Ctrl Pts',(-13.4186336478962,-1.95637916299247,
-0.0568422773001921));
#50767=CARTESIAN_POINT('Ctrl Pts',(-13.3815848662704,-1.93759337756717,
-0.703405379837554));
#50768=CARTESIAN_POINT('Ctrl Pts',(-13.3445360846446,-1.56657552112786,
-1.33973443703577));
#50769=CARTESIAN_POINT('Ctrl Pts',(-13.3074873030187,-1.01314767462749,
-1.67456927694159));
#50770=CARTESIAN_POINT('Ctrl Pts',(-13.2704385213929,-0.459719828127115,
-2.00940411684742));
#50771=CARTESIAN_POINT('Ctrl Pts',(-13.2333897397671,0.276118008434306,
-2.04274473946083));
#50772=CARTESIAN_POINT('Ctrl Pts',(-13.1963409581413,0.857558561552295,
-1.7593304940767));
#50773=CARTESIAN_POINT('Ctrl Pts',(-13.1592921765155,1.43899911467027,-1.47591624869258));
#50774=CARTESIAN_POINT('Ctrl Pts',(-13.1222433948897,1.86604238434483,-0.875747135310894));
#50775=CARTESIAN_POINT('Ctrl Pts',(-13.0851946132639,1.94322236953466,-0.233532217092017));
#50776=CARTESIAN_POINT('Ctrl Pts',(-13.0481458316381,2.02040235472448,0.40868270112686));
#50777=CARTESIAN_POINT('Ctrl Pts',(-13.0110970500123,1.74771905542961,1.09294342418297));
#50778=CARTESIAN_POINT('Ctrl Pts',(-12.9740482683865,1.2499849153739,1.50605052545307));
#50779=CARTESIAN_POINT('Ctrl Pts',(-12.9369994867607,0.75225077531818,1.91915762672319));
#50780=CARTESIAN_POINT('Ctrl Pts',(-12.8999507051349,0.029465794501616,
2.06111110620728));
#50781=CARTESIAN_POINT('Ctrl Pts',(-12.862901923509,-0.587537299234008,
1.86693609850166));
#50782=CARTESIAN_POINT('Ctrl Pts',(-12.8258531418832,-1.20454039296963,
1.67276109079604));
#50783=CARTESIAN_POINT('Ctrl Pts',(-12.7888043602574,-1.7157615996243,1.14245759590073));
#50784=CARTESIAN_POINT('Ctrl Pts',(-12.7517555786316,-1.88720504100882,
0.518755826059528));
#50785=CARTESIAN_POINT('Ctrl Pts',(-12.7417936164625,-1.93330407591021,
0.351050083432241));
#50786=CARTESIAN_POINT('Ctrl Pts',(-12.7318316542933,-1.95483697372639,
0.176591589270381));
#50787=CARTESIAN_POINT('Ctrl Pts',(-12.7218696921242,-1.95330164162301,
0.00176139094907822));
#50788=CARTESIAN_POINT('Origin',(-14.8,0.,0.));
#50789=CARTESIAN_POINT('',(-11.9201303078758,-1.95093708226589,-0.000550973528005427));
#50790=CARTESIAN_POINT('',(-12.0218696921242,-1.95102823519099,-0.000697989405693117));
#50791=CARTESIAN_POINT('',(-14.8,-1.954,-2.39295984553393E-16));
#50792=CARTESIAN_POINT('Ctrl Pts',(-11.9201303078758,-1.95093708226589,
-0.000550973528005427));
#50793=CARTESIAN_POINT('Ctrl Pts',(-11.9405910575861,-1.95002744544509,
0.359627574766655));
#50794=CARTESIAN_POINT('Ctrl Pts',(-11.9610518072965,-1.85458725485174,
0.720254388310455));
#50795=CARTESIAN_POINT('Ctrl Pts',(-11.9815125570069,-1.66757630645233,
1.02461694017705));
#50796=CARTESIAN_POINT('Ctrl Pts',(-12.0185613386327,-1.3289509927683,1.57573368217324));
#50797=CARTESIAN_POINT('Ctrl Pts',(-12.0556101202585,-0.690090496095906,
1.9423754749052));
#50798=CARTESIAN_POINT('Ctrl Pts',(-12.0926589018843,-0.0434136774160742,
1.95672324679608));
#50799=CARTESIAN_POINT('Ctrl Pts',(-12.1297076835101,0.603263141263758,
1.97107101868696));
#50800=CARTESIAN_POINT('Ctrl Pts',(-12.1667564651359,1.25775628195103,1.63312476973678));
#50801=CARTESIAN_POINT('Ctrl Pts',(-12.2038052467617,1.62049151879134,1.09756906364216));
#50802=CARTESIAN_POINT('Ctrl Pts',(-12.2408540283875,1.98322675563165,0.562013357547537));
#50803=CARTESIAN_POINT('Ctrl Pts',(-12.2779028100133,2.05420408862499,-0.171151805691514));
#50804=CARTESIAN_POINT('Ctrl Pts',(-12.3149515916392,1.80093581352688,-0.766342487074322));
#50805=CARTESIAN_POINT('Ctrl Pts',(-12.352000373265,1.54766753842878,-1.36153316845711));
#50806=CARTESIAN_POINT('Ctrl Pts',(-12.3890491548908,0.970153655239247,
-1.81874936798367));
#50807=CARTESIAN_POINT('Ctrl Pts',(-12.4260979365166,0.332733488118346,
-1.92871434842581));
#50808=CARTESIAN_POINT('Ctrl Pts',(-12.4631467181424,-0.304686679002573,
-2.03867932886795));
#50809=CARTESIAN_POINT('Ctrl Pts',(-12.5001954997682,-1.00201313005487,
-1.80139309022565));
#50810=CARTESIAN_POINT('Ctrl Pts',(-12.537244281394,-1.44006600087307,-1.32546615387509));
#50811=CARTESIAN_POINT('Ctrl Pts',(-12.5648729568879,-1.76673856838838,
-0.970549465492388));
#50812=CARTESIAN_POINT('Ctrl Pts',(-12.5925016323818,-1.94922266544841,
-0.482918764521644));
#50813=CARTESIAN_POINT('Ctrl Pts',(-12.6201303078758,-1.95358117384718,
0.00178179146160605));
#50814=CARTESIAN_POINT('Ctrl Pts',(-12.7218696921242,-1.95330164162301,
0.00176139094907822));
#50815=CARTESIAN_POINT('Ctrl Pts',(-12.6947828726675,-1.94912703597966,
-0.473606206025261));
#50816=CARTESIAN_POINT('Ctrl Pts',(-12.6676960532109,-1.77440682962847,
-0.951721846927492));
#50817=CARTESIAN_POINT('Ctrl Pts',(-12.6406092337542,-1.45925195975997,
-1.30431368612634));
#50818=CARTESIAN_POINT('Ctrl Pts',(-12.6035604521284,-1.02818976101222,
-1.786581383684));
#50819=CARTESIAN_POINT('Ctrl Pts',(-12.5665116705026,-0.334399687402313,
-2.03401673401225));
#50820=CARTESIAN_POINT('Ctrl Pts',(-12.5294628888768,0.30455706556366,-1.93336377014132));
#50821=CARTESIAN_POINT('Ctrl Pts',(-12.492414107251,0.943513818529596,-1.83271080627039));
#50822=CARTESIAN_POINT('Ctrl Pts',(-12.4553653256252,1.52763725085163,-1.38396952820033));
#50823=CARTESIAN_POINT('Ctrl Pts',(-12.4183165439994,1.78956271932274,-0.792537536959608));
#50824=CARTESIAN_POINT('Ctrl Pts',(-12.3812677623736,2.05148818779385,-0.20110554571887));
#50825=CARTESIAN_POINT('Ctrl Pts',(-12.3442189807477,1.99121569241405,0.533017158692502));
#50826=CARTESIAN_POINT('Ctrl Pts',(-12.3071701991219,1.63633312528064,1.07380835207642));
#50827=CARTESIAN_POINT('Ctrl Pts',(-12.2701214174961,1.28145055814724,1.61459954546034));
#50828=CARTESIAN_POINT('Ctrl Pts',(-12.2330726358703,0.631957919260208,
1.96205922781676));
#50829=CARTESIAN_POINT('Ctrl Pts',(-12.1960238542445,-0.0148593923487363,
1.95714835215392));
#50830=CARTESIAN_POINT('Ctrl Pts',(-12.1589750726187,-0.661676703957681,
1.95223747649109));
#50831=CARTESIAN_POINT('Ctrl Pts',(-12.1219262909929,-1.30581868828856,
1.59495604280899));
#50832=CARTESIAN_POINT('Ctrl Pts',(-12.0848775093671,-1.65244904485148,
1.04883870449618));
#50833=CARTESIAN_POINT('Ctrl Pts',(-12.0638749036195,-1.84895053287836,
0.739249923294692));
#50834=CARTESIAN_POINT('Ctrl Pts',(-12.0428722978718,-1.94984221352703,
0.368975902315217));
#50835=CARTESIAN_POINT('Ctrl Pts',(-12.0218696921242,-1.95102823519099,
-0.000697989405693117));
#50836=CARTESIAN_POINT('Origin',(-14.8,0.,0.));
#50837=CARTESIAN_POINT('',(-11.2201303078758,-1.95560116054388,-0.00149635199143683));
#50838=CARTESIAN_POINT('',(-11.3218696921242,-1.95585802078492,-0.00139750151859497));
#50839=CARTESIAN_POINT('',(-14.8,-1.954,-2.39295984553393E-16));
#50840=CARTESIAN_POINT('Ctrl Pts',(-11.2201303078758,-1.95560116054388,
-0.00149635199143683));
#50841=CARTESIAN_POINT('Ctrl Pts',(-11.2516317011646,-1.95092725946121,
0.549677370997484));
#50842=CARTESIAN_POINT('Ctrl Pts',(-11.2831330944535,-1.70683034372718,
1.10447412907545));
#50843=CARTESIAN_POINT('Ctrl Pts',(-11.3146344877423,-1.29426767174851,
1.4681695425957));
#50844=CARTESIAN_POINT('Ctrl Pts',(-11.3516832693681,-0.809052805188828,
1.89591163737426));
#50845=CARTESIAN_POINT('Ctrl Pts',(-11.388732050994,-0.0908143044123737,
2.05932031030366));
#50846=CARTESIAN_POINT('Ctrl Pts',(-11.4257808326198,0.531696114981536,
1.8836002371131));
#50847=CARTESIAN_POINT('Ctrl Pts',(-11.4628296142456,1.15420653437546,1.70788016392253));
#50848=CARTESIAN_POINT('Ctrl Pts',(-11.4998783958714,1.68098887238684,1.19303134461199));
#50849=CARTESIAN_POINT('Ctrl Pts',(-11.5369271774972,1.87092461868595,0.574710086159801));
#50850=CARTESIAN_POINT('Ctrl Pts',(-11.573975959123,2.06086036498506,-0.0436111722923718));
#50851=CARTESIAN_POINT('Ctrl Pts',(-11.6110247407488,1.91394951957191,-0.765404869886186));
#50852=CARTESIAN_POINT('Ctrl Pts',(-11.6480735223746,1.49743603054664,-1.26029200836937));
#50853=CARTESIAN_POINT('Ctrl Pts',(-11.6851223040004,1.08092254152136,-1.75517914685256));
#50854=CARTESIAN_POINT('Ctrl Pts',(-11.7221710856262,0.394806408883924,
-2.02315972622511));
#50855=CARTESIAN_POINT('Ctrl Pts',(-11.759219867252,-0.246863683730499,
-1.94157382903509));
#50856=CARTESIAN_POINT('Ctrl Pts',(-11.7962686488778,-0.888533776344921,
-1.85998793184507));
#50857=CARTESIAN_POINT('Ctrl Pts',(-11.8333174305036,-1.48575782893633,
-1.42883555809249));
#50858=CARTESIAN_POINT('Ctrl Pts',(-11.8703662121295,-1.76517478988419,
-0.845463525585991));
#50859=CARTESIAN_POINT('Ctrl Pts',(-11.8869542440449,-1.8902795102696,-0.584267516725894));
#50860=CARTESIAN_POINT('Ctrl Pts',(-11.9035422759603,-1.95167454715981,
-0.292556561736662));
#50861=CARTESIAN_POINT('Ctrl Pts',(-11.9201303078758,-1.95093708226589,
-0.000550973528005427));
#50862=CARTESIAN_POINT('Ctrl Pts',(-12.0218696921242,-1.95102823519099,
-0.000697989405693117));
#50863=CARTESIAN_POINT('Ctrl Pts',(-12.005823516246,-1.95193436619415,-0.283132100458183));
#50864=CARTESIAN_POINT('Ctrl Pts',(-11.9897773403678,-1.89464136026534,
-0.565215910381814));
#50865=CARTESIAN_POINT('Ctrl Pts',(-11.9737311644897,-1.77732263479807,
-0.819618646514493));
#50866=CARTESIAN_POINT('Ctrl Pts',(-11.9366823828639,-1.50644713938678,
-1.40700541626888));
#50867=CARTESIAN_POINT('Ctrl Pts',(-11.8996336012381,-0.915577419769245,
-1.84682571283413));
#50868=CARTESIAN_POINT('Ctrl Pts',(-11.8625848196122,-0.275166025913142,
-1.93776524173156));
#50869=CARTESIAN_POINT('Ctrl Pts',(-11.8255360379864,0.365245367942961,
-2.02870477062899));
#50870=CARTESIAN_POINT('Ctrl Pts',(-11.7884872563606,1.05519843603763,-1.7707635318586));
#50871=CARTESIAN_POINT('Ctrl Pts',(-11.7514384747348,1.47888825483371,-1.2820062416364));
#50872=CARTESIAN_POINT('Ctrl Pts',(-11.714389693109,1.90257807362979,-0.793248951414214));
#50873=CARTESIAN_POINT('Ctrl Pts',(-11.6773409114832,2.06000464312729,-0.0736756097402326));
#50874=CARTESIAN_POINT('Ctrl Pts',(-11.6402921298574,1.87911076401531,0.547351085174407));
#50875=CARTESIAN_POINT('Ctrl Pts',(-11.6032433482316,1.69821688490332,1.16837778008906));
#50876=CARTESIAN_POINT('Ctrl Pts',(-11.5661945666058,1.17900255718184,1.69085782824438));
#50877=CARTESIAN_POINT('Ctrl Pts',(-11.52914578498,0.559122265841095,1.87564196096177));
#50878=CARTESIAN_POINT('Ctrl Pts',(-11.4920970033542,-0.060758025499648,
2.06042609367916));
#50879=CARTESIAN_POINT('Ctrl Pts',(-11.4550482217284,-0.781304280459649,
1.90751431095864));
#50880=CARTESIAN_POINT('Ctrl Pts',(-11.4179994401025,-1.27270847951518,
1.48689730649092));
#50881=CARTESIAN_POINT('Ctrl Pts',(-11.3859561907764,-1.69772076276046,
1.1231084056549));
#50882=CARTESIAN_POINT('Ctrl Pts',(-11.3539129414503,-1.95132545851315,
0.559065099150166));
#50883=CARTESIAN_POINT('Ctrl Pts',(-11.3218696921242,-1.95585802078492,
-0.00139750151859497));
#50884=CARTESIAN_POINT('Origin',(-14.8,0.,0.));
#50885=CARTESIAN_POINT('',(-10.5201303078758,-1.95562737994549,0.00148708654483385));
#50886=CARTESIAN_POINT('',(-10.6218696921242,-1.95536008754156,0.00157356082676479));
#50887=CARTESIAN_POINT('',(-14.8,-1.954,-2.39295984553393E-16));
#50888=CARTESIAN_POINT('Ctrl Pts',(-10.5201303078758,-1.95562737994549,
0.00148708654483385));
#50889=CARTESIAN_POINT('Ctrl Pts',(-10.5256235631173,-1.95643899330848,
0.0975981474980406));
#50890=CARTESIAN_POINT('Ctrl Pts',(-10.5311168183588,-1.94996615192806,
0.19359947904084));
#50891=CARTESIAN_POINT('Ctrl Pts',(-10.5366100736004,-1.935831083387,0.288459058675073));
#50892=CARTESIAN_POINT('Ctrl Pts',(-10.5736588552262,-1.84049834448853,
0.928231233179569));
#50893=CARTESIAN_POINT('Ctrl Pts',(-10.610707636852,-1.39663306929388,1.51606841800423));
#50894=CARTESIAN_POINT('Ctrl Pts',(-10.6477564184778,-0.807401017585439,
1.78290611327152));
#50895=CARTESIAN_POINT('Ctrl Pts',(-10.6848052001036,-0.218168965877002,
2.04974380853882));
#50896=CARTESIAN_POINT('Ctrl Pts',(-10.7218539817294,0.516429862345236,
1.99558201424877));
#50897=CARTESIAN_POINT('Ctrl Pts',(-10.7589027633552,1.06015531176482,1.64521163589242));
#50898=CARTESIAN_POINT('Ctrl Pts',(-10.795951544981,1.60388076118439,1.29484125753609));
#50899=CARTESIAN_POINT('Ctrl Pts',(-10.8330003266068,1.95673283180133,0.648262295113474));
#50900=CARTESIAN_POINT('Ctrl Pts',(-10.8700491082326,1.95720427575482,0.00142650133218715));
#50901=CARTESIAN_POINT('Ctrl Pts',(-10.9070978898584,1.9576757197083,-0.645409292449136));
#50902=CARTESIAN_POINT('Ctrl Pts',(-10.9441466714843,1.60576653699831,-1.29250191758911));
#50903=CARTESIAN_POINT('Ctrl Pts',(-10.9811954531101,1.06255239737241,-1.64366450797512));
#50904=CARTESIAN_POINT('Ctrl Pts',(-11.0182442347359,0.519338257746561,
-1.99482709836111));
#50905=CARTESIAN_POINT('Ctrl Pts',(-11.0552930163617,-0.215180838795228,
-2.05005965399313));
#50906=CARTESIAN_POINT('Ctrl Pts',(-11.0923417979875,-0.804801231675591,
-1.78408116111135));
#50907=CARTESIAN_POINT('Ctrl Pts',(-11.1293905796133,-1.394421624556,-1.51810266822956));
#50908=CARTESIAN_POINT('Ctrl Pts',(-11.1664393612391,-1.839143313775,-0.930913126833975));
#50909=CARTESIAN_POINT('Ctrl Pts',(-11.2034881428649,-1.93540854221306,
-0.291280597822286));
#50910=CARTESIAN_POINT('Ctrl Pts',(-11.2090355312019,-1.94982252783031,
-0.195507137112811));
#50911=CARTESIAN_POINT('Ctrl Pts',(-11.2145829195388,-1.95642423348279,
-0.0985579217609101));
#50912=CARTESIAN_POINT('Ctrl Pts',(-11.2201303078758,-1.95560116054388,
-0.00149635199143683));
#50913=CARTESIAN_POINT('Ctrl Pts',(-11.3218696921242,-1.95585802078492,
-0.00139750151859497));
#50914=CARTESIAN_POINT('Ctrl Pts',(-11.3168641598245,-1.95656606030428,
-0.088948349494719));
#50915=CARTESIAN_POINT('Ctrl Pts',(-11.3118586275248,-1.95119621341652,
-0.17641182068154));
#50916=CARTESIAN_POINT('Ctrl Pts',(-11.3068530952251,-1.93945243087164,
-0.26301091662872));
#50917=CARTESIAN_POINT('Ctrl Pts',(-11.2698043135993,-1.85253004002152,
-0.903979909065702));
#50918=CARTESIAN_POINT('Ctrl Pts',(-11.2327555319735,-1.41642311517025,
-1.49759566772477));
#50919=CARTESIAN_POINT('Ctrl Pts',(-11.1957067503477,-0.830746268420352,
-1.77214872721943));
#50920=CARTESIAN_POINT('Ctrl Pts',(-11.1586579687219,-0.245069421670441,
-2.0467017867141));
#50921=CARTESIAN_POINT('Ctrl Pts',(-11.1216091870961,0.490177346978098,
-2.00219214704436));
#50922=CARTESIAN_POINT('Ctrl Pts',(-11.0845604054703,1.03845730728765,-1.65899273501142));
#50923=CARTESIAN_POINT('Ctrl Pts',(-11.0475116238445,1.58673726759721,-1.31579332297848));
#50924=CARTESIAN_POINT('Ctrl Pts',(-11.0104628422187,1.94805041956778,-0.673904138582339));
#50925=CARTESIAN_POINT('Ctrl Pts',(-10.9734140605929,1.95701671402278,-0.027130332015815));
#50926=CARTESIAN_POINT('Ctrl Pts',(-10.936365278967,1.96598300847778,0.61964347455069));
#50927=CARTESIAN_POINT('Ctrl Pts',(-10.8993164973412,1.62260244541722,1.27130190328758));
#50928=CARTESIAN_POINT('Ctrl Pts',(-10.8622677157154,1.08404697968283,1.62956823107237));
#50929=CARTESIAN_POINT('Ctrl Pts',(-10.8252189340896,0.545491513948429,
1.98783455885716));
#50930=CARTESIAN_POINT('Ctrl Pts',(-10.7881701524638,-0.188238854459824,
2.05270878568984));
#50931=CARTESIAN_POINT('Ctrl Pts',(-10.751121370838,-0.781301481154613,
1.79449671758557));
#50932=CARTESIAN_POINT('Ctrl Pts',(-10.7140725892122,-1.37436410784942,
1.5362846494813));
#50933=CARTESIAN_POINT('Ctrl Pts',(-10.6770238075864,-1.82675899283075,
0.954986286440074));
#50934=CARTESIAN_POINT('Ctrl Pts',(-10.6399750259606,-1.93141620820529,
0.316673182574209));
#50935=CARTESIAN_POINT('Ctrl Pts',(-10.6339399146818,-1.9484644865345,0.212694308141715));
#50936=CARTESIAN_POINT('Ctrl Pts',(-10.627904803403,-1.95628546906628,0.107202534980138));
#50937=CARTESIAN_POINT('Ctrl Pts',(-10.6218696921242,-1.95536008754156,
0.00157356082676479));
#50938=CARTESIAN_POINT('Origin',(-14.8,0.,0.));
#50939=CARTESIAN_POINT('',(-9.82013030787577,-1.95094521463585,0.000565864204244704));
#50940=CARTESIAN_POINT('',(-9.92186969212419,-1.95087369540874,0.000415097647679855));
#50941=CARTESIAN_POINT('',(-14.8,-1.954,-2.39295984553393E-16));
#50942=CARTESIAN_POINT('Ctrl Pts',(-9.82013030787577,-1.95094521463585,
0.000565864204244704));
#50943=CARTESIAN_POINT('Ctrl Pts',(-9.8366642066958,-1.95170031682729,0.291615497447128));
#50944=CARTESIAN_POINT('Ctrl Pts',(-9.85319810551582,-1.89072216247003,
0.582364427271289));
#50945=CARTESIAN_POINT('Ctrl Pts',(-9.86973200433584,-1.76640533997838,
0.842889546046716));
#50946=CARTESIAN_POINT('Ctrl Pts',(-9.90678078596165,-1.48783905267716,
1.42666826264686));
#50947=CARTESIAN_POINT('Ctrl Pts',(-9.94382956758744,-0.891244121992129,
1.85869074709312));
#50948=CARTESIAN_POINT('Ctrl Pts',(-9.98087834921325,-0.249693638224819,
1.941211915008));
#50949=CARTESIAN_POINT('Ctrl Pts',(-10.0179271308391,0.391856845542454,
2.02373308292288));
#50950=CARTESIAN_POINT('Ctrl Pts',(-10.0549759124649,1.07836288239199,1.75675293430644));
#50951=CARTESIAN_POINT('Ctrl Pts',(-10.0920246940907,1.4955973219558,1.26247347001733));
#50952=CARTESIAN_POINT('Ctrl Pts',(-10.1290734757165,1.91283176151965,0.768194005728199));
#50953=CARTESIAN_POINT('Ctrl Pts',(-10.1661222573423,2.06079460379773,0.0466152257663319));
#50954=CARTESIAN_POINT('Ctrl Pts',(-10.2031710389681,1.87176038128685,-0.57198224359142));
#50955=CARTESIAN_POINT('Ctrl Pts',(-10.2402198205939,1.68272615877597,-1.19057971294919));
#50956=CARTESIAN_POINT('Ctrl Pts',(-10.2772686022197,1.15669487147614,-1.70619587170287));
#50957=CARTESIAN_POINT('Ctrl Pts',(-10.3143173838455,0.534441259215129,
-1.88282318670329));
#50958=CARTESIAN_POINT('Ctrl Pts',(-10.3513661654713,-0.0878123530458442,
-2.0594505017037));
#50959=CARTESIAN_POINT('Ctrl Pts',(-10.3884149470971,-0.806288290267959,
-1.89708897295088));
#50960=CARTESIAN_POINT('Ctrl Pts',(-10.4254637287229,-1.29212615757787,
-1.47005462648231));
#50961=CARTESIAN_POINT('Ctrl Pts',(-10.4570192551072,-1.70592841955826,
-1.10633703589916));
#50962=CARTESIAN_POINT('Ctrl Pts',(-10.4885747814915,-1.9509651376568,-0.550614533783712));
#50963=CARTESIAN_POINT('Ctrl Pts',(-10.5201303078758,-1.95562737994549,
0.00148708654483385));
#50964=CARTESIAN_POINT('Ctrl Pts',(-10.6218696921242,-1.95536008754156,
0.00157356082676479));
#50965=CARTESIAN_POINT('Ctrl Pts',(-10.5908560217772,-1.95060466941801,
-0.541240321494284));
#50966=CARTESIAN_POINT('Ctrl Pts',(-10.5598423514302,-1.71487513271243,
-1.08767740974916));
#50967=CARTESIAN_POINT('Ctrl Pts',(-10.5288286810832,-1.31343749192923,
-1.45104528829201));
#50968=CARTESIAN_POINT('Ctrl Pts',(-10.4917798994573,-0.833882014510803,
-1.885122810602));
#50969=CARTESIAN_POINT('Ctrl Pts',(-10.4547311178315,-0.117851513906124,
-2.05795001053151));
#50970=CARTESIAN_POINT('Ctrl Pts',(-10.4176823362057,0.506912938860662,
-1.89042052102051));
#50971=CARTESIAN_POINT('Ctrl Pts',(-10.3806335545799,1.13167739162745,-1.72289103150951));
#50972=CARTESIAN_POINT('Ctrl Pts',(-10.3435847729541,1.66517579655636,-1.21500485255799));
#50973=CARTESIAN_POINT('Ctrl Pts',(-10.3065359913283,1.86321556901111,-0.599231355383206));
#50974=CARTESIAN_POINT('Ctrl Pts',(-10.2694872097025,2.06125534146585,0.0165421417915641));
#50975=CARTESIAN_POINT('Ctrl Pts',(-10.2324384280767,1.92383648144648,0.740202957189575));
#50976=CARTESIAN_POINT('Ctrl Pts',(-10.1953896464509,1.51385827092997,1.24051747646566));
#50977=CARTESIAN_POINT('Ctrl Pts',(-10.1583408648251,1.10388006041343,1.74083199574176));
#50978=CARTESIAN_POINT('Ctrl Pts',(-10.1212920831993,0.421342499399717,
2.01780021889587));
#50979=CARTESIAN_POINT('Ctrl Pts',(-10.0842433015735,-0.221343710231941,
1.94464840930708));
#50980=CARTESIAN_POINT('Ctrl Pts',(-10.0471945199477,-0.864029919863581,
1.87149659971829));
#50981=CARTESIAN_POINT('Ctrl Pts',(-10.0101457383219,-1.46686477811318,
1.44822475738663));
#50982=CARTESIAN_POINT('Ctrl Pts',(-9.97309695669604,-1.75391905860483,
0.868572627787997));
#50983=CARTESIAN_POINT('Ctrl Pts',(-9.95602120183876,-1.88622215493648,
0.601411408628383));
#50984=CARTESIAN_POINT('Ctrl Pts',(-9.93894544698147,-1.95144458357273,
0.301030622392327));
#50985=CARTESIAN_POINT('Ctrl Pts',(-9.92186969212419,-1.95087369540874,
0.000415097647679855));
#50986=CARTESIAN_POINT('Origin',(-14.8,0.,0.));
#50987=CARTESIAN_POINT('',(-9.12013030787577,-1.9535529839402,-0.00178040573474675));
#50988=CARTESIAN_POINT('',(-9.22186969212419,-1.95383722770402,-0.00178766236736636));
#50989=CARTESIAN_POINT('',(-14.8,-1.954,-2.39295984553393E-16));
#50990=CARTESIAN_POINT('Ctrl Pts',(-9.12013030787577,-1.9535529839402,-0.00178040573474675));
#50991=CARTESIAN_POINT('Ctrl Pts',(-9.14770485027428,-1.94921168804754,
0.481988254547837));
#50992=CARTESIAN_POINT('Ctrl Pts',(-9.17527939267279,-1.76751241565099,
0.968669397052054));
#50993=CARTESIAN_POINT('Ctrl Pts',(-9.2028539350713,-1.4419965923978,1.32336557286795));
#50994=CARTESIAN_POINT('Ctrl Pts',(-9.2399027166971,-1.00463794190191,1.79993054977301));
#50995=CARTESIAN_POINT('Ctrl Pts',(-9.27695149832291,-0.307658121980692,
2.03823302355113));
#50996=CARTESIAN_POINT('Ctrl Pts',(-9.31400027994872,0.329921663003375,
1.92919732226127));
#50997=CARTESIAN_POINT('Ctrl Pts',(-9.35104906157453,0.967501447987441,
1.82016162097141));
#50998=CARTESIAN_POINT('Ctrl Pts',(-9.38809784320034,1.54568119803435,1.36378774461357));
#50999=CARTESIAN_POINT('Ctrl Pts',(-9.42514662482614,1.79981680878709,0.768966882737124));
#51000=CARTESIAN_POINT('Ctrl Pts',(-9.46219540645195,2.05395241953981,0.174146020860696));
#51001=CARTESIAN_POINT('Ctrl Pts',(-9.49924418807775,1.98404389099838,-0.559121826534324));
#51002=CARTESIAN_POINT('Ctrl Pts',(-9.53629296970356,1.62208971484511,-1.09520571991416));
#51003=CARTESIAN_POINT('Ctrl Pts',(-9.57334175132937,1.26013553869183,-1.63128961329401));
#51004=CARTESIAN_POINT('Ctrl Pts',(-9.61039053295519,0.606135714926695,
-1.97018955265867));
#51005=CARTESIAN_POINT('Ctrl Pts',(-9.64743931458099,-0.0405613313352086,
-1.95678445168069));
#51006=CARTESIAN_POINT('Ctrl Pts',(-9.6844880962068,-0.687258377597112,
-1.94337935070271));
#51007=CARTESIAN_POINT('Ctrl Pts',(-9.7215368778326,-1.32665264635579,-1.57766920938208));
#51008=CARTESIAN_POINT('Ctrl Pts',(-9.75858565945841,-1.66608095877641,
-1.02704666434474));
#51009=CARTESIAN_POINT('Ctrl Pts',(-9.77910054226419,-1.8540313243405,-0.722152508964587));
#51010=CARTESIAN_POINT('Ctrl Pts',(-9.79961542506998,-1.95000830113878,
-0.360561851747099));
#51011=CARTESIAN_POINT('Ctrl Pts',(-9.82013030787577,-1.95094521463585,
0.000565864204244704));
#51012=CARTESIAN_POINT('Ctrl Pts',(-9.92186969212419,-1.95087369540874,
0.000415097647679855));
#51013=CARTESIAN_POINT('Ctrl Pts',(-9.90189666535567,-1.95020594369431,
-0.351206366407061));
#51014=CARTESIAN_POINT('Ctrl Pts',(-9.88192363858714,-1.85952426139783,
-0.703148983685942));
#51015=CARTESIAN_POINT('Ctrl Pts',(-9.86195061181862,-1.68088875115348,
-1.00262828611878));
#51016=CARTESIAN_POINT('Ctrl Pts',(-9.82490183019282,-1.34953046047678,
-1.55814465356138));
#51017=CARTESIAN_POINT('Ctrl Pts',(-9.78785304856701,-0.715540176389686,
-1.93314497158098));
#51018=CARTESIAN_POINT('Ctrl Pts',(-9.7508042669412,-0.0691075689552816,
-1.95598430918883));
#51019=CARTESIAN_POINT('Ctrl Pts',(-9.71375548531539,0.577325038479105,
-1.97882364679667));
#51020=CARTESIAN_POINT('Ctrl Pts',(-9.67670670368958,1.23619996926078,-1.64950200399279));
#51021=CARTESIAN_POINT('Ctrl Pts',(-9.63965792206377,1.60593736708061,-1.11875629468351));
#51022=CARTESIAN_POINT('Ctrl Pts',(-9.60260914043797,1.97567476490046,-0.588010585374225));
#51023=CARTESIAN_POINT('Ctrl Pts',(-9.56556035881216,2.05627462975842,0.14415919044051));
#51024=CARTESIAN_POINT('Ctrl Pts',(-9.52851157718636,1.81084483763096,0.742624701922234));
#51025=CARTESIAN_POINT('Ctrl Pts',(-9.49146279556055,1.56541504550351,1.34109021340394));
#51026=CARTESIAN_POINT('Ctrl Pts',(-9.45441401393473,0.993955596390669,
1.80585146055268));
#51027=CARTESIAN_POINT('Ctrl Pts',(-9.41736523230892,0.358034582351254,
1.92417819125994));
#51028=CARTESIAN_POINT('Ctrl Pts',(-9.38031645068311,-0.277886431688179,
2.04250492196719));
#51029=CARTESIAN_POINT('Ctrl Pts',(-9.34326766905731,-0.978269010654174,
1.81439713623294));
#51030=CARTESIAN_POINT('Ctrl Pts',(-9.30621888743151,-1.42253444126134,
1.34426419922019));
#51031=CARTESIAN_POINT('Ctrl Pts',(-9.27810248899574,-1.75968841259436,
0.987479322774409));
#51032=CARTESIAN_POINT('Ctrl Pts',(-9.24998609055996,-1.94933621795992,
0.491304318172266));
#51033=CARTESIAN_POINT('Ctrl Pts',(-9.22186969212419,-1.95383722770402,
-0.00178766236736636));
#51034=CARTESIAN_POINT('Origin',(-14.8,0.,0.));
#51035=CARTESIAN_POINT('',(-8.42013030787577,-1.95704676357205,0.000502930207441042));
#51036=CARTESIAN_POINT('',(-8.52186969212418,-1.95692604939057,0.000668243846604161));
#51037=CARTESIAN_POINT('',(-14.8,-1.954,-2.39295984553393E-16));
#51038=CARTESIAN_POINT('Ctrl Pts',(-8.42013030787577,-1.95704676357205,
0.000502930207441042));
#51039=CARTESIAN_POINT('Ctrl Pts',(-8.42169671222696,-1.95714101498148,
0.0278567662564005));
#51040=CARTESIAN_POINT('Ctrl Pts',(-8.42326311657814,-1.95661716157646,
0.0552069111146564));
#51041=CARTESIAN_POINT('Ctrl Pts',(-8.42482952092933,-1.95546396780841,
0.0825304946185233));
#51042=CARTESIAN_POINT('Ctrl Pts',(-8.46187830255513,-1.92818849193753,
0.728791134602187));
#51043=CARTESIAN_POINT('Ctrl Pts',(-8.49892708418095,-1.54884571939758,
1.36019274950974));
#51044=CARTESIAN_POINT('Ctrl Pts',(-8.53597586580676,-0.991068206975607,
1.6877305534537));
#51045=CARTESIAN_POINT('Ctrl Pts',(-8.57302464743257,-0.433290694553603,
2.01526835739768));
#51046=CARTESIAN_POINT('Ctrl Pts',(-8.61007342905837,0.302921557750443,
2.03894235037805));
#51047=CARTESIAN_POINT('Ctrl Pts',(-8.64712221068418,0.880589899072553,
1.74791648587407));
#51048=CARTESIAN_POINT('Ctrl Pts',(-8.68417099230999,1.45825824039463,1.45689062137012));
#51049=CARTESIAN_POINT('Ctrl Pts',(-8.7212197739358,1.8773826707348,0.851164899381864));
#51050=CARTESIAN_POINT('Ctrl Pts',(-8.75826855556161,1.94612179566075,0.207991750781512));
#51051=CARTESIAN_POINT('Ctrl Pts',(-8.79531733718741,2.0148609205867,-0.435181397818841));
#51052=CARTESIAN_POINT('Ctrl Pts',(-8.83236611881321,1.73321474009845,-1.11580197303129));
#51053=CARTESIAN_POINT('Ctrl Pts',(-8.86941490043902,1.23009818277112,-1.52233671462071));
#51054=CARTESIAN_POINT('Ctrl Pts',(-8.90646368206483,0.726981625443756,
-1.92887145621015));
#51055=CARTESIAN_POINT('Ctrl Pts',(-8.94351246369065,0.00239469127729805,
-2.06132036417651));
#51056=CARTESIAN_POINT('Ctrl Pts',(-8.98056124531646,-0.612005102830212,
-1.8590590001527));
#51057=CARTESIAN_POINT('Ctrl Pts',(-9.01761002694226,-1.22640489693769,
-1.6567976361289));
#51058=CARTESIAN_POINT('Ctrl Pts',(-9.05465880856807,-1.73061755098623,
-1.11982600011496));
#51059=CARTESIAN_POINT('Ctrl Pts',(-9.09170759019387,-1.89385513747523,
-0.493926442092014));
#51060=CARTESIAN_POINT('Ctrl Pts',(-9.10118182942117,-1.93559880291891,
-0.333869298921619));
#51061=CARTESIAN_POINT('Ctrl Pts',(-9.11065606864847,-1.95504459439919,
-0.167996763995528));
#51062=CARTESIAN_POINT('Ctrl Pts',(-9.12013030787577,-1.9535529839402,-0.00178040573474675));
#51063=CARTESIAN_POINT('Ctrl Pts',(-9.22186969212419,-1.95383722770402,
-0.00178766236736636));
#51064=CARTESIAN_POINT('Ctrl Pts',(-9.21293730893415,-1.95526716702816,
-0.158439536830396));
#51065=CARTESIAN_POINT('Ctrl Pts',(-9.20400492574411,-1.93801045369618,
-0.314780245228718));
#51066=CARTESIAN_POINT('Ctrl Pts',(-9.19507254255408,-1.90086016391406,
-0.466241472977706));
#51067=CARTESIAN_POINT('Ctrl Pts',(-9.15802376092827,-1.7467721737113,-1.09445611987165));
#51068=CARTESIAN_POINT('Ctrl Pts',(-9.12097497930247,-1.25044791105744,
-1.63872732536828));
#51069=CARTESIAN_POINT('Ctrl Pts',(-9.08392619767666,-0.639064633457673,
-1.84993158471966));
#51070=CARTESIAN_POINT('Ctrl Pts',(-9.04687741605085,-0.0276813558578867,
-2.06113584407105));
#51071=CARTESIAN_POINT('Ctrl Pts',(-9.00982863442504,0.698760936687822,
-1.93927315727717));
#51072=CARTESIAN_POINT('Ctrl Pts',(-8.97277985279923,1.20775549370569,-1.54012244360749));
#51073=CARTESIAN_POINT('Ctrl Pts',(-8.93573107117342,1.71675005072351,-1.14097172993785));
#51074=CARTESIAN_POINT('Ctrl Pts',(-8.89868228954762,2.00829687221353,-0.464532989392456));
#51075=CARTESIAN_POINT('Ctrl Pts',(-8.86163350792181,1.94894931386644,0.179574624764523));
#51076=CARTESIAN_POINT('Ctrl Pts',(-8.824584726296,1.88960175551935,0.823682238921539));
#51077=CARTESIAN_POINT('Ctrl Pts',(-8.7875359446702,1.4793598173351,1.43545872669014));
#51078=CARTESIAN_POINT('Ctrl Pts',(-8.75048716304439,0.905999204518953,
1.73488210414737));
#51079=CARTESIAN_POINT('Ctrl Pts',(-8.71343838141858,0.332638591702826,
2.0343054816046));
#51080=CARTESIAN_POINT('Ctrl Pts',(-8.67638959979277,-0.403840695745188,
2.02137574875049));
#51081=CARTESIAN_POINT('Ctrl Pts',(-8.63934081816697,-0.966337779787842,
1.70201109550863));
#51082=CARTESIAN_POINT('Ctrl Pts',(-8.60229203654116,-1.52883486383051,
1.38264644226677));
#51083=CARTESIAN_POINT('Ctrl Pts',(-8.56524325491535,-1.91734974446781,
0.756846868637128));
#51084=CARTESIAN_POINT('Ctrl Pts',(-8.52819447328954,-1.95405161284264,
0.111052997378969));
#51085=CARTESIAN_POINT('Ctrl Pts',(-8.52608621290109,-1.95614013213751,
0.0743041063727897));
#51086=CARTESIAN_POINT('Ctrl Pts',(-8.52397795251263,-1.9570894184881,0.0374904702839609));
#51087=CARTESIAN_POINT('Ctrl Pts',(-8.52186969212418,-1.95692604939057,
0.000668243846604161));
#51088=CARTESIAN_POINT('Origin',(-14.8,0.,0.));
#51089=CARTESIAN_POINT('',(-7.72013030787578,-1.95207303808925,0.00146614720672802));
#51090=CARTESIAN_POINT('',(-7.82186969212419,-1.95186016998754,0.00136964534846597));
#51091=CARTESIAN_POINT('',(-14.8,-1.954,-2.39295984553393E-16));
#51092=CARTESIAN_POINT('Ctrl Pts',(-7.72013030787578,-1.95207303808925,
0.00146614720672802));
#51093=CARTESIAN_POINT('Ctrl Pts',(-7.73273735580545,-1.95361829365223,
0.223069353944344));
#51094=CARTESIAN_POINT('Ctrl Pts',(-7.74534440373512,-1.91879720445243,
0.444201465762539));
#51095=CARTESIAN_POINT('Ctrl Pts',(-7.75795145166479,-1.84550193984431,
0.651746271159146));
#51096=CARTESIAN_POINT('Ctrl Pts',(-7.7950002332906,-1.63010653024322,1.26166559688908));
#51097=CARTESIAN_POINT('Ctrl Pts',(-7.8320490149164,-1.08244170036397,1.75424266953811));
#51098=CARTESIAN_POINT('Ctrl Pts',(-7.86909779654221,-0.453184282765084,
1.90401539326595));
#51099=CARTESIAN_POINT('Ctrl Pts',(-7.90614657816802,0.176073134833824,
2.05378811699378));
#51100=CARTESIAN_POINT('Ctrl Pts',(-7.94319535979383,0.886923140152381,
1.8607564918004));
#51101=CARTESIAN_POINT('Ctrl Pts',(-7.98024414141964,1.35399587550455,1.41327484271661));
#51102=CARTESIAN_POINT('Ctrl Pts',(-8.01729292304545,1.82106861085671,0.965793193632821));
#51103=CARTESIAN_POINT('Ctrl Pts',(-8.05434170467126,2.04436407624249,0.263861520658632));
#51104=CARTESIAN_POINT('Ctrl Pts',(-8.09139048629706,1.92167559901516,-0.371232412497511));
#51105=CARTESIAN_POINT('Ctrl Pts',(-8.12843926792287,1.79898712178783,-1.00632634565364));
#51106=CARTESIAN_POINT('Ctrl Pts',(-8.16548804954867,1.33031470194742,-1.57458253899172));
#51107=CARTESIAN_POINT('Ctrl Pts',(-8.20253683117448,0.730178811328908,
-1.81589909285326));
#51108=CARTESIAN_POINT('Ctrl Pts',(-8.23958561280029,0.130042920710383,
-2.0572156467148));
#51109=CARTESIAN_POINT('Ctrl Pts',(-8.27663439442611,-0.601556440686245,
-1.97159256109978));
#51110=CARTESIAN_POINT('Ctrl Pts',(-8.31368317605191,-1.12975203178366,
-1.59822118576237));
#51111=CARTESIAN_POINT('Ctrl Pts',(-8.34916555332654,-1.63561577184945,
-1.24063576940312));
#51112=CARTESIAN_POINT('Ctrl Pts',(-8.38464793060115,-1.95491176945909,
-0.619119410514391));
#51113=CARTESIAN_POINT('Ctrl Pts',(-8.42013030787577,-1.95704676357205,
0.000502930207441042));
#51114=CARTESIAN_POINT('Ctrl Pts',(-8.52186969212418,-1.95692604939057,
0.000668243846604161));
#51115=CARTESIAN_POINT('Ctrl Pts',(-8.48692917088682,-1.95421850839941,
-0.609592135700733));
#51116=CARTESIAN_POINT('Ctrl Pts',(-8.45198864964947,-1.64589857568518,
-1.22221202102663));
#51117=CARTESIAN_POINT('Ctrl Pts',(-8.41704812841211,-1.15295067365337,
-1.58156732958228));
#51118=CARTESIAN_POINT('Ctrl Pts',(-8.37999934678631,-0.630259009976949,
-1.96260561639862));
#51119=CARTESIAN_POINT('Ctrl Pts',(-8.34295056516051,0.100013173488252,
-2.05889402114469));
#51120=CARTESIAN_POINT('Ctrl Pts',(-8.3059017835347,0.703606110788312,-1.82635947029634));
#51121=CARTESIAN_POINT('Ctrl Pts',(-8.26885300190889,1.30719904808841,-1.59382491944798));
#51122=CARTESIAN_POINT('Ctrl Pts',(-8.23180422028307,1.78411273922334,-1.03246741300516));
#51123=CARTESIAN_POINT('Ctrl Pts',(-8.19475543865726,1.91605452237685,-0.399231187608135));
#51124=CARTESIAN_POINT('Ctrl Pts',(-8.15770665703146,2.04799630553036,0.234005037788894));
#51125=CARTESIAN_POINT('Ctrl Pts',(-8.12065787540566,1.83496618070244,0.939119982140134));
#51126=CARTESIAN_POINT('Ctrl Pts',(-8.08360909377985,1.3744721747335,1.3933688365839));
#51127=CARTESIAN_POINT('Ctrl Pts',(-8.04656031215404,0.913978168764561,
1.84761769102765));
#51128=CARTESIAN_POINT('Ctrl Pts',(-8.00951153052823,0.206020281654609,
2.05100045556395));
#51129=CARTESIAN_POINT('Ctrl Pts',(-7.97246274890242,-0.425355407601904,
1.91042488758486));
#51130=CARTESIAN_POINT('Ctrl Pts',(-7.93541396727661,-1.05673109685843,
1.76984931960576));
#51131=CARTESIAN_POINT('Ctrl Pts',(-7.89836518565081,-1.61152458826152,
1.28531541911125));
#51132=CARTESIAN_POINT('Ctrl Pts',(-7.861316404025,-1.83579612237898,0.678603765785385));
#51133=CARTESIAN_POINT('Ctrl Pts',(-7.84816750005806,-1.91539185360739,
0.463277028572364));
#51134=CARTESIAN_POINT('Ctrl Pts',(-7.83501859609112,-1.95335517386918,
0.232560831431699));
#51135=CARTESIAN_POINT('Ctrl Pts',(-7.82186969212419,-1.95186016998754,
0.00136964534846597));
#51136=CARTESIAN_POINT('Origin',(-14.8,0.,0.));
#51137=CARTESIAN_POINT('',(-7.02013030787579,-1.95176668991016,-0.00132109256869101));
#51138=CARTESIAN_POINT('',(-7.12186969212419,-1.9519719800925,-0.00142259664250751));
#51139=CARTESIAN_POINT('',(-14.8,-1.954,-2.39295984553393E-16));
#51140=CARTESIAN_POINT('Ctrl Pts',(-7.02013030787579,-1.95176668991016,
-0.00132109256869101));
#51141=CARTESIAN_POINT('Ctrl Pts',(-7.04377799938394,-1.94918116590277,
0.414515544669262));
#51142=CARTESIAN_POINT('Ctrl Pts',(-7.0674256908921,-1.81911222147843,0.831829046295296));
#51143=CARTESIAN_POINT('Ctrl Pts',(-7.09107338240025,-1.57361703474163,
1.16377834655484));
#51144=CARTESIAN_POINT('Ctrl Pts',(-7.12812216402606,-1.18900031388915,
1.68384251991882));
#51145=CARTESIAN_POINT('Ctrl Pts',(-7.16517094565186,-0.521065104670545,
1.99437672845672));
#51146=CARTESIAN_POINT('Ctrl Pts',(-7.20221972727767,0.124461671143169,
1.95324343192425));
#51147=CARTESIAN_POINT('Ctrl Pts',(-7.23926850890348,0.769988446956902,
1.91211013539178));
#51148=CARTESIAN_POINT('Ctrl Pts',(-7.2763172905293,1.39310678936575,1.51930933378892));
#51149=CARTESIAN_POINT('Ctrl Pts',(-7.31336607215511,1.70860332723064,0.954633585264722));
#51150=CARTESIAN_POINT('Ctrl Pts',(-7.35041485378091,2.02409986509553,0.389957836740521));
#51151=CARTESIAN_POINT('Ctrl Pts',(-7.38746363540671,2.03197459841647,-0.346592858705026));
#51152=CARTESIAN_POINT('Ctrl Pts',(-7.42451241703252,1.72862310876371,-0.917884938206884));
#51153=CARTESIAN_POINT('Ctrl Pts',(-7.46156119865832,1.42527161911097,-1.48917701770873));
#51154=CARTESIAN_POINT('Ctrl Pts',(-7.49860998028414,0.810693906484552,
-1.89521048126689));
#51155=CARTESIAN_POINT('Ctrl Pts',(-7.53565876190995,0.166194129846451,
-1.95013592427388));
#51156=CARTESIAN_POINT('Ctrl Pts',(-7.57270754353575,-0.478305646791669,
-2.00506136728088));
#51157=CARTESIAN_POINT('Ctrl Pts',(-7.60975632516156,-1.15272748744147,
-1.70887878973669));
#51158=CARTESIAN_POINT('Ctrl Pts',(-7.64680510678737,-1.54837541310491,
-1.19715671155917));
#51159=CARTESIAN_POINT('Ctrl Pts',(-7.6712468404835,-1.80939131732991,-0.859564644765363));
#51160=CARTESIAN_POINT('Ctrl Pts',(-7.69568857417964,-1.94907719598778,
-0.428163897471984));
#51161=CARTESIAN_POINT('Ctrl Pts',(-7.72013030787578,-1.95207303808925,
0.00146614720672802));
#51162=CARTESIAN_POINT('Ctrl Pts',(-7.82186969212419,-1.95186016998754,
0.00136964534846597));
#51163=CARTESIAN_POINT('Ctrl Pts',(-7.79796981446532,-1.94914280206391,
-0.418851011604582));
#51164=CARTESIAN_POINT('Ctrl Pts',(-7.77406993680645,-1.81606347314505,
-0.840640931605373));
#51165=CARTESIAN_POINT('Ctrl Pts',(-7.75017005914758,-1.56567773577053,
-1.17443761077048));
#51166=CARTESIAN_POINT('Ctrl Pts',(-7.71312127752177,-1.17753823821277,
-1.69187792784332));
#51167=CARTESIAN_POINT('Ctrl Pts',(-7.67607249589596,-0.507509666265409,
-1.99786915583173));
#51168=CARTESIAN_POINT('Ctrl Pts',(-7.63902371427015,0.137722885510151,
-1.95235316494904));
#51169=CARTESIAN_POINT('Ctrl Pts',(-7.60197493264435,0.782955437285656,
-1.90683717406636));
#51170=CARTESIAN_POINT('Ctrl Pts',(-7.56492615101854,1.40339196888934,-1.50981396431264));
#51171=CARTESIAN_POINT('Ctrl Pts',(-7.52787736939273,1.7150466260894,-0.943008772079646));
#51172=CARTESIAN_POINT('Ctrl Pts',(-7.49082858776692,2.02670128328947,-0.376203579846622));
#51173=CARTESIAN_POINT('Ctrl Pts',(-7.45377980614111,2.02957406608585,0.360383594865731));
#51174=CARTESIAN_POINT('Ctrl Pts',(-7.41673102451531,1.72235004598079,0.929602491923175));
#51175=CARTESIAN_POINT('Ctrl Pts',(-7.3796822428895,1.41512602587571,1.49882138898064));
#51176=CARTESIAN_POINT('Ctrl Pts',(-7.34263346126368,0.797805202869196,
1.90067200838321));
#51177=CARTESIAN_POINT('Ctrl Pts',(-7.30558467963788,0.152947310836807,
1.95121951455688));
#51178=CARTESIAN_POINT('Ctrl Pts',(-7.26853589801207,-0.491910581195545,
2.00176702073054));
#51179=CARTESIAN_POINT('Ctrl Pts',(-7.23148711638627,-1.16430554225374,
1.70101141367534));
#51180=CARTESIAN_POINT('Ctrl Pts',(-7.19443833476046,-1.55646933550666,
1.18661437776021));
#51181=CARTESIAN_POINT('Ctrl Pts',(-7.17024878721504,-1.81251728920985,
0.850759026748462));
#51182=CARTESIAN_POINT('Ctrl Pts',(-7.14605923966961,-1.94910481502684,
0.423829950049081));
#51183=CARTESIAN_POINT('Ctrl Pts',(-7.12186969212419,-1.9519719800925,-0.00142259664250751));
#51184=CARTESIAN_POINT('Origin',(-14.8,0.,0.));
#51185=CARTESIAN_POINT('',(-6.32013030787579,-1.95685981962429,-0.000742816091480747));
#51186=CARTESIAN_POINT('',(-6.4218696921242,-1.95699436955386,-0.000580667263057569));
#51187=CARTESIAN_POINT('',(-14.8,-1.954,-2.39295984553393E-16));
#51188=CARTESIAN_POINT('Ctrl Pts',(-6.32013030787579,-1.95685981962429,
-0.000742816091480747));
#51189=CARTESIAN_POINT('Ctrl Pts',(-6.35481864296243,-1.9539129004879,0.60516754541605));
#51190=CARTESIAN_POINT('Ctrl Pts',(-6.38950697804907,-1.65062025506416,
1.21362467071175));
#51191=CARTESIAN_POINT('Ctrl Pts',(-6.42419531313571,-1.16366421853117,
1.57370143243539));
#51192=CARTESIAN_POINT('Ctrl Pts',(-6.46124409476151,-0.643572152601299,
1.95828043515508));
#51193=CARTESIAN_POINT('Ctrl Pts',(-6.49829287638732,0.0860293302205446,
2.05952575430774));
#51194=CARTESIAN_POINT('Ctrl Pts',(-6.53534165801313,0.691187456695122,
1.83109544034338));
#51195=CARTESIAN_POINT('Ctrl Pts',(-6.57239043963894,1.29634558316972,1.60266512637901));
#51196=CARTESIAN_POINT('Ctrl Pts',(-6.60943922126475,1.77706035329704,1.04455917929761));
#51197=CARTESIAN_POINT('Ctrl Pts',(-6.64648800289056,1.9132992775594,0.412233533849047));
#51198=CARTESIAN_POINT('Ctrl Pts',(-6.68353678451637,2.04953820182175,-0.22009211159951));
#51199=CARTESIAN_POINT('Ctrl Pts',(-6.72058556614217,1.84130128021915,-0.926637455415224));
#51200=CARTESIAN_POINT('Ctrl Pts',(-6.75763434776798,1.38390259735436,-1.384002967112));
#51201=CARTESIAN_POINT('Ctrl Pts',(-6.79468312939378,0.926503914489585,
-1.84136847880877));
#51202=CARTESIAN_POINT('Ctrl Pts',(-6.83173191101959,0.219943470362641,
-2.04955415838662));
#51203=CARTESIAN_POINT('Ctrl Pts',(-6.8687806926454,-0.412372292834584,
-1.91326937571303));
#51204=CARTESIAN_POINT('Ctrl Pts',(-6.90582947427121,-1.04468805603181,
-1.77698459303944));
#51205=CARTESIAN_POINT('Ctrl Pts',(-6.94287825589702,-1.60275913829931,
-1.2962293481144));
#51206=CARTESIAN_POINT('Ctrl Pts',(-6.97992703752283,-1.8311455631899,-0.691054656556856));
#51207=CARTESIAN_POINT('Ctrl Pts',(-6.99332812764048,-1.91375629766748,
-0.472154055171452));
#51208=CARTESIAN_POINT('Ctrl Pts',(-7.00672921775813,-1.95323190017021,
-0.23697471854422));
#51209=CARTESIAN_POINT('Ctrl Pts',(-7.02013030787579,-1.95176668991016,
-0.00132109256869101));
#51210=CARTESIAN_POINT('Ctrl Pts',(-7.12186969212419,-1.9519719800925,-0.00142259664250751));
#51211=CARTESIAN_POINT('Ctrl Pts',(-7.1090104580438,-1.95349617341018,-0.227488091704733));
#51212=CARTESIAN_POINT('Ctrl Pts',(-7.09615122396341,-1.91723077036094,
-0.453079796598166));
#51213=CARTESIAN_POINT('Ctrl Pts',(-7.08329198988303,-1.84103347457747,
-0.66426366705173));
#51214=CARTESIAN_POINT('Ctrl Pts',(-7.04624320825722,-1.62150119494774,
-1.27270621117352));
#51215=CARTESIAN_POINT('Ctrl Pts',(-7.00919442663142,-1.07050401024064,
-1.76155283464202));
#51216=CARTESIAN_POINT('Ctrl Pts',(-6.97214564500561,-0.440244036559741,
-1.90704894068122));
#51217=CARTESIAN_POINT('Ctrl Pts',(-6.9350968633798,0.190015937121125,-2.05254504672042));
#51218=CARTESIAN_POINT('Ctrl Pts',(-6.89804808175399,0.899538699775802,
-1.85469063533038));
#51219=CARTESIAN_POINT('Ctrl Pts',(-6.86099930012818,1.36356189847091,-1.40404751448026));
#51220=CARTESIAN_POINT('Ctrl Pts',(-6.82395051850237,1.82758509716603,-0.95340439363013));
#51221=CARTESIAN_POINT('Ctrl Pts',(-6.78690173687657,2.04610873190157,-0.249972563319941));
#51222=CARTESIAN_POINT('Ctrl Pts',(-6.74985295525077,1.91911028962563,0.384273561584486));
#51223=CARTESIAN_POINT('Ctrl Pts',(-6.71280417362496,1.79211184734969,1.0185196864889));
#51224=CARTESIAN_POINT('Ctrl Pts',(-6.67575539199914,1.31959132806222,1.58358010598756));
#51225=CARTESIAN_POINT('Ctrl Pts',(-6.63870661037333,0.717830553475292,
1.82081568819503));
#51226=CARTESIAN_POINT('Ctrl Pts',(-6.60165782874752,0.11606977888833,2.05805127040252));
#51227=CARTESIAN_POINT('Ctrl Pts',(-6.56460904712172,-0.614931250998082,
1.96746201531886));
#51228=CARTESIAN_POINT('Ctrl Pts',(-6.52756026549591,-1.14057916306319,
1.59051238494576));
#51229=CARTESIAN_POINT('Ctrl Pts',(-6.49233007437201,-1.64042492298516,
1.23206584664237));
#51230=CARTESIAN_POINT('Ctrl Pts',(-6.45709988324811,-1.95458285395145,
0.614681742887991));
#51231=CARTESIAN_POINT('Ctrl Pts',(-6.4218696921242,-1.95699436955386,-0.000580667263057569));
#51232=CARTESIAN_POINT('Origin',(-14.8,0.,0.));
#51233=CARTESIAN_POINT('',(-5.62013030787578,-1.95397084692293,0.00178599170134505));
#51234=CARTESIAN_POINT('',(-5.7218696921242,-1.9536847040016,0.00178561523945243));
#51235=CARTESIAN_POINT('',(-14.8,-1.954,-2.39295984553393E-16));
#51236=CARTESIAN_POINT('Ctrl Pts',(-5.62013030787578,-1.95397084692293,
0.00178599170134505));
#51237=CARTESIAN_POINT('Ctrl Pts',(-5.6288105049151,-1.95536772671579,0.153988559362694));
#51238=CARTESIAN_POINT('Ctrl Pts',(-5.63749070195442,-1.93908361863309,
0.305895547971744));
#51239=CARTESIAN_POINT('Ctrl Pts',(-5.64617089899374,-1.90398252153289,
0.45332236833873));
#51240=CARTESIAN_POINT('Ctrl Pts',(-5.68321968061955,-1.75416416194949,
1.08256892216945));
#51241=CARTESIAN_POINT('Ctrl Pts',(-5.72026846224536,-1.26154737176521,
1.63019802696095));
#51242=CARTESIAN_POINT('Ctrl Pts',(-5.75731724387117,-0.651612426307885,
1.84554920222142));
#51243=CARTESIAN_POINT('Ctrl Pts',(-5.79436602549697,-0.0416774808505747,
2.06090037748189));
#51244=CARTESIAN_POINT('Ctrl Pts',(-5.83141480712278,0.68557561987972,1.94397362321138));
#51245=CARTESIAN_POINT('Ctrl Pts',(-5.86846358874859,1.19726900275107,1.54828858646908));
#51246=CARTESIAN_POINT('Ctrl Pts',(-5.9055123703744,1.70896238562244,1.15260354972677));
#51247=CARTESIAN_POINT('Ctrl Pts',(-5.94256115200021,2.00509605063479,0.478160230512601));
#51248=CARTESIAN_POINT('Ctrl Pts',(-5.97960993362602,1.95012386608632,-0.166335561019096));
#51249=CARTESIAN_POINT('Ctrl Pts',(-6.01665871525182,1.89515168153785,-0.810831352550793));
#51250=CARTESIAN_POINT('Ctrl Pts',(-6.05370749687763,1.48907364742859,-1.42537961640006));
#51251=CARTESIAN_POINT('Ctrl Pts',(-6.09075627850344,0.917759569173183,
-1.72868967288233));
#51252=CARTESIAN_POINT('Ctrl Pts',(-6.12780506012924,0.346445490917778,
-2.0319997293646));
#51253=CARTESIAN_POINT('Ctrl Pts',(-6.16485384175505,-0.390104631483775,
-2.02407157847987));
#51254=CARTESIAN_POINT('Ctrl Pts',(-6.20190262338086,-0.954757497459811,
-1.7085340889146));
#51255=CARTESIAN_POINT('Ctrl Pts',(-6.23895140500667,-1.51941036343583,
-1.39299659934935));
#51256=CARTESIAN_POINT('Ctrl Pts',(-6.27600018663248,-1.91216597298635,
-0.769849771103581));
#51257=CARTESIAN_POINT('Ctrl Pts',(-6.31304896825829,-1.95325245324266,
-0.124320013837331));
#51258=CARTESIAN_POINT('Ctrl Pts',(-6.31540941479745,-1.95587014904456,
-0.0831921166541531));
#51259=CARTESIAN_POINT('Ctrl Pts',(-6.31776986133662,-1.95706034942947,
-0.0419733626799344));
#51260=CARTESIAN_POINT('Ctrl Pts',(-6.32013030787579,-1.95685981962429,
-0.000742816091480747));
#51261=CARTESIAN_POINT('Ctrl Pts',(-6.4218696921242,-1.95699436955386,-0.000580667263057569));
#51262=CARTESIAN_POINT('Ctrl Pts',(-6.4200511016223,-1.95711885253933,-0.032340653217794));
#51263=CARTESIAN_POINT('Ctrl Pts',(-6.4182325111204,-1.95641264107839,-0.0640949856060214));
#51264=CARTESIAN_POINT('Ctrl Pts',(-6.41641392061849,-1.95485839584589,
-0.0958077557958485));
#51265=CARTESIAN_POINT('Ctrl Pts',(-6.37936513899268,-1.92319492231974,
-0.741868260501935));
#51266=CARTESIAN_POINT('Ctrl Pts',(-6.34231635736687,-1.53957318102366,
-1.3706792642516));
#51267=CARTESIAN_POINT('Ctrl Pts',(-6.30526757574106,-0.979584295875341,
-1.69442175421417));
#51268=CARTESIAN_POINT('Ctrl Pts',(-6.26821879411526,-0.419595410727051,
-2.01816424417671));
#51269=CARTESIAN_POINT('Ctrl Pts',(-6.23117001248945,0.316760618273472,
-2.03683822035221));
#51270=CARTESIAN_POINT('Ctrl Pts',(-6.19412123086365,0.892439330875022,
-1.74189624105086));
#51271=CARTESIAN_POINT('Ctrl Pts',(-6.15707244923784,1.46811804347659,-1.44695426174951));
#51272=CARTESIAN_POINT('Ctrl Pts',(-6.12002366761203,1.88311943967917,-0.838396326971331));
#51273=CARTESIAN_POINT('Ctrl Pts',(-6.08297488598622,1.94748931787675,-0.194771226406078));
#51274=CARTESIAN_POINT('Ctrl Pts',(-6.04592610436041,2.01185919607434,0.448853874159157));
#51275=CARTESIAN_POINT('Ctrl Pts',(-6.00887732273461,1.72559755626691,1.12754614051143));
#51276=CARTESIAN_POINT('Ctrl Pts',(-5.9718285411088,1.21973191242823,1.53065493684369));
#51277=CARTESIAN_POINT('Ctrl Pts',(-5.93477975948299,0.713866268589532,
1.93376373317597));
#51278=CARTESIAN_POINT('Ctrl Pts',(-5.89773097785719,-0.0116033792804625,
2.06128905948823));
#51279=CARTESIAN_POINT('Ctrl Pts',(-5.86068219623138,-0.624615479072405,
1.85486009639081));
#51280=CARTESIAN_POINT('Ctrl Pts',(-5.82363341460557,-1.23762757886435,
1.6484311332934));
#51281=CARTESIAN_POINT('Ctrl Pts',(-5.78658463297976,-1.73818213057826,
1.10804788078631));
#51282=CARTESIAN_POINT('Ctrl Pts',(-5.74953585135395,-1.89716559122094,
0.481054251999797));
#51283=CARTESIAN_POINT('Ctrl Pts',(-5.74031379827737,-1.93673919790939,
0.32498519197648));
#51284=CARTESIAN_POINT('Ctrl Pts',(-5.73109174520078,-1.95514925643464,
0.163549802899745));
#51285=CARTESIAN_POINT('Ctrl Pts',(-5.7218696921242,-1.9536847040016,0.00178561523945243));
#51286=CARTESIAN_POINT('Origin',(-14.8,0.,0.));
#51287=CARTESIAN_POINT('',(-4.9201303078758,-1.95084803715115,-0.000343805551916709));
#51288=CARTESIAN_POINT('',(-5.0218696921242,-1.95090916188199,-0.000496152702984699));
#51289=CARTESIAN_POINT('',(-14.8,-1.954,-2.39295984553393E-16));
#51290=CARTESIAN_POINT('Ctrl Pts',(-4.9201303078758,-1.95084803715115,-0.000343805551916709));
#51291=CARTESIAN_POINT('Ctrl Pts',(-4.9398511484936,-1.95030235658804,0.346849383744408));
#51292=CARTESIAN_POINT('Ctrl Pts',(-4.9595719891114,-1.86202658127011,0.694301680604123));
#51293=CARTESIAN_POINT('Ctrl Pts',(-4.97929282972921,-1.68765867280898,
0.991190605298301));
#51294=CARTESIAN_POINT('Ctrl Pts',(-5.01634161135502,-1.36008041748383,
1.54894436190979));
#51295=CARTESIAN_POINT('Ctrl Pts',(-5.05339039298082,-0.728651292790854,
1.92824134169696));
#51296=CARTESIAN_POINT('Ctrl Pts',(-5.09043917460663,-0.0823886763808118,
1.95546994810536));
#51297=CARTESIAN_POINT('Ctrl Pts',(-5.12748795623243,0.563873940029249,
1.98269855451377));
#51298=CARTESIAN_POINT('Ctrl Pts',(-5.16453673785825,1.2249700481564,1.65785878754338));
#51299=CARTESIAN_POINT('Ctrl Pts',(-5.20158551948405,1.59830311566784,1.12963611945859));
#51300=CARTESIAN_POINT('Ctrl Pts',(-5.23863430110986,1.97163618317925,0.601413451373826));
#51301=CARTESIAN_POINT('Ctrl Pts',(-5.27568308273567,2.05720621007502,-0.130192117825276));
#51302=CARTESIAN_POINT('Ctrl Pts',(-5.31273186436147,1.81584613260757,-0.730310505629698));
#51303=CARTESIAN_POINT('Ctrl Pts',(-5.34978064598728,1.57448605514012,-1.33042889343414));
#51304=CARTESIAN_POINT('Ctrl Pts',(-5.38682942761309,1.00619587330941,-1.79906009984386));
#51305=CARTESIAN_POINT('Ctrl Pts',(-5.4238782092389,0.371093043967381,-1.92170251721176));
#51306=CARTESIAN_POINT('Ctrl Pts',(-5.46092699086471,-0.264009785374633,
-2.04434493457966));
#51307=CARTESIAN_POINT('Ctrl Pts',(-5.49797577249051,-0.965925262227987,
-1.82099856290576));
#51308=CARTESIAN_POINT('Ctrl Pts',(-5.53502455411632,-1.4133730361634,-1.35389337563386));
#51309=CARTESIAN_POINT('Ctrl Pts',(-5.5633931387028,-1.75598781230169,-0.996226741687653));
#51310=CARTESIAN_POINT('Ctrl Pts',(-5.5917617232893,-1.94940557007707,-0.495641819605568));
#51311=CARTESIAN_POINT('Ctrl Pts',(-5.62013030787578,-1.95397084692293,
0.00178599170134505));
#51312=CARTESIAN_POINT('Ctrl Pts',(-5.7218696921242,-1.9536847040016,0.00178561523945243));
#51313=CARTESIAN_POINT('Ctrl Pts',(-5.69404296357498,-1.94926554672048,
-0.486323496866887));
#51314=CARTESIAN_POINT('Ctrl Pts',(-5.66621623502575,-1.76389259084126,
-0.977426245064707));
#51315=CARTESIAN_POINT('Ctrl Pts',(-5.63838950647653,-1.43297660565845,
-1.33312734632344));
#51316=CARTESIAN_POINT('Ctrl Pts',(-5.60134072485072,-0.99239178988181,
-1.80671131079422));
#51317=CARTESIAN_POINT('Ctrl Pts',(-5.56429194322491,-0.293809788757061,
-2.04027523466985));
#51318=CARTESIAN_POINT('Ctrl Pts',(-5.5272431615991,0.343014843889603,-1.92691237235926));
#51319=CARTESIAN_POINT('Ctrl Pts',(-5.4901943799733,0.979839476536231,-1.81354951004867));
#51320=CARTESIAN_POINT('Ctrl Pts',(-5.45314559834749,1.55490674070476,-1.35325986155189));
#51321=CARTESIAN_POINT('Ctrl Pts',(-5.41609681672169,1.8049971772935,-0.756726941401114));
#51322=CARTESIAN_POINT('Ctrl Pts',(-5.37904803509588,2.05508761388226,-0.160194021250283));
#51323=CARTESIAN_POINT('Ctrl Pts',(-5.34199925347006,1.98020122289115,0.572582170554614));
#51324=CARTESIAN_POINT('Ctrl Pts',(-5.30495047184425,1.61461496035463,1.10619573479508));
#51325=CARTESIAN_POINT('Ctrl Pts',(-5.26790169021845,1.24902869781812,1.63980929903553));
#51326=CARTESIAN_POINT('Ctrl Pts',(-5.23085290859264,0.592742563736288,
1.97426023571157));
#51327=CARTESIAN_POINT('Ctrl Pts',(-5.19380412696683,-0.0538485281259382,
1.95646385346074));
#51328=CARTESIAN_POINT('Ctrl Pts',(-5.15675534534103,-0.700439619988128,
1.93866747120991));
#51329=CARTESIAN_POINT('Ctrl Pts',(-5.11970656371521,-1.33733566963071,
1.56862377003217));
#51330=CARTESIAN_POINT('Ctrl Pts',(-5.08265778208941,-1.67301698164315,
1.01570894109161));
#51331=CARTESIAN_POINT('Ctrl Pts',(-5.06239508543434,-1.85660759649205,
0.713309105975045));
#51332=CARTESIAN_POINT('Ctrl Pts',(-5.04213238877927,-1.95009861576432,
0.356208711437961));
#51333=CARTESIAN_POINT('Ctrl Pts',(-5.0218696921242,-1.95090916188199,-0.000496152702984699));
#51334=CARTESIAN_POINT('Origin',(-14.8,0.,0.));
#51335=CARTESIAN_POINT('',(-4.22013030787579,-1.95523249314758,-0.00160897937940108));
#51336=CARTESIAN_POINT('',(-4.32186969212421,-1.95550425013349,-0.00152907383372617));
#51337=CARTESIAN_POINT('',(-14.8,-1.954,-2.39295984553393E-16));
#51338=CARTESIAN_POINT('Ctrl Pts',(-4.22013030787579,-1.95523249314758,
-0.00160897937940108));
#51339=CARTESIAN_POINT('Ctrl Pts',(-4.25089179207208,-1.95045093383183,
0.536882135883852));
#51340=CARTESIAN_POINT('Ctrl Pts',(-4.28165327626837,-1.71897769238846,
1.07898378182717));
#51341=CARTESIAN_POINT('Ctrl Pts',(-4.31241476046466,-1.3232609900624,1.44209256433779));
#51342=CARTESIAN_POINT('Ctrl Pts',(-4.34946354209047,-0.846664295422686,
1.87941665129689));
#51343=CARTESIAN_POINT('Ctrl Pts',(-4.38651232371628,-0.131823927041808,
2.05710228976936));
#51344=CARTESIAN_POINT('Ctrl Pts',(-4.42356110534209,0.494063790696452,
1.89381931098549));
#51345=CARTESIAN_POINT('Ctrl Pts',(-4.46060988696789,1.11995150843469,1.73053633220162));
#51346=CARTESIAN_POINT('Ctrl Pts',(-4.4976586685937,1.6568865755303,1.22628473616144));
#51347=CARTESIAN_POINT('Ctrl Pts',(-4.53470745021951,1.85910338030663,0.611870274871573));
#51348=CARTESIAN_POINT('Ctrl Pts',(-4.57175623184532,2.06132018508296,-0.00254418641831178));
#51349=CARTESIAN_POINT('Ctrl Pts',(-4.60880501347113,1.92881872753997,-0.727121512957918));
#51350=CARTESIAN_POINT('Ctrl Pts',(-4.64585379509694,1.52224749900685,-1.23020858544655));
#51351=CARTESIAN_POINT('Ctrl Pts',(-4.68290257672275,1.11567627047375,-1.73329565793517));
#51352=CARTESIAN_POINT('Ctrl Pts',(-4.71995135834855,0.435035270950569,
-2.01489247637288));
#51353=CARTESIAN_POINT('Ctrl Pts',(-4.75700013997436,-0.20813289072373,
-1.9461067061541));
#51354=CARTESIAN_POINT('Ctrl Pts',(-4.79404892160016,-0.851301052398028,
-1.87732093593532));
#51355=CARTESIAN_POINT('Ctrl Pts',(-4.83109770322597,-1.45699637622342,
-1.45815257706005));
#51356=CARTESIAN_POINT('Ctrl Pts',(-4.86814648485178,-1.74798034515745,
-0.880463130904529));
#51357=CARTESIAN_POINT('Ctrl Pts',(-4.88547442585978,-1.88407532120525,
-0.610274255463677));
#51358=CARTESIAN_POINT('Ctrl Pts',(-4.90280236686779,-1.95132750558711,
-0.305409051963234));
#51359=CARTESIAN_POINT('Ctrl Pts',(-4.9201303078758,-1.95084803715115,-0.000343805551916709));
#51360=CARTESIAN_POINT('Ctrl Pts',(-5.0218696921242,-1.95090916188199,-0.000496152702984699));
#51361=CARTESIAN_POINT('Ctrl Pts',(-5.00508360715346,-1.95158063696922,
-0.295998684319199));
#51362=CARTESIAN_POINT('Ctrl Pts',(-4.98829752218272,-1.88864691667946,
-0.591229769456263));
#51363=CARTESIAN_POINT('Ctrl Pts',(-4.97151143721199,-1.76064068408562,
-0.854865401933136));
#51364=CARTESIAN_POINT('Ctrl Pts',(-4.93446265558618,-1.47811650013332,
-1.43673895931385));
#51365=CARTESIAN_POINT('Ctrl Pts',(-4.89741387396037,-0.878601557846366,
-1.86470011737183));
#51366=CARTESIAN_POINT('Ctrl Pts',(-4.86036509233456,-0.236505493565925,
-1.94286273972016));
#51367=CARTESIAN_POINT('Ctrl Pts',(-4.82331631070875,0.405590570714517,
-2.02102536206849));
#51368=CARTESIAN_POINT('Ctrl Pts',(-4.78626752908294,1.09026775698847,-1.74938944870716));
#51369=CARTESIAN_POINT('Ctrl Pts',(-4.74921874745714,1.50413601532688,-1.25228803446986));
#51370=CARTESIAN_POINT('Ctrl Pts',(-4.71216996583133,1.91800427366528,-0.755186620232563));
#51371=CARTESIAN_POINT('Ctrl Pts',(-4.67512118420552,2.06106360406817,-0.032619705119299));
#51372=CARTESIAN_POINT('Ctrl Pts',(-4.63807240257972,1.8678329716821,0.584679795937079));
#51373=CARTESIAN_POINT('Ctrl Pts',(-4.60102362095391,1.67460233929601,1.20197929699349));
#51374=CARTESIAN_POINT('Ctrl Pts',(-4.5639748393281,1.14508174412095,1.71401138399298));
#51375=CARTESIAN_POINT('Ctrl Pts',(-4.52692605770229,0.521643049988718,
1.88640902305896));
#51376=CARTESIAN_POINT('Ctrl Pts',(-4.48987727607648,-0.101795644143479,
2.05880666212493));
#51377=CARTESIAN_POINT('Ctrl Pts',(-4.45282849445068,-0.819152437232826,
1.89156985325739));
#51378=CARTESIAN_POINT('Ctrl Pts',(-4.41577971282487,-1.302079188418,1.46124613291825));
#51379=CARTESIAN_POINT('Ctrl Pts',(-4.38447637259131,-1.71011474955787,
1.09765604338717));
#51380=CARTESIAN_POINT('Ctrl Pts',(-4.35317303235776,-1.95079219889668,
0.546249885634487));
#51381=CARTESIAN_POINT('Ctrl Pts',(-4.32186969212421,-1.95550425013349,
-0.00152907383372617));
#51382=CARTESIAN_POINT('Origin',(-14.8,0.,0.));
#51383=CARTESIAN_POINT('',(-3.5201303078758,-1.95597299937839,0.001346970720391));
#51384=CARTESIAN_POINT('',(-3.6218696921242,-1.95572226229912,0.0014520242175467));
#51385=CARTESIAN_POINT('',(-14.8,-1.954,-2.39295984553393E-16));
#51386=CARTESIAN_POINT('Ctrl Pts',(-3.5201303078758,-1.95597299937839,0.001346970720391));
#51387=CARTESIAN_POINT('Ctrl Pts',(-3.52488365402476,-1.95662759721798,
0.0844741162826126));
#51388=CARTESIAN_POINT('Ctrl Pts',(-3.52963700017373,-1.95178720852235,
0.167524479998186));
#51389=CARTESIAN_POINT('Ctrl Pts',(-3.5343903463227,-1.94119380112327,0.249834421968559));
#51390=CARTESIAN_POINT('Ctrl Pts',(-3.57143912794851,-1.85862610563013,
0.891378919281443));
#51391=CARTESIAN_POINT('Ctrl Pts',(-3.60848790957432,-1.42656035489239,
1.48794251641861));
#51392=CARTESIAN_POINT('Ctrl Pts',(-3.64553669120012,-0.842761437094918,
1.76646646503613));
#51393=CARTESIAN_POINT('Ctrl Pts',(-3.68258547282593,-0.25896251929748,
2.04499041365363));
#51394=CARTESIAN_POINT('Ctrl Pts',(-3.71963425445174,0.476569565559663,
2.00547471375154));
#51395=CARTESIAN_POINT('Ctrl Pts',(-3.75668303607755,1.02716749245939,1.66600646888654));
#51396=CARTESIAN_POINT('Ctrl Pts',(-3.79373181770335,1.57776541935914,1.32653822402154));
#51397=CARTESIAN_POINT('Ctrl Pts',(-3.83078059932916,1.94342918830146,0.68711743419361));
#51398=CARTESIAN_POINT('Ctrl Pts',(-3.86782938095497,1.95678738820298,0.0404194174418129));
#51399=CARTESIAN_POINT('Ctrl Pts',(-3.90487816258078,1.97014558810449,-0.606278599309984));
#51400=CARTESIAN_POINT('Ctrl Pts',(-3.94192694420659,1.6311982189652,-1.26025384298565));
#51401=CARTESIAN_POINT('Ctrl Pts',(-3.9789757258324,1.0950880766397,-1.62216913925226));
#51402=CARTESIAN_POINT('Ctrl Pts',(-4.0160245074582,0.558977934314219,-1.98408443551887));
#51403=CARTESIAN_POINT('Ctrl Pts',(-4.05307328908401,-0.174294981197453,
-2.05393978437644));
#51404=CARTESIAN_POINT('Ctrl Pts',(-4.09012207070982,-0.769097410584957,
-1.79976103551835));
#51405=CARTESIAN_POINT('Ctrl Pts',(-4.12717085233562,-1.36389983997248,
-1.54558228666025));
#51406=CARTESIAN_POINT('Ctrl Pts',(-4.16421963396143,-1.82023178323582,
-0.967369440086464));
#51407=CARTESIAN_POINT('Ctrl Pts',(-4.20126841558724,-1.92922124441822,
-0.329781749076715));
#51408=CARTESIAN_POINT('Ctrl Pts',(-4.20755571301676,-1.94771710660494,
-0.221581066763726));
#51409=CARTESIAN_POINT('Ctrl Pts',(-4.21384301044628,-1.95620978947708,
-0.11167043750699));
#51410=CARTESIAN_POINT('Ctrl Pts',(-4.22013030787579,-1.95523249314758,
-0.00160897937940108));
#51411=CARTESIAN_POINT('Ctrl Pts',(-4.32186969212421,-1.95550425013349,
-0.00152907383372617));
#51412=CARTESIAN_POINT('Ctrl Pts',(-4.31612425073195,-1.95636910398029,
-0.102068884730967));
#51413=CARTESIAN_POINT('Ctrl Pts',(-4.3103788093397,-1.94928493475609,-0.202486505327942));
#51414=CARTESIAN_POINT('Ctrl Pts',(-4.30463336794745,-1.93382754467879,
-0.301598244891043));
#51415=CARTESIAN_POINT('Ctrl Pts',(-4.26758458632164,-1.83415244047339,
-0.940708270550516));
#51416=CARTESIAN_POINT('Ctrl Pts',(-4.23053580469583,-1.38630552278153,
-1.52551769005868));
#51417=CARTESIAN_POINT('Ctrl Pts',(-4.19348702307002,-0.795275026511071,
-1.78834787054631));
#51418=CARTESIAN_POINT('Ctrl Pts',(-4.15643824144421,-0.204244530240643,
-2.05117805103393));
#51419=CARTESIAN_POINT('Ctrl Pts',(-4.11938945981841,0.529969544608357,
-1.99202899250104));
#51420=CARTESIAN_POINT('Ctrl Pts',(-4.0823406781926,1.07130315181323,-1.63797436817403));
#51421=CARTESIAN_POINT('Ctrl Pts',(-4.04529189656679,1.61263675901812,-1.283919743847));
#51422=CARTESIAN_POINT('Ctrl Pts',(-4.00824311494098,1.96108989857888,-0.634959553725796));
#51423=CARTESIAN_POINT('Ctrl Pts',(-3.97119433331517,1.95716879884085,0.0118645153018863));
#51424=CARTESIAN_POINT('Ctrl Pts',(-3.93414555168936,1.95324769910283,0.65868858432955));
#51425=CARTESIAN_POINT('Ctrl Pts',(-3.89709677006356,1.59695236006608,1.30337653226371));
#51426=CARTESIAN_POINT('Ctrl Pts',(-3.86004798843775,1.05136608044181,1.65084216046714));
#51427=CARTESIAN_POINT('Ctrl Pts',(-3.82299920681194,0.505779800817546,
1.99830778867057));
#51428=CARTESIAN_POINT('Ctrl Pts',(-3.78595042518614,-0.229097419394216,
2.04855109714326));
#51429=CARTESIAN_POINT('Ctrl Pts',(-3.74890164356033,-0.816897999454004,
1.77857474747893));
#51430=CARTESIAN_POINT('Ctrl Pts',(-3.71185286193452,-1.40469857951381,
1.50859839781459));
#51431=CARTESIAN_POINT('Ctrl Pts',(-3.67480408030871,-1.84542251942161,
0.918402390013208));
#51432=CARTESIAN_POINT('Ctrl Pts',(-3.6377552986829,-1.93734190958681,0.278130903058121));
#51433=CARTESIAN_POINT('Ctrl Pts',(-3.63246009649667,-1.95047950101089,
0.186620013125221));
#51434=CARTESIAN_POINT('Ctrl Pts',(-3.62716489431044,-1.95649185444208,
0.0940862015967139));
#51435=CARTESIAN_POINT('Ctrl Pts',(-3.6218696921242,-1.95572226229912,0.00145202421754669));
#51436=CARTESIAN_POINT('Origin',(-14.8,0.,0.));
#51437=CARTESIAN_POINT('',(-2.8201303078758,-1.95107804107358,0.000764698408270981));
#51438=CARTESIAN_POINT('',(-2.92186969212421,-1.95097678997586,0.000619975964519355));
#51439=CARTESIAN_POINT('',(-14.8,-1.954,-2.39295984553393E-16));
#51440=CARTESIAN_POINT('Ctrl Pts',(-2.8201303078758,-1.95107804107358,0.000764698408270981));
#51441=CARTESIAN_POINT('Ctrl Pts',(-2.83592429760325,-1.95205660270951,
0.278742283343092));
#51442=CARTESIAN_POINT('Ctrl Pts',(-2.85171828733071,-1.89661935698062,
0.556347448730421));
#51443=CARTESIAN_POINT('Ctrl Pts',(-2.86751227705816,-1.78284755244559,
0.807530318679176));
#51444=CARTESIAN_POINT('Ctrl Pts',(-2.90456105868397,-1.51596712424919,
1.39674301651317));
#51445=CARTESIAN_POINT('Ctrl Pts',(-2.94160984030977,-0.928097750495292,
1.84056565868186));
#51446=CARTESIAN_POINT('Ctrl Pts',(-2.97865862193558,-0.288318663858768,
1.93585199861038));
#51447=CARTESIAN_POINT('Ctrl Pts',(-3.01570740356139,0.351460422777774,
2.0311383385389));
#51448=CARTESIAN_POINT('Ctrl Pts',(-3.0527561851872,1.04314922229697,1.77788837622724));
#51449=CARTESIAN_POINT('Ctrl Pts',(-3.08980496681301,1.47014833279873,1.29201953991286));
#51450=CARTESIAN_POINT('Ctrl Pts',(-3.12685374843881,1.8971474433005,0.806150703598486));
#51451=CARTESIAN_POINT('Ctrl Pts',(-3.16390253006462,2.05945686478485,0.0876629932813832));
#51452=CARTESIAN_POINT('Ctrl Pts',(-3.20095131169043,1.88278442191711,-0.534577807599872));
#51453=CARTESIAN_POINT('Ctrl Pts',(-3.23800009331624,1.70611197904937,-1.15681860848111));
#51454=CARTESIAN_POINT('Ctrl Pts',(-3.27504887494204,1.19045767182961,-1.68281249992648));
#51455=CARTESIAN_POINT('Ctrl Pts',(-3.31209765656785,0.571846494599176,
-1.87180185880745));
#51456=CARTESIAN_POINT('Ctrl Pts',(-3.34914643819366,-0.0467646826312976,
-2.06079121768844));
#51457=CARTESIAN_POINT('Ctrl Pts',(-3.38619521981947,-0.768332729872451,
-1.91277604400494));
#51458=CARTESIAN_POINT('Ctrl Pts',(-3.42324400144528,-1.26258193336873,
-1.49550575841888));
#51459=CARTESIAN_POINT('Ctrl Pts',(-3.45553943692212,-1.6934191312612,-1.13177110931077));
#51460=CARTESIAN_POINT('Ctrl Pts',(-3.48783487239896,-1.95152549616082,
-0.563439872430474));
#51461=CARTESIAN_POINT('Ctrl Pts',(-3.5201303078758,-1.95597299937839,0.001346970720391));
#51462=CARTESIAN_POINT('Ctrl Pts',(-3.6218696921242,-1.95572226229912,0.00145202421754669));
#51463=CARTESIAN_POINT('Ctrl Pts',(-3.59011611268463,-1.9511072722783,-0.554044556796195));
#51464=CARTESIAN_POINT('Ctrl Pts',(-3.55836253324505,-1.70261318298284,
-1.11315029877843));
#51465=CARTESIAN_POINT('Ctrl Pts',(-3.52660895380548,-1.28426775910331,
-1.47692477696249));
#51466=CARTESIAN_POINT('Ctrl Pts',(-3.48956017217967,-0.796159378032062,
-1.90136200391921));
#51467=CARTESIAN_POINT('Ctrl Pts',(-3.45251139055387,-0.0768277754669797,
-2.05988949172389));
#51468=CARTESIAN_POINT('Ctrl Pts',(-3.41546260892806,0.54447499906108,-1.87994612935844));
#51469=CARTESIAN_POINT('Ctrl Pts',(-3.37841382730225,1.16577777358918,-1.70000276699299));
#51470=CARTESIAN_POINT('Ctrl Pts',(-3.34136504567644,1.68905172008024,-1.18158855445736));
#51471=CARTESIAN_POINT('Ctrl Pts',(-3.30431626405063,1.87478418717573,-0.561991748494958));
#51472=CARTESIAN_POINT('Ctrl Pts',(-3.26726748242482,2.06051665427121,0.0576050574674037));
#51473=CARTESIAN_POINT('Ctrl Pts',(-3.23021870079902,1.90870764197117,0.778384456856518));
#51474=CARTESIAN_POINT('Ctrl Pts',(-3.19316991917321,1.48884308449759,1.2704317154486));
#51475=CARTESIAN_POINT('Ctrl Pts',(-3.1561211375474,1.06897852702399,1.7624789740407));
#51476=CARTESIAN_POINT('Ctrl Pts',(-3.11907235592159,0.381058424376826,
2.02579409183575));
#51477=CARTESIAN_POINT('Ctrl Pts',(-3.08202357429578,-0.260042827644615,
1.93985262371964));
#51478=CARTESIAN_POINT('Ctrl Pts',(-3.04497479266997,-0.901144079666002,
1.85391115560354));
#51479=CARTESIAN_POINT('Ctrl Pts',(-3.00792601104417,-1.49542648106167,
1.41871310157634));
#51480=CARTESIAN_POINT('Ctrl Pts',(-2.97087722941836,-1.77087543119594,
0.833457066032298));
#51481=CARTESIAN_POINT('Ctrl Pts',(-2.95454138365365,-1.89232859019302,
0.575401283629502));
#51482=CARTESIAN_POINT('Ctrl Pts',(-2.93820553788893,-1.95179494190022,
0.288171601355809));
#51483=CARTESIAN_POINT('Ctrl Pts',(-2.92186969212421,-1.95097678997586,
0.000619975964519356));
#51484=CARTESIAN_POINT('Origin',(-14.8,0.,0.));
#51485=CARTESIAN_POINT('',(-2.12013030787579,-1.95317394526965,-0.00174698022608888));
#51486=CARTESIAN_POINT('',(-2.22186969212422,-1.95345029075282,-0.00177409282837831));
#51487=CARTESIAN_POINT('',(-14.8,-1.954,-2.39295984553393E-16));
#51488=CARTESIAN_POINT('Ctrl Pts',(-2.12013030787579,-1.95317394526965,
-0.00174698022608888));
#51489=CARTESIAN_POINT('Ctrl Pts',(-2.14696494118173,-1.94909320466695,
0.469273060468867));
#51490=CARTESIAN_POINT('Ctrl Pts',(-2.17379957448768,-1.77791707428167,
0.942952854675103));
#51491=CARTESIAN_POINT('Ctrl Pts',(-2.20063420779362,-1.4680756635552,1.29437413531823));
#51492=CARTESIAN_POINT('Ctrl Pts',(-2.23768298941942,-1.04029837165924,
1.77955796983428));
#51493=CARTESIAN_POINT('Ctrl Pts',(-2.27473177104523,-0.348204585851633,
2.03169902986245));
#51494=CARTESIAN_POINT('Ctrl Pts',(-2.31178055267104,0.291420955456007,
1.93538741782563));
#51495=CARTESIAN_POINT('Ctrl Pts',(-2.34882933429685,0.931046496763703,
1.83907580578881));
#51496=CARTESIAN_POINT('Ctrl Pts',(-2.38587811592266,1.51820379357145,1.39431152168696));
#51497=CARTESIAN_POINT('Ctrl Pts',(-2.42292689754847,1.78413952649653,0.804671837994208));
#51498=CARTESIAN_POINT('Ctrl Pts',(-2.45997567917427,2.05007525942159,0.215032154301494));
#51499=CARTESIAN_POINT('Ctrl Pts',(-2.49702446080008,1.99478942846401,-0.519482928982077));
#51500=CARTESIAN_POINT('Ctrl Pts',(-2.53407324242589,1.64358744171328,-1.06267159813429));
#51501=CARTESIAN_POINT('Ctrl Pts',(-2.57112202405169,1.29238545496256,-1.6058602672865));
#51502=CARTESIAN_POINT('Ctrl Pts',(-2.6081708056775,0.645267312418673,-1.95772252230736));
#51503=CARTESIAN_POINT('Ctrl Pts',(-2.64521958730331,-0.00156844481900884,
-1.95720416795535));
#51504=CARTESIAN_POINT('Ctrl Pts',(-2.68226836892912,-0.648404202056746,
-1.95668581360334));
#51505=CARTESIAN_POINT('Ctrl Pts',(-2.71931715055492,-1.29495757398828,
-1.60378684987845));
#51506=CARTESIAN_POINT('Ctrl Pts',(-2.75636593218073,-1.6452885186346,-1.06003599126631));
#51507=CARTESIAN_POINT('Ctrl Pts',(-2.77762072407909,-1.84627249158189,
-0.748087505049368));
#51508=CARTESIAN_POINT('Ctrl Pts',(-2.79887551597744,-1.9497611398795,-0.373324168442596));
#51509=CARTESIAN_POINT('Ctrl Pts',(-2.8201303078758,-1.95107804107358,0.000764698408270981));
#51510=CARTESIAN_POINT('Ctrl Pts',(-2.92186969212421,-1.95097678997586,
0.000619975964519356));
#51511=CARTESIAN_POINT('Ctrl Pts',(-2.90115675626312,-1.94993941924049,
-0.363979351138944));
#51512=CARTESIAN_POINT('Ctrl Pts',(-2.88044382040203,-1.85198375439503,
-0.729096260305443));
#51513=CARTESIAN_POINT('Ctrl Pts',(-2.85973088454094,-1.66057985668843,
-1.03591747424635));
#51514=CARTESIAN_POINT('Ctrl Pts',(-2.82268210291513,-1.31821983317378,
-1.58472196191997));
#51515=CARTESIAN_POINT('Ctrl Pts',(-2.78563332128933,-0.676884287271719,
-1.94701692020621));
#51516=CARTESIAN_POINT('Ctrl Pts',(-2.74858453966352,-0.0301249583795292,
-1.95697290765036));
#51517=CARTESIAN_POINT('Ctrl Pts',(-2.71153575803771,0.616634370512606,
-1.9669288950945));
#51518=CARTESIAN_POINT('Ctrl Pts',(-2.6744869764119,1.26881748239483,-1.6245459116965));
#51519=CARTESIAN_POINT('Ctrl Pts',(-2.6374381947861,1.62790749704489,-1.08653930156781));
#51520=CARTESIAN_POINT('Ctrl Pts',(-2.60038941316029,1.98699751169498,-0.548532691439077));
#51521=CARTESIAN_POINT('Ctrl Pts',(-2.56334063153448,2.05299442911292,0.185097545420415));
#51522=CARTESIAN_POINT('Ctrl Pts',(-2.52629184990867,1.79569017693857,0.778554598418215));
#51523=CARTESIAN_POINT('Ctrl Pts',(-2.48924306828286,1.53838592476424,1.372011651416));
#51524=CARTESIAN_POINT('Ctrl Pts',(-2.45219428665705,0.957780502997632,
1.82529552055212));
#51525=CARTESIAN_POINT('Ctrl Pts',(-2.41514550503124,0.319628295127426,
1.93092936949567));
#51526=CARTESIAN_POINT('Ctrl Pts',(-2.37809672340544,-0.31852391274278,
2.03656321843921));
#51527=CARTESIAN_POINT('Ctrl Pts',(-2.34104794177963,-1.01422290671656,
1.79454704719021));
#51528=CARTESIAN_POINT('Ctrl Pts',(-2.30399916015382,-1.4490337452698,1.31565636510377));
#51529=CARTESIAN_POINT('Ctrl Pts',(-2.27662267081062,-1.77032890709691,
0.961789245069641));
#51530=CARTESIAN_POINT('Ctrl Pts',(-2.24924618146742,-1.94917421396601,
0.478584173078087));
#51531=CARTESIAN_POINT('Ctrl Pts',(-2.22186969212422,-1.95345029075282,
-0.00177409282837831));
#51532=CARTESIAN_POINT('Origin',(-14.8,0.,0.));
#51533=CARTESIAN_POINT('',(-1.42013030787581,-1.95716002788236,0.00026938582704918));
#51534=CARTESIAN_POINT('',(-1.52186969212421,-1.95708308893297,0.00044115932539827));
#51535=CARTESIAN_POINT('',(-14.8,-1.954,-2.39295984553393E-16));
#51536=CARTESIAN_POINT('Ctrl Pts',(-1.42013030787581,-1.95716002788236,
0.00026938582704918));
#51537=CARTESIAN_POINT('Ctrl Pts',(-1.42095680313442,-1.95718785457129,
0.0147001219979106));
#51538=CARTESIAN_POINT('Ctrl Pts',(-1.42178329839304,-1.95704207475312,
0.0291302803216468));
#51539=CARTESIAN_POINT('Ctrl Pts',(-1.42260979365165,-1.95672097128892,
0.0435565347292863));
#51540=CARTESIAN_POINT('Ctrl Pts',(-1.45965857527746,-1.94232706884309,
0.690233141347453));
#51541=CARTESIAN_POINT('Ctrl Pts',(-1.49670735690327,-1.57563723982012,
1.32906520577453));
#51542=CARTESIAN_POINT('Ctrl Pts',(-1.53375613852908,-1.02449553657502,
1.66765011296634));
#51543=CARTESIAN_POINT('Ctrl Pts',(-1.57080492015488,-0.4733538333299,2.00623502015817));
#51544=CARTESIAN_POINT('Ctrl Pts',(-1.60785370178069,0.262239744137332,
2.04457277011474));
#51545=CARTESIAN_POINT('Ctrl Pts',(-1.6449024834065,0.845591298174233,1.76511373086623));
#51546=CARTESIAN_POINT('Ctrl Pts',(-1.68195126503231,1.42894285221115,1.48565469161772));
#51547=CARTESIAN_POINT('Ctrl Pts',(-1.71900004665812,1.86005238281769,0.888398863164098));
#51548=CARTESIAN_POINT('Ctrl Pts',(-1.75604882828392,1.94159185503945,0.246722734698324));
#51549=CARTESIAN_POINT('Ctrl Pts',(-1.79309760990973,2.02313132726121,-0.394953393767413));
#51550=CARTESIAN_POINT('Ctrl Pts',(-1.83014639153554,1.75510074109823,-1.08104982224532));
#51551=CARTESIAN_POINT('Ctrl Pts',(-1.86719517316134,1.26018333797668,-1.49752735559181));
#51552=CARTESIAN_POINT('Ctrl Pts',(-1.90424395478715,0.765265934855106,
-1.91400488893831));
#51553=CARTESIAN_POINT('Ctrl Pts',(-1.94129273641296,0.0434617147749864,
-2.06086352715338));
#51554=CARTESIAN_POINT('Ctrl Pts',(-1.97834151803877,-0.574845736284208,
-1.87088297156715));
#51555=CARTESIAN_POINT('Ctrl Pts',(-2.01539029966458,-1.19315318734342,
-1.68090241598091));
#51556=CARTESIAN_POINT('Ctrl Pts',(-2.05243908129039,-1.70796386938168,
-1.15408266659332));
#51557=CARTESIAN_POINT('Ctrl Pts',(-2.08948786291619,-1.88363881140861,
-0.531559487397536));
#51558=CARTESIAN_POINT('Ctrl Pts',(-2.09970201123606,-1.93207144090963,
-0.359933220464345));
#51559=CARTESIAN_POINT('Ctrl Pts',(-2.10991615955593,-1.95472721001136,
-0.181032774909288));
#51560=CARTESIAN_POINT('Ctrl Pts',(-2.12013030787579,-1.95317394526965,
-0.00174698022608888));
#51561=CARTESIAN_POINT('Ctrl Pts',(-2.22186969212422,-1.95345029075282,
-0.00177409282837831));
#51562=CARTESIAN_POINT('Ctrl Pts',(-2.21219739984161,-1.9549610565777,-0.171487801915292));
#51563=CARTESIAN_POINT('Ctrl Pts',(-2.20252510755901,-1.9346811310198,-0.34084615700999));
#51564=CARTESIAN_POINT('Ctrl Pts',(-2.1928528152764,-1.89119399620921,-0.504019590408433));
#51565=CARTESIAN_POINT('Ctrl Pts',(-2.15580403365059,-1.72462072546273,
-1.12903967091033));
#51566=CARTESIAN_POINT('Ctrl Pts',(-2.11875525202478,-1.21755150083708,
-1.66331463899026));
#51567=CARTESIAN_POINT('Ctrl Pts',(-2.08170647039897,-0.602081771860848,
-1.86229644050529));
#51568=CARTESIAN_POINT('Ctrl Pts',(-2.04465768877316,0.013387957115369,
-2.06127824202032));
#51569=CARTESIAN_POINT('Ctrl Pts',(-2.00760890714736,0.737258190442158,
-1.92496687697051));
#51570=CARTESIAN_POINT('Ctrl Pts',(-1.97056012552155,1.23819948608823,-1.51575474619958));
#51571=CARTESIAN_POINT('Ctrl Pts',(-1.93351134389574,1.73914078173428,-1.10654261542867));
#51572=CARTESIAN_POINT('Ctrl Pts',(-1.89646256226994,2.01715313969961,-0.424429718936621));
#51573=CARTESIAN_POINT('Ctrl Pts',(-1.85941378064413,1.944984851277,0.218367696264819));
#51574=CARTESIAN_POINT('Ctrl Pts',(-1.82236499901832,1.87281656285439,0.861165111466315));
#51575=CARTESIAN_POINT('Ctrl Pts',(-1.78531621739251,1.45046762804381,1.46464704537719));
#51576=CARTESIAN_POINT('Ctrl Pts',(-1.7482674357667,0.871255457195034,1.75258794478866));
#51577=CARTESIAN_POINT('Ctrl Pts',(-1.71121865414089,0.29204328634627,2.04052884420011));
#51578=CARTESIAN_POINT('Ctrl Pts',(-1.67416987251508,-0.444032120540709,
2.01292870911214));
#51579=CARTESIAN_POINT('Ctrl Pts',(-1.63712109088927,-1.00005493501247,
1.68242093857152));
#51580=CARTESIAN_POINT('Ctrl Pts',(-1.60007230926347,-1.55607774948418,
1.35191316803094));
#51581=CARTESIAN_POINT('Ctrl Pts',(-1.56302352763766,-1.93204797154073,
0.718497762037816));
#51582=CARTESIAN_POINT('Ctrl Pts',(-1.52597474601186,-1.95587637322525,
0.0721007232658861));
#51583=CARTESIAN_POINT('Ctrl Pts',(-1.52460639471597,-1.95675644600748,
0.048226841673994));
#51584=CARTESIAN_POINT('Ctrl Pts',(-1.52323804342009,-1.95715616086527,
0.0243352517901117));
#51585=CARTESIAN_POINT('Ctrl Pts',(-1.52186969212421,-1.95708308893297,
0.00044115932539827));
#51586=CARTESIAN_POINT('Origin',(-14.8,0.,0.));
#51587=CARTESIAN_POINT('',(-0.720130307875805,-1.95236950710743,0.00155959742907545));
#51588=CARTESIAN_POINT('',(-0.821869692124218,-1.95215209727744,0.00149476428280041));
#51589=CARTESIAN_POINT('',(-14.8,-1.954,-2.39295984553393E-16));
#51590=CARTESIAN_POINT('Ctrl Pts',(-0.720130307875805,-1.95236950710743,
0.00155959742907545));
#51591=CARTESIAN_POINT('Ctrl Pts',(-0.731997446712908,-1.95397811762504,
0.210098641876465));
#51592=CARTESIAN_POINT('Ctrl Pts',(-0.74386458555001,-1.9232378714622,0.418181660990822));
#51593=CARTESIAN_POINT('Ctrl Pts',(-0.755731724387113,-1.85816191132805,
0.61489403534867));
#51594=CARTESIAN_POINT('Ctrl Pts',(-0.79278050601292,-1.65499709888296,
1.22902300954524));
#51595=CARTESIAN_POINT('Ctrl Pts',(-0.829829287638726,-1.11717375820457,
1.73232617588306));
#51596=CARTESIAN_POINT('Ctrl Pts',(-0.866878069264533,-0.491005984724849,
1.89458512275237));
#51597=CARTESIAN_POINT('Ctrl Pts',(-0.90392685089034,0.135161788754873,
2.05684406962167));
#51598=CARTESIAN_POINT('Ctrl Pts',(-0.940975632516148,0.849673995035926,
1.87805879702246));
#51599=CARTESIAN_POINT('Ctrl Pts',(-0.978024414141956,1.32555909087577,
1.43998228306123));
#51600=CARTESIAN_POINT('Ctrl Pts',(-1.01507319576777,1.80144418671564,1.00190576909997));
#51601=CARTESIAN_POINT('Ctrl Pts',(-1.05212197739358,2.03870217211428,0.304538013776658));
#51602=CARTESIAN_POINT('Ctrl Pts',(-1.08917075901938,1.92869625712718,-0.332879891399014));
#51603=CARTESIAN_POINT('Ctrl Pts',(-1.12621954064519,1.81869034214009,-0.97029779657465));
#51604=CARTESIAN_POINT('Ctrl Pts',(-1.163268322271,1.36142052676731,-1.54776585160265));
#51605=CARTESIAN_POINT('Ctrl Pts',(-1.2003171038968,0.766208696269818,-1.8009879562628));
#51606=CARTESIAN_POINT('Ctrl Pts',(-1.23736588552261,0.170996865772328,
-2.05421006092295));
#51607=CARTESIAN_POINT('Ctrl Pts',(-1.27441466714842,-0.562156979849869,
-1.98318621521523));
#51608=CARTESIAN_POINT('Ctrl Pts',(-1.31146344877423,-1.09768491472663,
-1.62041371795675));
#51609=CARTESIAN_POINT('Ctrl Pts',(-1.34768573514142,-1.62126613288,-1.26573405764948));
#51610=CARTESIAN_POINT('Ctrl Pts',(-1.38390802150861,-1.95594048513913,
-0.632177385793262));
#51611=CARTESIAN_POINT('Ctrl Pts',(-1.42013030787581,-1.95716002788236,
0.00026938582704918));
#51612=CARTESIAN_POINT('Ctrl Pts',(-1.52186969212421,-1.95708308893297,
0.00044115932539827));
#51613=CARTESIAN_POINT('Ctrl Pts',(-1.48618926179428,-1.95517770250362,
-0.622609006263858));
#51614=CARTESIAN_POINT('Ctrl Pts',(-1.45050883146436,-1.63180984023605,
-1.24736075456756));
#51615=CARTESIAN_POINT('Ctrl Pts',(-1.41482840113443,-1.12121221885139,
-1.60422384641027));
#51616=CARTESIAN_POINT('Ctrl Pts',(-1.37777961950862,-0.591033081480647,
-1.97477270576364));
#51617=CARTESIAN_POINT('Ctrl Pts',(-1.34073083788282,0.141011774573193,
-2.05649175291963));
#51618=CARTESIAN_POINT('Ctrl Pts',(-1.30368205625701,0.739852474057205,
-1.81197852634512));
#51619=CARTESIAN_POINT('Ctrl Pts',(-1.2666332746312,1.3386931735412,-1.56746529977062));
#51620=CARTESIAN_POINT('Ctrl Pts',(-1.2295844930054,1.80432971645534,-0.996719799465619));
#51621=CARTESIAN_POINT('Ctrl Pts',(-1.19253571137959,1.92362878104123,-0.360979650549547));
#51622=CARTESIAN_POINT('Ctrl Pts',(-1.15548692975378,2.04292784562714,0.274760498366579));
#51623=CARTESIAN_POINT('Ctrl Pts',(-1.11843814812797,1.81588943188477,0.975495295893765));
#51624=CARTESIAN_POINT('Ctrl Pts',(-1.08138936650216,1.34643805442864,1.42047781403675));
#51625=CARTESIAN_POINT('Ctrl Pts',(-1.04434058487635,0.87698667697254,1.8654603321797));
#51626=CARTESIAN_POINT('Ctrl Pts',(-1.00729180325054,0.165122335802693,
2.05469057093846));
#51627=CARTESIAN_POINT('Ctrl Pts',(-0.970243021624738,-0.463329621498074,
1.90156748386759));
#51628=CARTESIAN_POINT('Ctrl Pts',(-0.933194239998929,-1.09178157879888,
1.7484443967967));
#51629=CARTESIAN_POINT('Ctrl Pts',(-0.896145458373119,-1.63682115223063,
1.25296798389613));
#51630=CARTESIAN_POINT('Ctrl Pts',(-0.85909667674731,-1.84895641765906,
0.641902107360681));
#51631=CARTESIAN_POINT('Ctrl Pts',(-0.846687681872946,-1.92000829320952,
0.437233748589477));
#51632=CARTESIAN_POINT('Ctrl Pts',(-0.834278686998582,-1.95371411099365,
0.219598267788578));
#51633=CARTESIAN_POINT('Ctrl Pts',(-0.821869692124218,-1.95215209727744,
0.00149476428280041));
#51634=CARTESIAN_POINT('Origin',(-30.9400562256037,0.,0.));
#51635=CARTESIAN_POINT('',(-0.490056225603759,-1.55420203086265,0.00124153214009217));
#51636=CARTESIAN_POINT('',(-0.351943774396335,-1.55328744883452,-0.00161118505867947));
#51637=CARTESIAN_POINT('',(-30.9400562256037,-1.5555,7.38654183493349E-13));
#51638=CARTESIAN_POINT('',(-0.199999999999997,1.3381997242603,-0.79799174809645));
#51639=CARTESIAN_POINT('Ctrl Pts',(-0.490056225603758,-1.55420203086265,
0.00124153214009213));
#51640=CARTESIAN_POINT('Ctrl Pts',(-0.464874582815045,-1.55148475084143,
-0.351024583825932));
#51641=CARTESIAN_POINT('Ctrl Pts',(-0.402644158400524,-1.25822046322886,
-1.2256057899134));
#51642=CARTESIAN_POINT('Ctrl Pts',(-0.305958749865941,0.154235008178209,
-1.81221901823593));
#51643=CARTESIAN_POINT('Ctrl Pts',(-0.234454984120064,1.09063722427217,
-1.20829039445635));
#51644=CARTESIAN_POINT('Ctrl Pts',(-0.199999999999997,1.33821259954898,
-0.797996165556926));
#51645=CARTESIAN_POINT('',(-0.199999999999996,-0.319621170202251,-1.52230829911636));
#51646=CARTESIAN_POINT('Origin',(-0.2,0.,0.));
#51647=CARTESIAN_POINT('Ctrl Pts',(-0.351943774396335,-1.55328744883452,
-0.00161118505867953));
#51648=CARTESIAN_POINT('Ctrl Pts',(-0.338344631223361,-1.5543673293507,
-0.192088933053909));
#51649=CARTESIAN_POINT('Ctrl Pts',(-0.287696706424579,-1.4337686830043,
-0.899654195900291));
#51650=CARTESIAN_POINT('Ctrl Pts',(-0.237048781625798,-0.82586340403187,
-1.41601857102626));
#51651=CARTESIAN_POINT('Ctrl Pts',(-0.199999999999991,-0.319621170202164,
-1.52230829911638));
#51652=CARTESIAN_POINT('Origin',(-30.9400562256037,0.,0.));
#51653=CARTESIAN_POINT('',(-1.19005622560375,-1.55801556979069,0.000214447110768814));
#51654=CARTESIAN_POINT('',(-1.05194377439633,-1.55402895973136,0.00118992110716552));
#51655=CARTESIAN_POINT('',(-30.9400562256037,-1.5555,7.38654183493349E-13));
#51656=CARTESIAN_POINT('Ctrl Pts',(-1.19005622560375,-1.55801556979069,
0.000214447110768934));
#51657=CARTESIAN_POINT('Ctrl Pts',(-1.15383393923655,-1.55704474136851,
-0.503250728557323));
#51658=CARTESIAN_POINT('Ctrl Pts',(-1.08056287124355,-1.01812443290281,
-1.52345605568379));
#51659=CARTESIAN_POINT('Ctrl Pts',(-0.970243021624738,0.719757641542406,
-1.69181235504817));
#51660=CARTESIAN_POINT('Ctrl Pts',(-0.859096676747318,1.81179939867516,
-0.312715794767707));
#51661=CARTESIAN_POINT('Ctrl Pts',(-0.747950331869893,1.24518507479472,
1.35272260350057));
#51662=CARTESIAN_POINT('Ctrl Pts',(-0.636803986992467,-0.461197325722433,
1.77969367544763));
#51663=CARTESIAN_POINT('Ctrl Pts',(-0.550839284903758,-1.45461374558017,
0.850039657502599));
#51664=CARTESIAN_POINT('Ctrl Pts',(-0.501923364440855,-1.55548258033043,
0.167250991524811));
#51665=CARTESIAN_POINT('Ctrl Pts',(-0.490056225603758,-1.55420203086265,
0.00124153214009213));
#51666=CARTESIAN_POINT('Ctrl Pts',(-1.05194377439633,-1.55402895973136,
0.00118992110716549));
#51667=CARTESIAN_POINT('Ctrl Pts',(-1.02730398764487,-1.55155990544438,
-0.343563383414919));
#51668=CARTESIAN_POINT('Ctrl Pts',(-0.965615419267606,-1.26824253586962,
-1.21037106719846));
#51669=CARTESIAN_POINT('Ctrl Pts',(-0.866878069264529,0.165833894051307,
-1.83098644971143));
#51670=CARTESIAN_POINT('Ctrl Pts',(-0.755731724387107,1.62851911260145,
-0.853729469588644));
#51671=CARTESIAN_POINT('Ctrl Pts',(-0.644585379509683,1.60003419765428,
0.9056105153729));
#51672=CARTESIAN_POINT('Ctrl Pts',(-0.533439034632261,0.107502597833407,
1.83487847835014));
#51673=CARTESIAN_POINT('Ctrl Pts',(-0.435891832927811,-1.28993868652504,
1.17800533567591));
#51674=CARTESIAN_POINT('Ctrl Pts',(-0.375393412849168,-1.55142536036654,
0.326838502321218));
#51675=CARTESIAN_POINT('Ctrl Pts',(-0.351943774396335,-1.55328744883452,
-0.00161118505867953));
#51676=CARTESIAN_POINT('Origin',(-30.9400562256037,0.,0.));
#51677=CARTESIAN_POINT('',(-1.89005622560376,-1.55484241139557,-0.00139069996956104));
#51678=CARTESIAN_POINT('',(-1.75194377439633,-1.55795432181946,0.000351189013561961));
#51679=CARTESIAN_POINT('',(-30.9400562256037,-1.5555,7.38654183493349E-13));
#51680=CARTESIAN_POINT('Ctrl Pts',(-1.89005622560376,-1.55484241139557,
-0.00139069996956129));
#51681=CARTESIAN_POINT('Ctrl Pts',(-1.87984207728388,-1.55607890234021,
-0.144112835911223));
#51682=CARTESIAN_POINT('Ctrl Pts',(-1.8325791473382,-1.47262574984037,-0.803097578304466));
#51683=CARTESIAN_POINT('Ctrl Pts',(-1.74826743576671,-0.540000904300196,
-1.75747790595217));
#51684=CARTESIAN_POINT('Ctrl Pts',(-1.63712109088928,1.1837961238493,-1.40675332292743));
#51685=CARTESIAN_POINT('Ctrl Pts',(-1.52597474601186,1.82390089883899,0.231767139453362));
#51686=CARTESIAN_POINT('Ctrl Pts',(-1.41482840113443,0.794334560776014,
1.65812042680182));
#51687=CARTESIAN_POINT('Ctrl Pts',(-1.30368205625701,-0.962393908646208,
1.56656305209763));
#51688=CARTESIAN_POINT('Ctrl Pts',(-1.22875799774678,-1.55271959931364,
0.538121710656146));
#51689=CARTESIAN_POINT('Ctrl Pts',(-1.19088272086236,-1.55803772148702,
0.0117021697892325));
#51690=CARTESIAN_POINT('Ctrl Pts',(-1.19005622560375,-1.55801556979069,
0.000214447110768934));
#51691=CARTESIAN_POINT('Ctrl Pts',(-1.75194377439633,-1.55795432181946,
0.000351189013562063));
#51692=CARTESIAN_POINT('Ctrl Pts',(-1.71626334406638,-1.55643752110799,
-0.495633730420732));
#51693=CARTESIAN_POINT('Ctrl Pts',(-1.64353413211064,-1.03172538405955,
-1.50938575475204));
#51694=CARTESIAN_POINT('Ctrl Pts',(-1.53375613852907,0.695004907338835,
-1.70214273260888));
#51695=CARTESIAN_POINT('Ctrl Pts',(-1.42260979365165,1.80702789992282,-0.339100830268501));
#51696=CARTESIAN_POINT('Ctrl Pts',(-1.31146344877422,1.26481973322455,1.33437866444013));
#51697=CARTESIAN_POINT('Ctrl Pts',(-1.2003171038968,-0.43523909383229,1.78629417578513));
#51698=CARTESIAN_POINT('Ctrl Pts',(-1.11381054577083,-1.44833041407964,
0.865328290434377));
#51699=CARTESIAN_POINT('Ctrl Pts',(-1.06435276927068,-1.55527241537895,
0.174813257700223));
#51700=CARTESIAN_POINT('Ctrl Pts',(-1.05194377439633,-1.55402895973136,
0.00118992110716549));
#51701=CARTESIAN_POINT('Origin',(-30.9400562256037,0.,0.));
#51702=CARTESIAN_POINT('',(-2.59005622560375,-1.5531739472313,0.00060874532998613));
#51703=CARTESIAN_POINT('',(-2.45194377439633,-1.55506239880552,-0.00141228321026893));
#51704=CARTESIAN_POINT('',(-30.9400562256037,-1.5555,7.38654183493349E-13));
#51705=CARTESIAN_POINT('Ctrl Pts',(-2.59005622560375,-1.5531739472313,0.000608745329986182));
#51706=CARTESIAN_POINT('Ctrl Pts',(-2.56880143370539,-1.5521256157025,-0.297188200620199));
#51707=CARTESIAN_POINT('Ctrl Pts',(-2.51049786018122,-1.32614224219593,
-1.11554156078284));
#51708=CARTESIAN_POINT('Ctrl Pts',(-2.41514550503125,-0.00147337065513613,
-1.83856659218734));
#51709=CARTESIAN_POINT('Ctrl Pts',(-2.30399916015382,1.54396000303022,-0.998256861862604));
#51710=CARTESIAN_POINT('Ctrl Pts',(-2.1928528152764,1.67599241355422,0.755895971373255));
#51711=CARTESIAN_POINT('Ctrl Pts',(-2.08170647039897,0.273756218286524,
1.81807229264321));
#51712=CARTESIAN_POINT('Ctrl Pts',(-1.98077427384143,-1.22719369529558,
1.27125174603469));
#51713=CARTESIAN_POINT('Ctrl Pts',(-1.91689085890969,-1.55159389962086,
0.373569214718623));
#51714=CARTESIAN_POINT('Ctrl Pts',(-1.89005622560376,-1.55484241139557,
-0.00139069996956129));
#51715=CARTESIAN_POINT('Ctrl Pts',(-2.45194377439633,-1.55506239880552,
-0.00141228321026872));
#51716=CARTESIAN_POINT('Ctrl Pts',(-2.44227148211371,-1.55626505808943,
-0.136514470766642));
#51717=CARTESIAN_POINT('Ctrl Pts',(-2.39555040820528,-1.4782829057982,-0.78774610379817));
#51718=CARTESIAN_POINT('Ctrl Pts',(-2.31178055267104,-0.565586069932105,
-1.74941178802327));
#51719=CARTESIAN_POINT('Ctrl Pts',(-2.20063420779361,1.16314496579956,-1.42387597174662));
#51720=CARTESIAN_POINT('Ctrl Pts',(-2.08948786291619,1.82708798956902,0.205131106799974));
#51721=CARTESIAN_POINT('Ctrl Pts',(-1.97834151803877,0.818443514495715,
1.64635344282621));
#51722=CARTESIAN_POINT('Ctrl Pts',(-1.86719517316135,-0.939435649392642,
1.58043940475681));
#51723=CARTESIAN_POINT('Ctrl Pts',(-1.79172925861386,-1.54907896162025,
0.55334352462763));
#51724=CARTESIAN_POINT('Ctrl Pts',(-1.75331212569219,-1.55801249141551,
0.0193723050976691));
#51725=CARTESIAN_POINT('Ctrl Pts',(-1.75194377439633,-1.55795432181946,
0.000351189013562063));
#51726=CARTESIAN_POINT('Origin',(-30.9400562256037,0.,0.));
#51727=CARTESIAN_POINT('',(-3.29005622560375,-1.55707062463311,0.00107226865735175));
#51728=CARTESIAN_POINT('',(-3.15194377439632,-1.5530933453467,0.000493537673696837));
#51729=CARTESIAN_POINT('',(-30.9400562256037,-1.5555,7.38654183493349E-13));
#51730=CARTESIAN_POINT('Ctrl Pts',(-3.29005622560375,-1.55707062463311,
0.00107226865735168));
#51731=CARTESIAN_POINT('Ctrl Pts',(-3.25776079012691,-1.55353014804423,
-0.448531587290127));
#51732=CARTESIAN_POINT('Ctrl Pts',(-3.18841657302425,-1.11235272993948,
-1.41997182206607));
#51733=CARTESIAN_POINT('Ctrl Pts',(-3.08202357429579,0.537183538203758,
-1.75834101421655));
#51734=CARTESIAN_POINT('Ctrl Pts',(-2.97087722941836,1.76865785992407,-0.502173923924951));
#51735=CARTESIAN_POINT('Ctrl Pts',(-2.85973088454094,1.38103405472633,1.21370268825252));
#51736=CARTESIAN_POINT('Ctrl Pts',(-2.74858453966351,-0.27084198568111,
1.81850870111212));
#51737=CARTESIAN_POINT('Ctrl Pts',(-2.65869298668446,-1.4063004296344,0.961273762251427));
#51738=CARTESIAN_POINT('Ctrl Pts',(-2.6058502153312,-1.55395294038616,0.221895405189746));
#51739=CARTESIAN_POINT('Ctrl Pts',(-2.59005622560375,-1.5531739472313,0.000608745329986182));
#51740=CARTESIAN_POINT('Ctrl Pts',(-3.15194377439632,-1.5530933453467,0.000493537673696715));
#51741=CARTESIAN_POINT('Ctrl Pts',(-3.13123083853522,-1.55226753665755,
-0.289749171287345));
#51742=CARTESIAN_POINT('Ctrl Pts',(-3.0734691210483,-1.33481050756564,-1.1002917617943));
#51743=CARTESIAN_POINT('Ctrl Pts',(-2.97865862193558,-0.0282989084957232,
-1.83834934851334));
#51744=CARTESIAN_POINT('Ctrl Pts',(-2.86751227705816,1.52923051402139,-1.02067780704635));
#51745=CARTESIAN_POINT('Ctrl Pts',(-2.75636593218073,1.6868429066166,0.731361855340862));
#51746=CARTESIAN_POINT('Ctrl Pts',(-2.64521958730331,0.300253755811285,
1.81388446297849));
#51747=CARTESIAN_POINT('Ctrl Pts',(-2.54374553470851,-1.21661465163989,
1.28620411926705));
#51748=CARTESIAN_POINT('Ctrl Pts',(-2.47932026373952,-1.55165838783199,
0.380981413113712));
#51749=CARTESIAN_POINT('Ctrl Pts',(-2.45194377439633,-1.55506239880552,
-0.00141228321026872));
#51750=CARTESIAN_POINT('Origin',(-30.9400562256037,0.,0.));
#51751=CARTESIAN_POINT('',(-3.99005622560375,-1.55648113771292,-0.00128084310329906));
#51752=CARTESIAN_POINT('',(-3.85194377439632,-1.5568710230329,0.00115589747807187));
#51753=CARTESIAN_POINT('',(-30.9400562256037,-1.5555,7.38654183493349E-13));
#51754=CARTESIAN_POINT('Ctrl Pts',(-3.99005622560375,-1.55648113771292,
-0.00128084310329882));
#51755=CARTESIAN_POINT('Ctrl Pts',(-3.98376892817423,-1.55725912360882,
-0.0888962976159076));
#51756=CARTESIAN_POINT('Ctrl Pts',(-3.9404328491189,-1.51066019062247,-0.691970511541442));
#51757=CARTESIAN_POINT('Ctrl Pts',(-3.86004798843775,-0.72247792391575,
-1.69066700601096));
#51758=CARTESIAN_POINT('Ctrl Pts',(-3.74890164356033,1.02870839145545,-1.52383999196612));
#51759=CARTESIAN_POINT('Ctrl Pts',(-3.63775529868291,1.83817507420302,0.0379693604454949));
#51760=CARTESIAN_POINT('Ctrl Pts',(-3.52660895380548,0.964904870636465,
1.56502008497577));
#51761=CARTESIAN_POINT('Ctrl Pts',(-3.41546260892806,-0.791676743481206,
1.65939061393862));
#51762=CARTESIAN_POINT('Ctrl Pts',(-3.33661169952748,-1.52370538518956,
0.648661022529862));
#51763=CARTESIAN_POINT('Ctrl Pts',(-3.29480957175271,-1.55759172337387,
0.0672464114013962));
#51764=CARTESIAN_POINT('Ctrl Pts',(-3.29005622560375,-1.55707062463311,
0.00107226865735168));
#51765=CARTESIAN_POINT('Ctrl Pts',(-3.85194377439632,-1.5568710230329,0.0011558974780719));
#51766=CARTESIAN_POINT('Ctrl Pts',(-3.82019019495673,-1.55319721700584,
-0.441052358288231));
#51767=CARTESIAN_POINT('Ctrl Pts',(-3.75138783389134,-1.12457747294624,
-1.40543650404529));
#51768=CARTESIAN_POINT('Ctrl Pts',(-3.64553669120012,0.511471188869394,
-1.7659916129257));
#51769=CARTESIAN_POINT('Ctrl Pts',(-3.5343903463227,1.76114256619831,-0.527926145782834));
#51770=CARTESIAN_POINT('Ctrl Pts',(-3.42324400144528,1.3985956082158,1.19342342803983));
#51771=CARTESIAN_POINT('Ctrl Pts',(-3.31209765656785,-0.244280112870538,
1.82226682475983));
#51772=CARTESIAN_POINT('Ctrl Pts',(-3.22166424755154,-1.39904427633039,
0.976623212198346));
#51773=CARTESIAN_POINT('Ctrl Pts',(-3.16827962016103,-1.55374464284829,
0.229401702103439));
#51774=CARTESIAN_POINT('Ctrl Pts',(-3.15194377439632,-1.5530933453467,0.000493537673696715));
#51775=CARTESIAN_POINT('Origin',(-30.9400562256037,0.,0.));
#51776=CARTESIAN_POINT('',(-4.69005622560375,-1.55299085045476,-0.000273689629153198));
#51777=CARTESIAN_POINT('',(-4.55194377439633,-1.55669747240667,-0.00121723354483211));
#51778=CARTESIAN_POINT('',(-30.9400562256037,-1.5555,7.38654183493349E-13));
#51779=CARTESIAN_POINT('Ctrl Pts',(-4.69005622560374,-1.55299085045476,
-0.000273689629153306));
#51780=CARTESIAN_POINT('Ctrl Pts',(-4.67272828459573,-1.55337253579367,
-0.243123736094311));
#51781=CARTESIAN_POINT('Ctrl Pts',(-4.61835156196192,-1.38536919465911,
-1.00471048981168));
#51782=CARTESIAN_POINT('Ctrl Pts',(-4.52692605770229,-0.195516740427347,
-1.82814181068467));
#51783=CARTESIAN_POINT('Ctrl Pts',(-4.41577971282487,1.42997518601849,-1.15563845692861));
#51784=CARTESIAN_POINT('Ctrl Pts',(-4.30463336794744,1.74641226463907,0.57478124332561));
#51785=CARTESIAN_POINT('Ctrl Pts',(-4.19348702307002,0.464115698312818,
1.77902385996933));
#51786=CARTESIAN_POINT('Ctrl Pts',(-4.08862797562212,-1.14647988477387,
1.37868314453131));
#51787=CARTESIAN_POINT('Ctrl Pts',(-4.02081770980003,-1.55267473263827,
0.42739005238893));
#51788=CARTESIAN_POINT('Ctrl Pts',(-3.99005622560375,-1.55648113771292,
-0.00128084310329882));
#51789=CARTESIAN_POINT('Ctrl Pts',(-4.55194377439633,-1.55669747240667,
-0.00121723354483209));
#51790=CARTESIAN_POINT('Ctrl Pts',(-4.54619833300405,-1.55738594741117,
-0.0812528916058229));
#51791=CARTESIAN_POINT('Ctrl Pts',(-4.50340410998597,-1.51538141740202,
-0.676664269333276));
#51792=CARTESIAN_POINT('Ctrl Pts',(-4.42356110534208,-0.747068761626052,
-1.67994565963717));
#51793=CARTESIAN_POINT('Ctrl Pts',(-4.31241476046467,1.00636520985961,-1.53868717363749));
#51794=CARTESIAN_POINT('Ctrl Pts',(-4.20126841558724,1.83853336531533,0.0111453377239352));
#51795=CARTESIAN_POINT('Ctrl Pts',(-4.09012207070981,0.987636640845155,
1.55077497387288));
#51796=CARTESIAN_POINT('Ctrl Pts',(-3.9789757258324,-0.767381039870437,
1.6707649426488));
#51797=CARTESIAN_POINT('Ctrl Pts',(-3.89958296039456,-1.5192100806146,0.663952155285627));
#51798=CARTESIAN_POINT('Ctrl Pts',(-3.85723897658254,-1.55748366406581,
0.0748982019370303));
#51799=CARTESIAN_POINT('Ctrl Pts',(-3.85194377439632,-1.5568710230329,0.0011558974780719));
#51800=CARTESIAN_POINT('Origin',(-30.9400562256037,0.,0.));
#51801=CARTESIAN_POINT('',(-5.39005622560374,-1.55547679241997,0.00142175542085012));
#51802=CARTESIAN_POINT('',(-5.25194377439632,-1.55303950936921,-0.000394967004932745));
#51803=CARTESIAN_POINT('',(-30.9400562256037,-1.5555,7.38654183493349E-13));
#51804=CARTESIAN_POINT('Ctrl Pts',(-5.39005622560374,-1.55547679241997,
0.00142175542085003));
#51805=CARTESIAN_POINT('Ctrl Pts',(-5.36168764101725,-1.55184256103128,
-0.394560312382684));
#51806=CARTESIAN_POINT('Ctrl Pts',(-5.29627027480494,-1.19678629005817,
-1.31348222412533));
#51807=CARTESIAN_POINT('Ctrl Pts',(-5.19380412696683,0.348598926865315,
-1.80521690218908));
#51808=CARTESIAN_POINT('Ctrl Pts',(-5.08265778208941,1.70577709140633,-0.686042119839725));
#51809=CARTESIAN_POINT('Ctrl Pts',(-4.97151143721198,1.50142062748163,1.06116227558912));
#51810=CARTESIAN_POINT('Ctrl Pts',(-4.86036509233456,-0.0773946174390751,
1.83693749184676));
#51811=CARTESIAN_POINT('Ctrl Pts',(-4.76654668846515,-1.35026498281733,
1.072329293764));
#51812=CARTESIAN_POINT('Ctrl Pts',(-4.70977706622154,-1.55255645633192,
0.276112700314716));
#51813=CARTESIAN_POINT('Ctrl Pts',(-4.69005622560374,-1.55299085045476,
-0.000273689629153306));
#51814=CARTESIAN_POINT('Ctrl Pts',(-5.25194377439632,-1.55303950936921,
-0.000394967004932641));
#51815=CARTESIAN_POINT('Ctrl Pts',(-5.23515768942556,-1.55357404340117,
-0.235632524798968));
#51816=CARTESIAN_POINT('Ctrl Pts',(-5.181322822829,-1.39290097570194,-0.989372871163793));
#51817=CARTESIAN_POINT('Ctrl Pts',(-5.09043917460663,-0.22216951407526,
-1.82509448000564));
#51818=CARTESIAN_POINT('Ctrl Pts',(-4.9792928297292,1.4129615451609,-1.17637954157153));
#51819=CARTESIAN_POINT('Ctrl Pts',(-4.86814648485178,1.75461270448817,0.549238938150095));
#51820=CARTESIAN_POINT('Ctrl Pts',(-4.75700013997435,0.490023217597568,
1.7720627528806));
#51821=CARTESIAN_POINT('Ctrl Pts',(-4.65159923648921,-1.13459408569634,
1.39331703519712));
#51822=CARTESIAN_POINT('Ctrl Pts',(-4.58324711462986,-1.55294639988908,
0.434847337311016));
#51823=CARTESIAN_POINT('Ctrl Pts',(-4.55194377439633,-1.55669747240667,
-0.00121723354483209));
#51824=CARTESIAN_POINT('Origin',(-30.9400562256037,0.,0.));
#51825=CARTESIAN_POINT('',(-6.09005622560374,-1.55777658619528,-0.000591325705981328));
#51826=CARTESIAN_POINT('',(-5.95194377439632,-1.5552490056676,0.00142145573523295));
#51827=CARTESIAN_POINT('',(-30.9400562256037,-1.5555,7.38654183493349E-13));
#51828=CARTESIAN_POINT('Ctrl Pts',(-6.09005622560374,-1.55777658619529,
-0.00059132570598132));
#51829=CARTESIAN_POINT('Ctrl Pts',(-6.08769577906457,-1.55793621982475,
-0.0334132884585462));
#51830=CARTESIAN_POINT('Ctrl Pts',(-6.04828655089958,-1.54211757398053,
-0.581241099247826));
#51831=CARTESIAN_POINT('Ctrl Pts',(-5.9718285411088,-0.896884068407809,
-1.60496985753535));
#51832=CARTESIAN_POINT('Ctrl Pts',(-5.86068219623137,0.862128800674478,
-1.62390369382189));
#51833=CARTESIAN_POINT('Ctrl Pts',(-5.74953585135396,1.83191546708753,-0.156252991031506));
#51834=CARTESIAN_POINT('Ctrl Pts',(-5.63838950647652,1.12469553475403,1.45443777105284));
#51835=CARTESIAN_POINT('Ctrl Pts',(-5.5272431615991,-0.612114390813121,
1.73367968446316));
#51836=CARTESIAN_POINT('Ctrl Pts',(-5.44446540130818,-1.4882965528505,0.759651063044836));
#51837=CARTESIAN_POINT('Ctrl Pts',(-5.39873642264305,-1.55658879166139,
0.122584034846145));
#51838=CARTESIAN_POINT('Ctrl Pts',(-5.39005622560374,-1.55547679241997,
0.00142175542085003));
#51839=CARTESIAN_POINT('Ctrl Pts',(-5.95194377439632,-1.5552490056676,0.0014214557352331));
#51840=CARTESIAN_POINT('Ctrl Pts',(-5.92411704584707,-1.55173109412698,
-0.387142374296427));
#51841=CARTESIAN_POINT('Ctrl Pts',(-5.85924153567202,-1.20768988464287,
-1.2985999419321));
#51842=CARTESIAN_POINT('Ctrl Pts',(-5.75731724387117,0.322222710510533,
-1.81011095758319));
#51843=CARTESIAN_POINT('Ctrl Pts',(-5.64617089899375,1.69558575464707,-0.710857301129708));
#51844=CARTESIAN_POINT('Ctrl Pts',(-5.53502455411632,1.51674371597785,1.03914274956487));
#51845=CARTESIAN_POINT('Ctrl Pts',(-5.4238782092389,-0.0505844542846405,
1.83787115079273));
#51846=CARTESIAN_POINT('Ctrl Pts',(-5.32951794933223,-1.34189057390848,
1.08760790747833));
#51847=CARTESIAN_POINT('Ctrl Pts',(-5.27220647105137,-1.55239426654098,
0.283563280779469));
#51848=CARTESIAN_POINT('Ctrl Pts',(-5.25194377439632,-1.55303950936921,
-0.000394967004932641));
#51849=CARTESIAN_POINT('Origin',(-30.9400562256037,0.,0.));
#51850=CARTESIAN_POINT('',(-6.79005622560374,-1.55372215258713,-0.00105166811141202));
#51851=CARTESIAN_POINT('',(-6.65194377439632,-1.55788369592683,-0.000462245611997092));
#51852=CARTESIAN_POINT('',(-30.9400562256037,-1.5555,7.38654183493349E-13));
#51853=CARTESIAN_POINT('Ctrl Pts',(-6.79005622560374,-1.55372215258713,
-0.00105166811141207));
#51854=CARTESIAN_POINT('Ctrl Pts',(-6.77665513548608,-1.55488854693699,
-0.188645944060803));
#51855=CARTESIAN_POINT('Ctrl Pts',(-6.72620526374262,-1.4365859816325,-0.89344377020468));
#51856=CARTESIAN_POINT('Ctrl Pts',(-6.63870661037334,-0.387375999329962,
-1.79729494265797));
#51857=CARTESIAN_POINT('Ctrl Pts',(-6.5275602654959,1.30001617698454,-1.30011046274511));
#51858=CARTESIAN_POINT('Ctrl Pts',(-6.4164139206185,1.79732303197884,0.387245651336726));
#51859=CARTESIAN_POINT('Ctrl Pts',(-6.30526757574106,0.649290547434899,
1.72010204952278));
#51860=CARTESIAN_POINT('Ctrl Pts',(-6.19648167740282,-1.05612350019664,
1.48344519834433));
#51861=CARTESIAN_POINT('Ctrl Pts',(-6.12474456069037,-1.55543066361753,
0.481749292167505));
#51862=CARTESIAN_POINT('Ctrl Pts',(-6.09005622560374,-1.55777658619529,
-0.00059132570598132));
#51863=CARTESIAN_POINT('Ctrl Pts',(-6.65194377439632,-1.55788369592683,
-0.000462245611997049));
#51864=CARTESIAN_POINT('Ctrl Pts',(-6.6501251838944,-1.55798279177326,-0.0257450798766383));
#51865=CARTESIAN_POINT('Ctrl Pts',(-6.61125781176667,-1.54596760635299,
-0.565999964779691));
#51866=CARTESIAN_POINT('Ctrl Pts',(-6.53534165801313,-0.920205969547918,
-1.59171295387702));
#51867=CARTESIAN_POINT('Ctrl Pts',(-6.42419531313571,0.838343369925463,
-1.63630973474875));
#51868=CARTESIAN_POINT('Ctrl Pts',(-6.31304896825829,1.82944061423442,-0.182965004634956));
#51869=CARTESIAN_POINT('Ctrl Pts',(-6.20190262338086,1.14579683626047,1.43787299993672));
#51870=CARTESIAN_POINT('Ctrl Pts',(-6.09075627850344,-0.586753886249875,
1.74242619094817));
#51871=CARTESIAN_POINT('Ctrl Pts',(-6.00743666217526,-1.48288220531212,
0.774993702200644));
#51872=CARTESIAN_POINT('Ctrl Pts',(-5.96116582747288,-1.55641487634798,
0.130195352308992));
#51873=CARTESIAN_POINT('Ctrl Pts',(-5.95194377439632,-1.5552490056676,0.0014214557352331));
#51874=CARTESIAN_POINT('Origin',(-30.9400562256037,0.,0.));
#51875=CARTESIAN_POINT('',(-7.49005622560373,-1.55396602392417,0.00116714021534956));
#51876=CARTESIAN_POINT('',(-7.35194377439631,-1.5538855757594,-0.00113247137955699));
#51877=CARTESIAN_POINT('',(-30.9400562256037,-1.5555,7.38654183493349E-13));
#51878=CARTESIAN_POINT('Ctrl Pts',(-7.49005622560373,-1.55396602392417,
0.00116714021534962));
#51879=CARTESIAN_POINT('Ctrl Pts',(-7.46561449190759,-1.5515811557621,-0.34084388051028));
#51880=CARTESIAN_POINT('Ctrl Pts',(-7.40412397658564,-1.271828585896,-1.20482146261895));
#51881=CARTESIAN_POINT('Ctrl Pts',(-7.30558467963788,0.156120132828023,
-1.83192679435794));
#51882=CARTESIAN_POINT('Ctrl Pts',(-7.19443833476045,1.62384116454318,-0.862246570359003));
#51883=CARTESIAN_POINT('Ctrl Pts',(-7.08329198988304,1.60503489891277,0.896767667254413));
#51884=CARTESIAN_POINT('Ctrl Pts',(-6.97214564500561,0.116917322223582,
1.83484593781736));
#51885=CARTESIAN_POINT('Ctrl Pts',(-6.87440039024584,-1.28590137517143,
1.1826521502983));
#51886=CARTESIAN_POINT('Ctrl Pts',(-6.81370391711189,-1.55166392198648,
0.329978981439988));
#51887=CARTESIAN_POINT('Ctrl Pts',(-6.79005622560374,-1.55372215258713,
-0.00105166811141207));
#51888=CARTESIAN_POINT('Ctrl Pts',(-7.35194377439631,-1.5538855757594,-0.00113247137955713));
#51889=CARTESIAN_POINT('Ctrl Pts',(-7.3390845403159,-1.55509892412473,-0.181094025918854));
#51890=CARTESIAN_POINT('Ctrl Pts',(-7.28917652460969,-1.44305374746564,
-0.878079590738082));
#51891=CARTESIAN_POINT('Ctrl Pts',(-7.20221972727767,-0.413558273857659,
-1.79145156452956));
#51892=CARTESIAN_POINT('Ctrl Pts',(-7.09107338240025,1.28090844667878,-1.31893999300895));
#51893=CARTESIAN_POINT('Ctrl Pts',(-6.97992703752282,1.80278180465922,0.360980496316825));
#51894=CARTESIAN_POINT('Ctrl Pts',(-6.8687806926454,0.674318650485929,1.71044541320042));
#51895=CARTESIAN_POINT('Ctrl Pts',(-6.7594529382699,-1.04287764167063,1.49764197438319));
#51896=CARTESIAN_POINT('Ctrl Pts',(-6.68717396552021,-1.5559639863464,0.489323158169705));
#51897=CARTESIAN_POINT('Ctrl Pts',(-6.65194377439632,-1.55788369592683,
-0.000462245611997049));
#51898=CARTESIAN_POINT('Origin',(-30.9400562256037,0.,0.));
#51899=CARTESIAN_POINT('',(-8.19005622560374,-1.5579254046757,0.000400362302149405));
#51900=CARTESIAN_POINT('',(-8.05194377439631,-1.55379656827821,0.0010903190078327));
#51901=CARTESIAN_POINT('',(-30.9400562256037,-1.5555,7.38654183493349E-13));
#51902=CARTESIAN_POINT('Ctrl Pts',(-8.19005622560374,-1.5579254046757,0.000400362302149489));
#51903=CARTESIAN_POINT('Ctrl Pts',(-8.15457384832911,-1.55622582261712,
-0.492855805043272));
#51904=CARTESIAN_POINT('Ctrl Pts',(-8.08204268942866,-1.03664772187573,
-1.50422548004318));
#51905=CARTESIAN_POINT('Ctrl Pts',(-7.97246274890243,0.685918408299438,
-1.70582684142229));
#51906=CARTESIAN_POINT('Ctrl Pts',(-7.86131640402499,1.80519161566156,-0.348729847455048));
#51907=CARTESIAN_POINT('Ctrl Pts',(-7.75017005914758,1.27192227624375,1.32760799898003));
#51908=CARTESIAN_POINT('Ctrl Pts',(-7.63902371427015,-0.425714136150784,
1.7886018981434));
#51909=CARTESIAN_POINT('Ctrl Pts',(-7.55231910308887,-1.44601574804416,
0.870928982546018));
#51910=CARTESIAN_POINT('Ctrl Pts',(-7.5026632735334,-1.55519613908698,0.17757644834238));
#51911=CARTESIAN_POINT('Ctrl Pts',(-7.49005622560373,-1.55396602392417,
0.00116714021534962));
#51912=CARTESIAN_POINT('Ctrl Pts',(-8.05194377439631,-1.55379656827821,
0.00109031900783265));
#51913=CARTESIAN_POINT('Ctrl Pts',(-8.02804389673742,-1.55163338209354,
-0.333430270496251));
#51914=CARTESIAN_POINT('Ctrl Pts',(-7.96709523745272,-1.28147121141093,
-1.18969909365111));
#51915=CARTESIAN_POINT('Ctrl Pts',(-7.86909779654222,0.12937469692319,-1.83400963512396));
#51916=CARTESIAN_POINT('Ctrl Pts',(-7.75795145166479,1.61108763178959,-0.885847501902045));
#51917=CARTESIAN_POINT('Ctrl Pts',(-7.64680510678736,1.61794834873923,0.873253854697203));
#51918=CARTESIAN_POINT('Ctrl Pts',(-7.53565876190995,0.143676280899092,
1.83294470190416));
#51919=CARTESIAN_POINT('Ctrl Pts',(-7.43737165111292,-1.27633745275613,
1.19778662186747));
#51920=CARTESIAN_POINT('Ctrl Pts',(-7.37613332194171,-1.55160314215653,
0.33739380107606));
#51921=CARTESIAN_POINT('Ctrl Pts',(-7.35194377439631,-1.5538855757594,-0.00113247137955713));
#51922=CARTESIAN_POINT('Origin',(-30.9400562256037,0.,0.));
#51923=CARTESIAN_POINT('',(-8.89005622560373,-1.55514414867911,-0.00141730865890474));
#51924=CARTESIAN_POINT('',(-8.75194377439631,-1.557829309021,0.000531961773406163));
#51925=CARTESIAN_POINT('',(-30.9400562256037,-1.5555,7.38654183493349E-13));
#51926=CARTESIAN_POINT('Ctrl Pts',(-8.89005622560373,-1.55514414867911,
-0.00141730865890458));
#51927=CARTESIAN_POINT('Ctrl Pts',(-8.88058198637642,-1.55633155915456,
-0.133735397335899));
#51928=CARTESIAN_POINT('Ctrl Pts',(-8.83405896552331,-1.48031737464662,
-0.782136131627296));
#51929=CARTESIAN_POINT('Ctrl Pts',(-8.75048716304438,-0.574907898574367,
-1.74637057462545));
#51930=CARTESIAN_POINT('Ctrl Pts',(-8.63934081816696,1.15553474640397,-1.43005899375302));
#51931=CARTESIAN_POINT('Ctrl Pts',(-8.52819447328953,1.82815598552823,0.195384155801151));
#51932=CARTESIAN_POINT('Ctrl Pts',(-8.41704812841212,0.827212201402232,
1.64196505736636));
#51933=CARTESIAN_POINT('Ctrl Pts',(-8.30590178353469,-0.930993773713778,
1.58542734588091));
#51934=CARTESIAN_POINT('Ctrl Pts',(-8.2302378159319,-1.54772004707537,0.558909923790492));
#51935=CARTESIAN_POINT('Ctrl Pts',(-8.19162262995491,-1.55800043439288,
0.022175639668584));
#51936=CARTESIAN_POINT('Ctrl Pts',(-8.19005622560374,-1.5579254046757,0.000400362302149489));
#51937=CARTESIAN_POINT('Ctrl Pts',(-8.75194377439631,-1.557829309021,0.000531961773406219));
#51938=CARTESIAN_POINT('Ctrl Pts',(-8.71700325315893,-1.55567394565809,
-0.485271528700681));
#51939=CARTESIAN_POINT('Ctrl Pts',(-8.64501395029575,-1.04998245345796,
-1.49006113550599));
#51940=CARTESIAN_POINT('Ctrl Pts',(-8.53597586580675,0.660956434360724,
-1.71565315428517));
#51941=CARTESIAN_POINT('Ctrl Pts',(-8.42482952092933,1.79991126531332,-0.375031453253858));
#51942=CARTESIAN_POINT('Ctrl Pts',(-8.31368317605192,1.29115738736595,1.30890861215818));
#51943=CARTESIAN_POINT('Ctrl Pts',(-8.20253683117448,-0.399572131671196,
1.79462287557114));
#51944=CARTESIAN_POINT('Ctrl Pts',(-8.11529036395596,-1.43961378644524,
0.886293114185729));
#51945=CARTESIAN_POINT('Ctrl Pts',(-8.06509267836323,-1.5549866801194,0.185132227888066));
#51946=CARTESIAN_POINT('Ctrl Pts',(-8.05194377439631,-1.55379656827821,
0.00109031900783265));
#51947=CARTESIAN_POINT('Origin',(-30.9400562256037,0.,0.));
#51948=CARTESIAN_POINT('',(-9.59005622560373,-1.55306820950157,0.00045046149979706));
#51949=CARTESIAN_POINT('',(-9.45194377439631,-1.55537042358935,-0.00142308536877606));
#51950=CARTESIAN_POINT('',(-30.9400562256037,-1.5555,7.38654183493349E-13));
#51951=CARTESIAN_POINT('Ctrl Pts',(-9.59005622560373,-1.55306820950157,
0.000450461499797109));
#51952=CARTESIAN_POINT('Ctrl Pts',(-9.56954134279794,-1.55232237073773,
-0.287028638890437));
#51953=CARTESIAN_POINT('Ctrl Pts',(-9.51197767836633,-1.33793859553732,
-1.09471369792781));
#51954=CARTESIAN_POINT('Ctrl Pts',(-9.41736523230892,-0.0381026721077461,
-1.83817231568183));
#51955=CARTESIAN_POINT('Ctrl Pts',(-9.30621888743151,1.5237653819353,-1.02881890368343));
#51956=CARTESIAN_POINT('Ctrl Pts',(-9.19507254255407,1.6907193985366,0.722355308122558));
#51957=CARTESIAN_POINT('Ctrl Pts',(-9.08392619767666,0.309923183800838,
1.81225740332426));
#51958=CARTESIAN_POINT('Ctrl Pts',(-8.98225409202653,-1.21270388908303,
1.29166012383535));
#51959=CARTESIAN_POINT('Ctrl Pts',(-8.91763076800223,-1.55168821942565,
0.383691264048035));
#51960=CARTESIAN_POINT('Ctrl Pts',(-8.89005622560373,-1.55514414867911,
-0.00141730865890458));
#51961=CARTESIAN_POINT('Ctrl Pts',(-9.45194377439631,-1.55537042358935,
-0.00142308536877613));
#51962=CARTESIAN_POINT('Ctrl Pts',(-9.44301139120625,-1.55650874018037,
-0.126127277143475));
#51963=CARTESIAN_POINT('Ctrl Pts',(-9.39703022639039,-1.48579298819755,
-0.766791032011734));
#51964=CARTESIAN_POINT('Ctrl Pts',(-9.31400027994872,-0.600327192984703,
-1.73779642515878));
#51965=CARTESIAN_POINT('Ctrl Pts',(-9.20285393507129,1.13454637823559,-1.44676662581219));
#51966=CARTESIAN_POINT('Ctrl Pts',(-9.09170759019388,1.83081211133877,0.168689557788168));
#51967=CARTESIAN_POINT('Ctrl Pts',(-8.98056124531644,0.851081300419372,
1.62972076565527));
#51968=CARTESIAN_POINT('Ctrl Pts',(-8.86941490043904,-0.907762402178502,
1.59884226086334));
#51969=CARTESIAN_POINT('Ctrl Pts',(-8.79320907679898,-1.54392384656025,
0.574146475722241));
#51970=CARTESIAN_POINT('Ctrl Pts',(-8.75405203478474,-1.55795936052109,
0.0298446399836376));
#51971=CARTESIAN_POINT('Ctrl Pts',(-8.75194377439631,-1.557829309021,0.000531961773406219));
#51972=CARTESIAN_POINT('Origin',(-30.9400562256037,0.,0.));
#51973=CARTESIAN_POINT('',(-10.2900562256037,-1.55679549104668,0.001183809171597));
#51974=CARTESIAN_POINT('',(-10.1519437743963,-1.55301127595102,0.000330442370898021));
#51975=CARTESIAN_POINT('',(-30.9400562256037,-1.5555,7.38654183493349E-13));
#51976=CARTESIAN_POINT('Ctrl Pts',(-10.2900562256037,-1.55679549104668,
0.00118380917159693));
#51977=CARTESIAN_POINT('Ctrl Pts',(-10.2585006992194,-1.5530840694091,-0.438321856345931));
#51978=CARTESIAN_POINT('Ctrl Pts',(-10.1898963912094,-1.12899939113678,
-1.40010995221672));
#51979=CARTESIAN_POINT('Ctrl Pts',(-10.0842433015735,0.502045652602867,
-1.76869427501289));
#51980=CARTESIAN_POINT('Ctrl Pts',(-9.97309695669603,1.75830205085506,-0.537311058624067));
#51981=CARTESIAN_POINT('Ctrl Pts',(-9.86195061181863,1.40494043187336,1.1859475783728));
#51982=CARTESIAN_POINT('Ctrl Pts',(-9.75080426694118,-0.234558248248651,
1.82354372142247));
#51983=CARTESIAN_POINT('Ctrl Pts',(-9.66017280486957,-1.39635476617201,
0.982232150910424));
#51984=CARTESIAN_POINT('Ctrl Pts',(-9.60659012442374,-1.55366931567284,
0.232143247840176));
#51985=CARTESIAN_POINT('Ctrl Pts',(-9.59005622560373,-1.55306820950157,
0.000450461499797109));
#51986=CARTESIAN_POINT('Ctrl Pts',(-10.1519437743963,-1.55301127595102,
0.000330442370898004));
#51987=CARTESIAN_POINT('Ctrl Pts',(-10.1319707476278,-1.55247970594514,
-0.279581117167299));
#51988=CARTESIAN_POINT('Ctrl Pts',(-10.0749489392334,-1.34638723470874,
-1.07944192578539));
#51989=CARTESIAN_POINT('Ctrl Pts',(-9.98087834921326,-0.0649185555153559,
-1.83742067450035));
#51990=CARTESIAN_POINT('Ctrl Pts',(-9.86973200433583,1.50859212232134,-1.05094194054737));
#51991=CARTESIAN_POINT('Ctrl Pts',(-9.75858565945843,1.70107895413302,0.697609880762318));
#51992=CARTESIAN_POINT('Ctrl Pts',(-9.64743931458098,0.33633201488792,1.80754251117172));
#51993=CARTESIAN_POINT('Ctrl Pts',(-9.54522535289363,-1.20188312644262,
1.30656081858063));
#51994=CARTESIAN_POINT('Ctrl Pts',(-9.48006017283206,-1.55178735262855,
0.391107403745289));
#51995=CARTESIAN_POINT('Ctrl Pts',(-9.45194377439631,-1.55537042358935,
-0.00142308536877613));
#51996=CARTESIAN_POINT('Origin',(-30.9400562256037,0.,0.));
#51997=CARTESIAN_POINT('',(-10.9900562256037,-1.55677461884647,-0.00119118501635344));
#51998=CARTESIAN_POINT('',(-10.8519437743963,-1.55658271042523,0.00125264783408005));
#51999=CARTESIAN_POINT('',(-30.9400562256037,-1.5555,7.38654183493349E-13));
#52000=CARTESIAN_POINT('Ctrl Pts',(-10.9900562256037,-1.55677461884647,
-0.00119118501635364));
#52001=CARTESIAN_POINT('Ctrl Pts',(-10.9845088372668,-1.55742983376792,
-0.0784579566522596));
#52002=CARTESIAN_POINT('Ctrl Pts',(-10.941912667304,-1.51707611203411,-0.671071724150687));
#52003=CARTESIAN_POINT('Ctrl Pts',(-10.8622677157155,-0.756017527849028,
-1.67593758038474));
#52004=CARTESIAN_POINT('Ctrl Pts',(-10.751121370838,0.998144889762121,-1.54403240082667));
#52005=CARTESIAN_POINT('Ctrl Pts',(-10.6399750259606,1.83856669176645,0.00134003275348477));
#52006=CARTESIAN_POINT('Ctrl Pts',(-10.5288286810832,0.99589310551582,1.54548574828332));
#52007=CARTESIAN_POINT('Ctrl Pts',(-10.4176823362057,-0.758459725548137,
1.67483375905857));
#52008=CARTESIAN_POINT('Ctrl Pts',(-10.3380915177126,-1.51753643586647,
0.669543322081447));
#52009=CARTESIAN_POINT('Ctrl Pts',(-10.2955494808453,-1.55744158346535,
0.0776939193622526));
#52010=CARTESIAN_POINT('Ctrl Pts',(-10.2900562256037,-1.55679549104668,
0.00118380917159693));
#52011=CARTESIAN_POINT('Ctrl Pts',(-10.8519437743963,-1.55658271042523,
0.00125264783408));
#52012=CARTESIAN_POINT('Ctrl Pts',(-10.8209301040493,-1.55279711529182,
-0.430859426859307));
#52013=CARTESIAN_POINT('Ctrl Pts',(-10.7528676520765,-1.14097100020651,
-1.38550035281079));
#52014=CARTESIAN_POINT('Ctrl Pts',(-10.6477564184778,0.476185984549256,
-1.77583109051801));
#52015=CARTESIAN_POINT('Ctrl Pts',(-10.5366100736004,1.7502751895651,-0.562908442576898));
#52016=CARTESIAN_POINT('Ctrl Pts',(-10.4254637287229,1.4220944780604,1.16532246584438));
#52017=CARTESIAN_POINT('Ctrl Pts',(-10.3143173838456,-0.207926774994991,
1.82677190972811));
#52018=CARTESIAN_POINT('Ctrl Pts',(-10.2231440657366,-1.38889345108409,
0.99757311028931));
#52019=CARTESIAN_POINT('Ctrl Pts',(-10.1690195292536,-1.55346573682043,
0.239638246229552));
#52020=CARTESIAN_POINT('Ctrl Pts',(-10.1519437743963,-1.55301127595102,
0.000330442370898004));
#52021=CARTESIAN_POINT('Origin',(-30.9400562256037,0.,0.));
#52022=CARTESIAN_POINT('',(-11.6900562256037,-1.5530617356523,-0.000438607636642084));
#52023=CARTESIAN_POINT('',(-11.5519437743963,-1.55697909484695,-0.00111249417114406));
#52024=CARTESIAN_POINT('',(-30.9400562256037,-1.5555,7.38654183493349E-13));
#52025=CARTESIAN_POINT('Ctrl Pts',(-11.6900562256037,-1.5530617356523,-0.000438607636642063));
#52026=CARTESIAN_POINT('Ctrl Pts',(-11.6734681936883,-1.55364880148782,
-0.232892390880623));
#52027=CARTESIAN_POINT('Ctrl Pts',(-11.619831380147,-1.39561614963909,-0.983765069282232));
#52028=CARTESIAN_POINT('Ctrl Pts',(-11.52914578498,-0.231899833827511,-1.82388369772625));
#52029=CARTESIAN_POINT('Ctrl Pts',(-11.4179994401025,1.40666768559556,-1.18389834785848));
#52030=CARTESIAN_POINT('Ctrl Pts',(-11.3068530952251,1.75751694870754,0.539873550719585));
#52031=CARTESIAN_POINT('Ctrl Pts',(-11.1957067503477,0.499466907597081,
1.7694242238582));
#52032=CARTESIAN_POINT('Ctrl Pts',(-11.0901077938073,-1.13020370428311,
1.39865279944782));
#52033=CARTESIAN_POINT('Ctrl Pts',(-11.0215576188926,-1.55305391611653,
0.437575819133659));
#52034=CARTESIAN_POINT('Ctrl Pts',(-10.9900562256037,-1.55677461884647,
-0.00119118501635364));
#52035=CARTESIAN_POINT('Ctrl Pts',(-11.5519437743963,-1.55697909484695,
-0.00111249417114408));
#52036=CARTESIAN_POINT('Ctrl Pts',(-11.5469382420966,-1.55754273633745,
-0.0708081666518759));
#52037=CARTESIAN_POINT('Ctrl Pts',(-11.5048839281711,-1.52162841675364,
-0.655776625116939));
#52038=CARTESIAN_POINT('Ctrl Pts',(-11.4257808326198,-0.780389884361033,
-1.66472844101327));
#52039=CARTESIAN_POINT('Ctrl Pts',(-11.3146344877423,0.975510343836714,
-1.55843149448383));
#52040=CARTESIAN_POINT('Ctrl Pts',(-11.2034881428649,1.83839049924661,-0.0254858041131052));
#52041=CARTESIAN_POINT('Ctrl Pts',(-11.0923417979875,1.01833655988029,1.53079058160895));
#52042=CARTESIAN_POINT('Ctrl Pts',(-10.9811954531101,-0.733942234478493,
1.68572178913967));
#52043=CARTESIAN_POINT('Ctrl Pts',(-10.9010627785797,-1.51287298574345,
0.684845816257308));
#52044=CARTESIAN_POINT('Ctrl Pts',(-10.8579788856751,-1.5573193690545,0.0853395819666858));
#52045=CARTESIAN_POINT('Ctrl Pts',(-10.8519437743963,-1.55658271042523,
0.00125264783408));
#52046=CARTESIAN_POINT('Origin',(-30.9400562256037,0.,0.));
#52047=CARTESIAN_POINT('',(-12.3900562256037,-1.55516658951858,0.00141841178062525));
#52048=CARTESIAN_POINT('',(-12.2519437743963,-1.55313429879201,-0.000555641002405599));
#52049=CARTESIAN_POINT('',(-30.9400562256037,-1.5555,7.38654183493349E-13));
#52050=CARTESIAN_POINT('Ctrl Pts',(-12.3900562256037,-1.55516658951858,
0.00141841178062522));
#52051=CARTESIAN_POINT('Ctrl Pts',(-12.3624275501098,-1.55169695808864,
-0.3844320052266));
#52052=CARTESIAN_POINT('Ctrl Pts',(-12.29775009299,-1.21163085071126,-1.29315050173403));
#52053=CARTESIAN_POINT('Ctrl Pts',(-12.1960238542445,0.312564567770197,
-1.81180370535426));
#52054=CARTESIAN_POINT('Ctrl Pts',(-12.0848775093671,1.69177057386242,-0.719889992411354));
#52055=CARTESIAN_POINT('Ctrl Pts',(-11.9737311644897,1.52226406188029,1.0310389913425));
#52056=CARTESIAN_POINT('Ctrl Pts',(-11.8625848196122,-0.0407821208305537,
1.83811482078279));
#52057=CARTESIAN_POINT('Ctrl Pts',(-11.7680265066503,-1.33878984124311,
1.09318869047629));
#52058=CARTESIAN_POINT('Ctrl Pts',(-11.7105169753141,-1.55233761074191,
0.286284898950973));
#52059=CARTESIAN_POINT('Ctrl Pts',(-11.6900562256037,-1.5530617356523,-0.000438607636642063));
#52060=CARTESIAN_POINT('Ctrl Pts',(-12.2519437743963,-1.553134298792,-0.000555641002405547));
#52061=CARTESIAN_POINT('Ctrl Pts',(-12.2358975985181,-1.55385563286349,
-0.225389960215645));
#52062=CARTESIAN_POINT('Ctrl Pts',(-12.1828026410141,-1.40294188872054,
-0.968418244866292));
#52063=CARTESIAN_POINT('Ctrl Pts',(-12.0926589018843,-0.258486605724834,
-1.82030597114671));
#52064=CARTESIAN_POINT('Ctrl Pts',(-11.9815125570069,1.38924419891378,-1.20429635460542));
#52065=CARTESIAN_POINT('Ctrl Pts',(-11.8703662121295,1.76520688394983,0.514172938599101));
#52066=CARTESIAN_POINT('Ctrl Pts',(-11.759219867252,0.525230599245605,1.76194834531198));
#52067=CARTESIAN_POINT('Ctrl Pts',(-11.6530790546743,-1.11806540396333,
1.41321386829771));
#52068=CARTESIAN_POINT('Ctrl Pts',(-11.5839870237224,-1.55337090620096,
0.445049008049826));
#52069=CARTESIAN_POINT('Ctrl Pts',(-11.5519437743963,-1.55697909484695,
-0.00111249417114408));
#52070=CARTESIAN_POINT('Origin',(-30.9400562256037,0.,0.));
#52071=CARTESIAN_POINT('',(-13.0900562256037,-1.55791691533987,-0.000413732030063911));
#52072=CARTESIAN_POINT('',(-12.9519437743963,-1.55494406527359,0.00140217176205479));
#52073=CARTESIAN_POINT('',(-30.9400562256037,-1.5555,7.38654183493349E-13));
#52074=CARTESIAN_POINT('Ctrl Pts',(-13.0900562256037,-1.55791691533987,
-0.000413732030063846));
#52075=CARTESIAN_POINT('Ctrl Pts',(-13.0884356881571,-1.55799687247773,
-0.0229418655251971));
#52076=CARTESIAN_POINT('Ctrl Pts',(-13.0497663690847,-1.54734598542797,
-0.560431660655591));
#52077=CARTESIAN_POINT('Ctrl Pts',(-12.9740482683865,-0.928681719728038,
-1.58678276370895));
#52078=CARTESIAN_POINT('Ctrl Pts',(-12.8629019235091,0.829604801984373,
-1.64075749222281));
#52079=CARTESIAN_POINT('Ctrl Pts',(-12.7517555786316,1.82843885316793,-0.192719059739105));
#52080=CARTESIAN_POINT('Ctrl Pts',(-12.6406092337542,1.15344893307288,1.43174188824448));
#52081=CARTESIAN_POINT('Ctrl Pts',(-12.5294628888768,-0.577452958307463,
1.74553068053895));
#52082=CARTESIAN_POINT('Ctrl Pts',(-12.4459452194933,-1.48087035346453,
0.780602884632271));
#52083=CARTESIAN_POINT('Ctrl Pts',(-12.3994763317356,-1.55634957407083,
0.132975636810733));
#52084=CARTESIAN_POINT('Ctrl Pts',(-12.3900562256037,-1.55516658951858,
0.00141841178062522));
#52085=CARTESIAN_POINT('Ctrl Pts',(-12.9519437743963,-1.55494406527359,
0.001402171762055));
#52086=CARTESIAN_POINT('Ctrl Pts',(-12.9248569549396,-1.55162083135455,
-0.377018655819353));
#52087=CARTESIAN_POINT('Ctrl Pts',(-12.8607213538571,-1.22229200510013,
-1.27821529541056));
#52088=CARTESIAN_POINT('Ctrl Pts',(-12.7595369711488,0.286096082776584,
-1.81617129846043));
#52089=CARTESIAN_POINT('Ctrl Pts',(-12.6483906262714,1.6810868693329,-0.74449720730706));
#52090=CARTESIAN_POINT('Ctrl Pts',(-12.537244281394,1.53714541606292,1.00871855530086));
#52091=CARTESIAN_POINT('Ctrl Pts',(-12.4260979365166,-0.0139586777784811,
1.83851415802169));
#52092=CARTESIAN_POINT('Ctrl Pts',(-12.3309977675173,-1.33019666661088,
1.10844624262991));
#52093=CARTESIAN_POINT('Ctrl Pts',(-12.2729463801439,-1.55219015513867,
0.293726722647215));
#52094=CARTESIAN_POINT('Ctrl Pts',(-12.2519437743963,-1.553134298792,-0.000555641002405547));
#52095=CARTESIAN_POINT('Origin',(-30.9400562256037,0.,0.));
#52096=CARTESIAN_POINT('',(-13.7900562256037,-1.55394853714682,-0.00115986111943391));
#52097=CARTESIAN_POINT('',(-13.6519437743963,-1.55799009741835,-0.000278060196764462));
#52098=CARTESIAN_POINT('',(-30.9400562256037,-1.5555,7.38654183493349E-13));
#52099=CARTESIAN_POINT('Ctrl Pts',(-13.7900562256037,-1.55394853714682,
-0.00115986111943394));
#52100=CARTESIAN_POINT('Ctrl Pts',(-13.7773950445786,-1.55517532350031,
-0.178331666446028));
#52101=CARTESIAN_POINT('Ctrl Pts',(-13.7276850819277,-1.44538251435531,
-0.872463892850537));
#52102=CARTESIAN_POINT('Ctrl Pts',(-13.640926337651,-0.423106453057855,
-1.78922055799212));
#52103=CARTESIAN_POINT('Ctrl Pts',(-13.5297799927736,1.27385616856038,-1.32575251747129));
#52104=CARTESIAN_POINT('Ctrl Pts',(-13.4186336478962,1.8046813570327,0.351360890452264));
#52105=CARTESIAN_POINT('Ctrl Pts',(-13.3074873030187,0.683431109300355,
1.70682488691761));
#52106=CARTESIAN_POINT('Ctrl Pts',(-13.1979614955879,-1.03798850696033,
1.50281360125476));
#52107=CARTESIAN_POINT('Ctrl Pts',(-13.1254844697829,-1.55616888970194,
0.492097080379339));
#52108=CARTESIAN_POINT('Ctrl Pts',(-13.0900562256037,-1.55791691533987,
-0.000413732030063846));
#52109=CARTESIAN_POINT('Ctrl Pts',(-13.6519437743963,-1.55799009741835,
-0.000278060196764374));
#52110=CARTESIAN_POINT('Ctrl Pts',(-13.6508650929869,-1.55802707523786,
-0.0152716175721371));
#52111=CARTESIAN_POINT('Ctrl Pts',(-13.6127376299518,-1.55103858389315,
-0.545203987085675));
#52112=CARTESIAN_POINT('Ctrl Pts',(-13.5375613852908,-0.951734875856344,
-1.57306385121844));
#52113=CARTESIAN_POINT('Ctrl Pts',(-13.4264150404134,0.805576927784317,
-1.65268719585804));
#52114=CARTESIAN_POINT('Ctrl Pts',(-13.315268695536,1.82543231055633,-0.219376465256566));
#52115=CARTESIAN_POINT('Ctrl Pts',(-13.2041223506585,1.1742160279774,1.41476000564494));
#52116=CARTESIAN_POINT('Ctrl Pts',(-13.0929760057811,-0.55192323148034,
1.75377019603021));
#52117=CARTESIAN_POINT('Ctrl Pts',(-13.0089164803604,-1.47527528717852,
0.795952296887006));
#52118=CARTESIAN_POINT('Ctrl Pts',(-12.9619057365654,-1.55616628077341,
0.140577388490967));
#52119=CARTESIAN_POINT('Ctrl Pts',(-12.9519437743963,-1.55494406527359,
0.001402171762055));
#52120=CARTESIAN_POINT('Origin',(-30.9400562256037,0.,0.));
#52121=CARTESIAN_POINT('',(-14.4900562256037,-1.55373788793014,0.00106011422664349));
#52122=CARTESIAN_POINT('',(-14.3519437743963,-1.55412884799482,-0.00122858297720713));
#52123=CARTESIAN_POINT('',(-30.9400562256037,-1.5555,7.38654183493349E-13));
#52124=CARTESIAN_POINT('Ctrl Pts',(-14.4900562256037,-1.55373788793014,
0.00106011422664335));
#52125=CARTESIAN_POINT('Ctrl Pts',(-14.4663544010001,-1.55165705021594,
-0.330719875177941));
#52126=CARTESIAN_POINT('Ctrl Pts',(-14.4056037947708,-1.28495349846119,
-1.18416527816597));
#52127=CARTESIAN_POINT('Ctrl Pts',(-14.3078044069155,0.119591838376424,
-1.83467355896208));
#52128=CARTESIAN_POINT('Ctrl Pts',(-14.1966580620381,1.60634040478516,-0.894427067857099));
#52129=CARTESIAN_POINT('Ctrl Pts',(-14.0855117171607,1.62258254933333,0.864612714664634));
#52130=CARTESIAN_POINT('Ctrl Pts',(-13.9743653722833,0.153449581803269,
1.83215242313658));
#52131=CARTESIAN_POINT('Ctrl Pts',(-13.875880208431,-1.27279954501849,1.2033118949607));
#52132=CARTESIAN_POINT('Ctrl Pts',(-13.8144438262044,-1.55158553676384,
0.340103344694499));
#52133=CARTESIAN_POINT('Ctrl Pts',(-13.7900562256037,-1.55394853714682,
-0.00115986111943394));
#52134=CARTESIAN_POINT('Ctrl Pts',(-14.3519437743963,-1.55412884799482,
-0.00122858297720718));
#52135=CARTESIAN_POINT('Ctrl Pts',(-14.3398244494084,-1.55538235764995,
-0.170768466806927));
#52136=CARTESIAN_POINT('Ctrl Pts',(-14.2906563427948,-1.45165790061733,
-0.857100278990044));
#52137=CARTESIAN_POINT('Ctrl Pts',(-14.2044394545554,-0.449167113826005,
-1.78285671263529));
#52138=CARTESIAN_POINT('Ctrl Pts',(-14.0932931096779,1.25437709178756,-1.34419762889618));
#52139=CARTESIAN_POINT('Ctrl Pts',(-13.9821467648005,1.80961576800425,0.324992193939892));
#52140=CARTESIAN_POINT('Ctrl Pts',(-13.8710004199231,0.708261856483432,
1.69667153467668));
#52141=CARTESIAN_POINT('Ctrl Pts',(-13.760932756455,-1.02448130719353,1.51691348615434));
#52142=CARTESIAN_POINT('Ctrl Pts',(-13.6879138746128,-1.5567570216814,0.499702524170623));
#52143=CARTESIAN_POINT('Ctrl Pts',(-13.6519437743963,-1.55799009741835,
-0.000278060196764374));
#52144=CARTESIAN_POINT('Origin',(-30.9400562256037,0.,0.));
#52145=CARTESIAN_POINT('',(-15.1900562256037,-1.5577883204632,0.000578693956271592));
#52146=CARTESIAN_POINT('',(-15.0519437743963,-1.55358657070994,0.000972031055979372));
#52147=CARTESIAN_POINT('',(-30.9400562256037,-1.5555,7.38654183493349E-13));
#52148=CARTESIAN_POINT('Ctrl Pts',(-15.1900562256037,-1.5577883204632,0.00057869395627152));
#52149=CARTESIAN_POINT('Ctrl Pts',(-15.1553137574216,-1.55548217457295,
-0.482504970374552));
#52150=CARTESIAN_POINT('Ctrl Pts',(-15.0835225076138,-1.05480877594759,
-1.48486659917243));
#52151=CARTESIAN_POINT('Ctrl Pts',(-14.9746824761801,0.651797236720689,
-1.71915375634761));
#52152=CARTESIAN_POINT('Ctrl Pts',(-14.8635361313027,1.79788560735673,-0.384625296386388));
#52153=CARTESIAN_POINT('Ctrl Pts',(-14.7523897864252,1.29811963509442,1.30200410473359));
#52154=CARTESIAN_POINT('Ctrl Pts',(-14.6412434415478,-0.389995490350614,
1.79672835822976));
#52155=CARTESIAN_POINT('Ctrl Pts',(-14.553798921274,-1.43723851868735,0.891908855350462));
#52156=CARTESIAN_POINT('Ctrl Pts',(-14.5034031826259,-1.55490964799528,
0.187891859608462));
#52157=CARTESIAN_POINT('Ctrl Pts',(-14.4900562256037,-1.55373788793014,
0.00106011422664335));
#52158=CARTESIAN_POINT('Ctrl Pts',(-15.0519437743963,-1.55358657070994,
0.000972031055979285));
#52159=CARTESIAN_POINT('Ctrl Pts',(-15.02878380583,-1.55173352040061,-0.323302252679583));
#52160=CARTESIAN_POINT('Ctrl Pts',(-14.9685750556378,-1.29436586684795,
-1.16900831967119));
#52161=CARTESIAN_POINT('Ctrl Pts',(-14.8713175238199,0.0928102146840508,
-1.83622313948545));
#52162=CARTESIAN_POINT('Ctrl Pts',(-14.7601711789425,1.59311920419314,-0.917769227618005));
#52163=CARTESIAN_POINT('Ctrl Pts',(-14.649024834065,1.63502497258126,0.840846295684967));
#52164=CARTESIAN_POINT('Ctrl Pts',(-14.5378784891876,0.180165351192192,
1.82971844833059));
#52165=CARTESIAN_POINT('Ctrl Pts',(-14.438851469298,-1.2630037891826,1.21840966606724));
#52166=CARTESIAN_POINT('Ctrl Pts',(-14.3768732310343,-1.5515503781028,0.347515029937033));
#52167=CARTESIAN_POINT('Ctrl Pts',(-14.3519437743963,-1.55412884799482,
-0.00122858297720718));
#52168=CARTESIAN_POINT('Origin',(-30.9400562256037,0.,0.));
#52169=CARTESIAN_POINT('',(-15.8900562256037,-1.55545392515721,-0.00142225739221978));
#52170=CARTESIAN_POINT('',(-15.7519437743963,-1.55766118063764,0.0007021623802533));
#52171=CARTESIAN_POINT('',(-30.9400562256037,-1.5555,7.38654183493349E-13));
#52172=CARTESIAN_POINT('Ctrl Pts',(-15.8900562256037,-1.55545392515721,
-0.00142225739221964));
#52173=CARTESIAN_POINT('Ctrl Pts',(-15.881321895469,-1.55657175029418,-0.123344733807148));
#52174=CARTESIAN_POINT('Ctrl Pts',(-15.8355387837084,-1.48776154766086,
-0.761183597128199));
#52175=CARTESIAN_POINT('Ctrl Pts',(-15.7527068903221,-0.609586569357517,
-1.73457011683579));
#52176=CARTESIAN_POINT('Ctrl Pts',(-15.6415605454446,1.12681446224207,-1.45279676604917));
#52177=CARTESIAN_POINT('Ctrl Pts',(-15.5304142005672,1.83168575205326,0.158923193668888));
#52178=CARTESIAN_POINT('Ctrl Pts',(-15.4192678556898,0.859760733185979,
1.6251586868464));
#52179=CARTESIAN_POINT('Ctrl Pts',(-15.3081215108124,-0.899222667358879,
1.60366077156884));
#52180=CARTESIAN_POINT('Ctrl Pts',(-15.231717634117,-1.54250743087965,0.579718025313162));
#52181=CARTESIAN_POINT('Ctrl Pts',(-15.1923625390475,-1.55794140962319,
0.0326472949451707));
#52182=CARTESIAN_POINT('Ctrl Pts',(-15.1900562256037,-1.5577883204632,0.00057869395627152));
#52183=CARTESIAN_POINT('Ctrl Pts',(-15.7519437743963,-1.55766118063764,
0.000702162380253313));
#52184=CARTESIAN_POINT('Ctrl Pts',(-15.7177431622515,-1.55498402201236,
-0.474950124415379));
#52185=CARTESIAN_POINT('Ctrl Pts',(-15.6464937684809,-1.06788313969608,
-1.47060850547255));
#52186=CARTESIAN_POINT('Ctrl Pts',(-15.5381955930844,0.626644448535124,
-1.72848080378452));
#52187=CARTESIAN_POINT('Ctrl Pts',(-15.427049248207,1.79208230060405,-0.410816481890913));
#52188=CARTESIAN_POINT('Ctrl Pts',(-15.3159029033296,1.31697838226697,1.28292521004654));
#52189=CARTESIAN_POINT('Ctrl Pts',(-15.2047565584522,-0.363738719182501,
1.80222731587859));
#52190=CARTESIAN_POINT('Ctrl Pts',(-15.1167701821411,-1.43064249288966,
0.907272496897055));
#52191=CARTESIAN_POINT('Ctrl Pts',(-15.0658325874558,-1.55469782737086,
0.195436237425902));
#52192=CARTESIAN_POINT('Ctrl Pts',(-15.0519437743963,-1.55358657070994,
0.000972031055979285));
#52193=CARTESIAN_POINT('Origin',(-30.9400562256037,0.,0.));
#52194=CARTESIAN_POINT('',(-16.5900562256037,-1.55299491568328,0.00028591225007826));
#52195=CARTESIAN_POINT('',(-16.4519437743963,-1.55568344433103,-0.00141187396391018));
#52196=CARTESIAN_POINT('',(-30.9400562256037,-1.5555,7.38654183493349E-13));
#52197=CARTESIAN_POINT('Ctrl Pts',(-16.5900562256037,-1.55299491568328,
0.000285912250078488));
#52198=CARTESIAN_POINT('Ctrl Pts',(-16.5702812518905,-1.55253980973498,
-0.276857339627901));
#52199=CARTESIAN_POINT('Ctrl Pts',(-16.5134574965514,-1.34943550918954,
-1.07385631818032));
#52200=CARTESIAN_POINT('Ctrl Pts',(-16.4195849595866,-0.0747168460009575,
-1.83704835774251));
#52201=CARTESIAN_POINT('Ctrl Pts',(-16.3084386147092,1.50296588015394,-1.05897253923504));
#52202=CARTESIAN_POINT('Ctrl Pts',(-16.1972922698318,1.70477524097488,0.688527888701595));
#52203=CARTESIAN_POINT('Ctrl Pts',(-16.0861459249543,0.345967106142554,
1.80572313415655));
#52204=CARTESIAN_POINT('Ctrl Pts',(-15.9837339102117,-1.19788362025332,
1.31199725711552));
#52205=CARTESIAN_POINT('Ctrl Pts',(-15.9183706770948,-1.55183022361081,
0.393819047993088));
#52206=CARTESIAN_POINT('Ctrl Pts',(-15.8900562256037,-1.55545392515721,
-0.00142225739221964));
#52207=CARTESIAN_POINT('Ctrl Pts',(-16.4519437743963,-1.55568344433103,
-0.00141187396391032));
#52208=CARTESIAN_POINT('Ctrl Pts',(-16.4437513002988,-1.55673883175469,
-0.115727400980526));
#52209=CARTESIAN_POINT('Ctrl Pts',(-16.3985100445755,-1.4930580543659,-0.745845982010793));
#52210=CARTESIAN_POINT('Ctrl Pts',(-16.3162200072264,-0.634829996541143,
-1.72549124292854));
#52211=CARTESIAN_POINT('Ctrl Pts',(-16.205073662349,1.10549739525827,-1.46908293265175));
#52212=CARTESIAN_POINT('Ctrl Pts',(-16.0939273174715,1.83380951667369,0.132180976273241));
#52213=CARTESIAN_POINT('Ctrl Pts',(-15.9827809725941,0.883381152756941,
1.61244128354657));
#52214=CARTESIAN_POINT('Ctrl Pts',(-15.8716346277167,-0.875728642698206,
1.61661018748783));
#52215=CARTESIAN_POINT('Ctrl Pts',(-15.7946888949841,-1.53855244475298,
0.59496787199439));
#52216=CARTESIAN_POINT('Ctrl Pts',(-15.7547919438773,-1.55788412990709,
0.0403136851530925));
#52217=CARTESIAN_POINT('Ctrl Pts',(-15.7519437743963,-1.55766118063764,
0.000702162380253313));
#52218=CARTESIAN_POINT('Origin',(-30.9400562256037,0.,0.));
#52219=CARTESIAN_POINT('',(-17.2900562256037,-1.55650306831887,0.00127499959212149));
#52220=CARTESIAN_POINT('',(-17.1519437743963,-1.55296225729592,0.000162760582741173));
#52221=CARTESIAN_POINT('',(-30.9400562256037,-1.5555,7.38654183493349E-13));
#52222=CARTESIAN_POINT('Ctrl Pts',(-17.2900562256037,-1.55650306831887,
0.00127499959212141));
#52223=CARTESIAN_POINT('Ctrl Pts',(-17.259240608312,-1.55270042160587,-0.428134586038267));
#52224=CARTESIAN_POINT('Ctrl Pts',(-17.1913762093945,-1.14530073562805,
-1.38014743223044));
#52225=CARTESIAN_POINT('Ctrl Pts',(-17.0864630288511,0.466708474190256,
-1.7783454321025));
#52226=CARTESIAN_POINT('Ctrl Pts',(-16.9753166839737,1.74724826325126,-0.572234901352823));
#52227=CARTESIAN_POINT('Ctrl Pts',(-16.8641703390963,1.42828910175244,1.15772169262565));
#52228=CARTESIAN_POINT('Ctrl Pts',(-16.7530239942189,-0.19818140052057,
1.82785486520361));
#52229=CARTESIAN_POINT('Ctrl Pts',(-16.6616526230547,-1.38612848041481,
1.00317856130571));
#52230=CARTESIAN_POINT('Ctrl Pts',(-16.6073300335163,-1.55339245920696,
0.242375705472255));
#52231=CARTESIAN_POINT('Ctrl Pts',(-16.5900562256037,-1.55299491568328,
0.000285912250078488));
#52232=CARTESIAN_POINT('Ctrl Pts',(-17.1519437743963,-1.55296225729592,
0.000162760582741381));
#52233=CARTESIAN_POINT('Ctrl Pts',(-17.1327106567203,-1.5527105748812,-0.269400586387375));
#52234=CARTESIAN_POINT('Ctrl Pts',(-17.0764287574185,-1.35766705289621,
-1.05856521250988));
#52235=CARTESIAN_POINT('Ctrl Pts',(-16.9830980764909,-0.101512432092709,
-1.83576261538962));
#52236=CARTESIAN_POINT('Ctrl Pts',(-16.8719517316135,1.48735487692949,-1.08078888965679));
#52237=CARTESIAN_POINT('Ctrl Pts',(-16.7608053867361,1.71463973954429,0.663580980368641));
#52238=CARTESIAN_POINT('Ctrl Pts',(-16.6496590418587,0.372276761224383,
1.80048303712748));
#52239=CARTESIAN_POINT('Ctrl Pts',(-16.5467051710787,-1.18681899835157,
1.32684253683931));
#52240=CARTESIAN_POINT('Ctrl Pts',(-16.4808000819246,-1.55196605887505,
0.401241093088767));
#52241=CARTESIAN_POINT('Ctrl Pts',(-16.4519437743963,-1.55568344433103,
-0.00141187396391032));
#52242=CARTESIAN_POINT('Origin',(-30.9400562256037,0.,0.));
#52243=CARTESIAN_POINT('',(-17.9900562256037,-1.55705119782931,-0.00108109148358255));
#52244=CARTESIAN_POINT('',(-17.8519437743963,-1.5562809354664,0.00132828490436523));
#52245=CARTESIAN_POINT('',(-30.9400562256037,-1.5555,7.38654183493349E-13));
#52246=CARTESIAN_POINT('Ctrl Pts',(-17.9900562256037,-1.55705119782931,
-0.00108109148358261));
#52247=CARTESIAN_POINT('Ctrl Pts',(-17.9852487463593,-1.55758140962675,
-0.0680110357998723));
#52248=CARTESIAN_POINT('Ctrl Pts',(-17.9433924854891,-1.52326178500861,
-0.650188269130915));
#52249=CARTESIAN_POINT('Ctrl Pts',(-17.8644874429931,-0.789257021834459,
-1.66054287184818));
#52250=CARTESIAN_POINT('Ctrl Pts',(-17.7533410981157,0.967185162849705,
-1.56361188807332));
#52251=CARTESIAN_POINT('Ctrl Pts',(-17.6421947532383,1.83822846890144,-0.0352898268780593));
#52252=CARTESIAN_POINT('Ctrl Pts',(-17.5310484083608,1.0264860090507,1.52533791304877));
#52253=CARTESIAN_POINT('Ctrl Pts',(-17.4199020634834,-0.724941628214821,
1.68961205945094));
#52254=CARTESIAN_POINT('Ctrl Pts',(-17.3395713358977,-1.51113746563686,
0.690441018192311));
#52255=CARTESIAN_POINT('Ctrl Pts',(-17.2962893899378,-1.55727224070449,
0.0881329225904781));
#52256=CARTESIAN_POINT('Ctrl Pts',(-17.2900562256037,-1.55650306831887,
0.00127499959212141));
#52257=CARTESIAN_POINT('Ctrl Pts',(-17.8519437743963,-1.5562809354664,0.00132828490436524));
#52258=CARTESIAN_POINT('Ctrl Pts',(-17.8216700131418,-1.55245751151989,
-0.420686373116763));
#52259=CARTESIAN_POINT('Ctrl Pts',(-17.7543474702616,-1.15702108826059,
-1.36546780177549));
#52260=CARTESIAN_POINT('Ctrl Pts',(-17.6499761457555,0.440711752671261,
-1.78496563131869));
#52261=CARTESIAN_POINT('Ctrl Pts',(-17.5388298008781,1.73871302083308,-0.59766728630315));
#52262=CARTESIAN_POINT('Ctrl Pts',(-17.4276834560006,1.44502883098667,1.1367589153153));
#52263=CARTESIAN_POINT('Ctrl Pts',(-17.3165371111232,-0.171490898207203,
1.83055183640442));
#52264=CARTESIAN_POINT('Ctrl Pts',(-17.2246238839218,-1.37845942243566,
1.0185088936086));
#52265=CARTESIAN_POINT('Ctrl Pts',(-17.1697594383461,-1.55319539107061,
0.249859667954793));
#52266=CARTESIAN_POINT('Ctrl Pts',(-17.1519437743963,-1.55296225729592,
0.000162760582741381));
#52267=CARTESIAN_POINT('Origin',(-30.9400562256037,0.,0.));
#52268=CARTESIAN_POINT('',(-18.6900562256037,-1.55316513377742,-0.000597426394639434));
#52269=CARTESIAN_POINT('',(-18.5519437743963,-1.55723989670315,-0.000988266840771385));
#52270=CARTESIAN_POINT('',(-30.9400562256037,-1.5555,7.38654183493349E-13));
#52271=CARTESIAN_POINT('Ctrl Pts',(-18.6900562256037,-1.55316513377742,
-0.000597426394639451));
#52272=CARTESIAN_POINT('Ctrl Pts',(-18.6742081027808,-1.55393201275337,
-0.22264568371156));
#52273=CARTESIAN_POINT('Ctrl Pts',(-18.6213111983321,-1.40558222477181,
-0.962807460992807));
#52274=CARTESIAN_POINT('Ctrl Pts',(-18.5313655122577,-0.268190871892204,
-1.8189015729265));
#52275=CARTESIAN_POINT('Ctrl Pts',(-18.4202191673802,1.38280179207861,-1.21168827657323));
#52276=CARTESIAN_POINT('Ctrl Pts',(-18.3090728225028,1.76792396598735,0.504751549030178));
#52277=CARTESIAN_POINT('Ctrl Pts',(-18.1979264776254,0.534619847684823,
1.75912219422707));
#52278=CARTESIAN_POINT('Ctrl Pts',(-18.0915876119923,-1.11358239234271,
1.41852223227391));
#52279=CARTESIAN_POINT('Ctrl Pts',(-18.0222975279851,-1.55349533871507,
0.447783784135027));
#52280=CARTESIAN_POINT('Ctrl Pts',(-17.9900562256037,-1.55705119782931,
-0.00108109148358261));
#52281=CARTESIAN_POINT('Ctrl Pts',(-18.5519437743963,-1.55723989670315,
-0.000988266840771402));
#52282=CARTESIAN_POINT('Ctrl Pts',(-18.5476781511891,-1.55767973414606,
-0.0603556251486268));
#52283=CARTESIAN_POINT('Ctrl Pts',(-18.5063637463562,-1.52764743145507,
-0.634904927561926));
#52284=CARTESIAN_POINT('Ctrl Pts',(-18.4280005598975,-0.813401222257357,
-1.64885038907772));
#52285=CARTESIAN_POINT('Ctrl Pts',(-18.31685421502,0.94426823764005,-1.57755717782769));
#52286=CARTESIAN_POINT('Ctrl Pts',(-18.2057078701426,1.83751786269281,-0.0621068290635167));
#52287=CARTESIAN_POINT('Ctrl Pts',(-18.0945615252652,1.04863223837752,1.51019852422351));
#52288=CARTESIAN_POINT('Ctrl Pts',(-17.9834151803877,-0.700212082183364,
1.70000946876656));
#52289=CARTESIAN_POINT('Ctrl Pts',(-17.9025425967648,-1.5063035789731,0.705754202625275));
#52290=CARTESIAN_POINT('Ctrl Pts',(-17.8587187947676,-1.55713658650058,
0.0957717166626119));
#52291=CARTESIAN_POINT('Ctrl Pts',(-17.8519437743963,-1.5562809354664,0.00132828490436524));
#52292=CARTESIAN_POINT('Origin',(-30.9400562256037,0.,0.));
#52293=CARTESIAN_POINT('',(-19.3900562256037,-1.55486411255501,0.00139338310010585));
#52294=CARTESIAN_POINT('',(-19.2519437743963,-1.55326082343937,-0.000708567253318582));
#52295=CARTESIAN_POINT('',(-30.9400562256037,-1.5555,7.38654183493349E-13));
#52296=CARTESIAN_POINT('Ctrl Pts',(-19.3900562256037,-1.55486411255501,
0.00139338310010598));
#52297=CARTESIAN_POINT('Ctrl Pts',(-19.3631674592023,-1.55159923321925,
-0.374309611256368));
#52298=CARTESIAN_POINT('Ctrl Pts',(-19.2992299111752,-1.22614475638912,
-1.2727471902601));
#52299=CARTESIAN_POINT('Ctrl Pts',(-19.1982435815222,0.276406132535501,
-1.81767129197156));
#52300=CARTESIAN_POINT('Ctrl Pts',(-19.0870972366448,1.67709248831789,-0.75345209627986));
#52301=CARTESIAN_POINT('Ctrl Pts',(-18.9759508917673,1.5425032158592,1.0005064241797));
#52302=CARTESIAN_POINT('Ctrl Pts',(-18.8648045468899,-0.00415343528496038,
1.83856248866775));
#52303=CARTESIAN_POINT('Ctrl Pts',(-18.7695063248354,-1.32701551155171,
1.11401883828569));
#52304=CARTESIAN_POINT('Ctrl Pts',(-18.7112568844066,-1.55213924953272,
0.296445282939095));
#52305=CARTESIAN_POINT('Ctrl Pts',(-18.6900562256037,-1.55316513377742,
-0.000597426394639451));
#52306=CARTESIAN_POINT('Ctrl Pts',(-19.2519437743963,-1.55326082343937,
-0.000708567253318564));
#52307=CARTESIAN_POINT('Ctrl Pts',(-19.2366375076107,-1.55414240975036,
-0.215131833202483));
#52308=CARTESIAN_POINT('Ctrl Pts',(-19.1842824591992,-1.41270450480641,
-0.947453497569264));
#52309=CARTESIAN_POINT('Ctrl Pts',(-19.094878629162,-0.29470108811063,-1.81479487066663));
#52310=CARTESIAN_POINT('Ctrl Pts',(-18.9837322842846,1.36497537602827,-1.23173510819818));
#52311=CARTESIAN_POINT('Ctrl Pts',(-18.8725859394071,1.77510034401367,0.478902832121552));
#52312=CARTESIAN_POINT('Ctrl Pts',(-18.7614395945297,0.560229484500028,
1.75113451186034));
#52313=CARTESIAN_POINT('Ctrl Pts',(-18.6545588728594,-1.10118975965476,
1.43300616103721));
#52314=CARTESIAN_POINT('Ctrl Pts',(-18.5847269328149,-1.55385955580829,
0.45527554686127));
#52315=CARTESIAN_POINT('Ctrl Pts',(-18.5519437743963,-1.55723989670315,
-0.000988266840771402));
#52316=CARTESIAN_POINT('Origin',(-30.9400562256037,0.,0.));
#52317=CARTESIAN_POINT('',(-20.0900562256037,-1.55801011030891,-0.000227597310305756));
#52318=CARTESIAN_POINT('',(-19.9519437743963,-1.55464974635955,0.00136170718391795));
#52319=CARTESIAN_POINT('',(-30.9400562256037,-1.5555,7.38654183493349E-13));
#52320=CARTESIAN_POINT('Ctrl Pts',(-20.0900562256037,-1.55801011030891,
-0.000227597310305798));
#52321=CARTESIAN_POINT('Ctrl Pts',(-20.0891755972497,-1.55803513677739,
-0.0124678168029296));
#52322=CARTESIAN_POINT('Ctrl Pts',(-20.0512461872698,-1.55235978918751,
-0.539640640879765));
#52323=CARTESIAN_POINT('Ctrl Pts',(-19.9762679956642,-0.960110720041205,
-1.56796577801391));
#52324=CARTESIAN_POINT('Ctrl Pts',(-19.8651216507867,0.796751482021758,
-1.65695997285902));
#52325=CARTESIAN_POINT('Ctrl Pts',(-19.7539753059093,1.82423641918512,-0.229108626375055));
#52326=CARTESIAN_POINT('Ctrl Pts',(-19.6428289610319,1.18174445642581,1.40847765884577));
#52327=CARTESIAN_POINT('Ctrl Pts',(-19.5316826161545,-0.542562299135568,
1.75668876791466));
#52328=CARTESIAN_POINT('Ctrl Pts',(-19.4474250376784,-1.4731969311599,0.801563749043876));
#52329=CARTESIAN_POINT('Ctrl Pts',(-19.4002162408281,-1.55609775872762,
0.143354084664209));
#52330=CARTESIAN_POINT('Ctrl Pts',(-19.3900562256037,-1.55486411255501,
0.00139338310010598));
#52331=CARTESIAN_POINT('Ctrl Pts',(-19.9519437743963,-1.55464974635955,
0.00136170718391808));
#52332=CARTESIAN_POINT('Ctrl Pts',(-19.9255968640322,-1.55155636764689,
-0.366898958960946));
#52333=CARTESIAN_POINT('Ctrl Pts',(-19.8622011720423,-1.23656566776766,
-1.25776274828745));
#52334=CARTESIAN_POINT('Ctrl Pts',(-19.7617566984265,0.249855885875982,
-1.82151068902289));
#52335=CARTESIAN_POINT('Ctrl Pts',(-19.6506103535491,1.66592065703884,-0.777841576661194));
#52336=CARTESIAN_POINT('Ctrl Pts',(-19.5394640086717,1.55693692840167,0.977893938477322));
#52337=CARTESIAN_POINT('Ctrl Pts',(-19.4283176637942,0.0226726397870904,
1.83842734567798));
#52338=CARTESIAN_POINT('Ctrl Pts',(-19.3324775857025,-1.31820105276063,
1.12925261793028));
#52339=CARTESIAN_POINT('Ctrl Pts',(-19.2736862892365,-1.55200853222309,
0.303879161895605));
#52340=CARTESIAN_POINT('Ctrl Pts',(-19.2519437743963,-1.55326082343937,
-0.000708567253318564));
#52341=CARTESIAN_POINT('Origin',(-30.9400562256037,0.,0.));
#52342=CARTESIAN_POINT('',(-20.7900562256037,-1.55419761171519,-0.00125134276329026));
#52343=CARTESIAN_POINT('',(-20.6519437743963,-1.55804494088714,-8.79497847153243E-5));
#52344=CARTESIAN_POINT('',(-30.9400562256037,-1.5555,7.38654183493349E-13));
#52345=CARTESIAN_POINT('Ctrl Pts',(-20.7900562256037,-1.55419761171519,
-0.00125134276329025));
#52346=CARTESIAN_POINT('Ctrl Pts',(-20.7781349536712,-1.5554572697494,-0.168002024361493));
#52347=CARTESIAN_POINT('Ctrl Pts',(-20.7291649001128,-1.45391681712917,
-0.85148506976451));
#52348=CARTESIAN_POINT('Ctrl Pts',(-20.6431460649287,-0.458668949759455,
-1.78043592142131));
#52349=CARTESIAN_POINT('Ctrl Pts',(-20.5319997200512,1.24719048811815,-1.35086829932027));
#52350=CARTESIAN_POINT('Ctrl Pts',(-20.4208533751738,1.81132329283767,0.315336652776849));
#52351=CARTESIAN_POINT('Ctrl Pts',(-20.3097070302964,0.717300375240254,
1.69287018032718));
#52352=CARTESIAN_POINT('Ctrl Pts',(-20.199441313773,-1.0194963881048,1.52204881850683));
#52353=CARTESIAN_POINT('Ctrl Pts',(-20.1262243788755,-1.55698225202566,
0.502488596935498));
#52354=CARTESIAN_POINT('Ctrl Pts',(-20.0900562256037,-1.55801011030891,
-0.000227597310305798));
#52355=CARTESIAN_POINT('Ctrl Pts',(-20.6519437743963,-1.55804494088714,
-8.79497847151454E-5));
#52356=CARTESIAN_POINT('Ctrl Pts',(-20.6516050020795,-1.55804879982747,
-0.0047964033161587));
#52357=CARTESIAN_POINT('Ctrl Pts',(-20.6142174481369,-1.55589696007643,
-0.524426616553616));
#52358=CARTESIAN_POINT('Ctrl Pts',(-20.5397811125685,-0.982885979939318,
-1.55379030257311));
#52359=CARTESIAN_POINT('Ctrl Pts',(-20.4286347676911,0.772490702514734,
-1.66840860356802));
#52360=CARTESIAN_POINT('Ctrl Pts',(-20.3174884228136,1.82069938029707,-0.255700841839434));
#52361=CARTESIAN_POINT('Ctrl Pts',(-20.2063420779362,1.20216910098862,1.3910854059186));
#52362=CARTESIAN_POINT('Ctrl Pts',(-20.0951957330588,-0.516873484366524,
1.76441802164065));
#52363=CARTESIAN_POINT('Ctrl Pts',(-20.0103962985455,-1.46741867778411,
0.816918777233318));
#52364=CARTESIAN_POINT('Ctrl Pts',(-19.962645645658,-1.55590624817661,0.150945783091283));
#52365=CARTESIAN_POINT('Ctrl Pts',(-19.9519437743963,-1.55464974635955,
0.00136170718391808));
#52366=CARTESIAN_POINT('Origin',(-30.9400562256037,0.,0.));
#52367=CARTESIAN_POINT('',(-21.4900562256037,-1.55353484309772,0.000937949434483771));
#52368=CARTESIAN_POINT('',(-21.3519437743963,-1.55439271669893,-0.00130685278909096));
#52369=CARTESIAN_POINT('',(-30.9400562256037,-1.5555,7.38654183493349E-13));
#52370=CARTESIAN_POINT('Ctrl Pts',(-21.4900562256037,-1.55353484309772,
0.000937949434483658));
#52371=CARTESIAN_POINT('Ctrl Pts',(-21.4670943100927,-1.55176566897119,
-0.320590158884561));
#52372=CARTESIAN_POINT('Ctrl Pts',(-21.4070836129559,-1.29776443387202,
-1.16346243513487));
#52373=CARTESIAN_POINT('Ctrl Pts',(-21.3100241341932,0.0830160705540191,
-1.83669202856401));
#52374=CARTESIAN_POINT('Ctrl Pts',(-21.1988777893158,1.58820198952549,-0.926252512130515));
#52375=CARTESIAN_POINT('Ctrl Pts',(-21.0877314444384,1.6394860967441,0.832114544004366));
#52376=CARTESIAN_POINT('Ctrl Pts',(-20.976585099561,0.189920927787188,1.82873161424777));
#52377=CARTESIAN_POINT('Ctrl Pts',(-20.8773600266161,-1.25938071046584,
1.22392092946362));
#52378=CARTESIAN_POINT('Ctrl Pts',(-20.815183735297,-1.55154252007364,0.350223683721566));
#52379=CARTESIAN_POINT('Ctrl Pts',(-20.7900562256037,-1.55419761171519,
-0.00125134276329025));
#52380=CARTESIAN_POINT('Ctrl Pts',(-21.3519437743963,-1.55439271669893,
-0.00130685278909071));
#52381=CARTESIAN_POINT('Ctrl Pts',(-21.340564358501,-1.55565952887394,-0.160427787637493));
#52382=CARTESIAN_POINT('Ctrl Pts',(-21.2921361609799,-1.46000236816005,
-0.836123537875991));
#52383=CARTESIAN_POINT('Ctrl Pts',(-21.206659181833,-0.484597651685728,
-1.77355413503851));
#52384=CARTESIAN_POINT('Ctrl Pts',(-21.0955128369556,1.2273477973243,-1.36892166990471));
#52385=CARTESIAN_POINT('Ctrl Pts',(-20.9843664920782,1.81573138332858,0.288874882132692));
#52386=CARTESIAN_POINT('Ctrl Pts',(-20.8732201472008,0.741923909701551,
1.68222414265896));
#52387=CARTESIAN_POINT('Ctrl Pts',(-20.7624125746401,-1.00572644221501,
1.53604696707474));
#52388=CARTESIAN_POINT('Ctrl Pts',(-20.6886537837053,-1.55762677881088,
0.510128984729696));
#52389=CARTESIAN_POINT('Ctrl Pts',(-20.6519437743963,-1.55804494088714,
-8.79497847151454E-5));
#52390=CARTESIAN_POINT('Origin',(-30.9400562256037,0.,0.));
#52391=CARTESIAN_POINT('',(-22.1900562256037,-1.55760963761123,0.000745528629259664));
#52392=CARTESIAN_POINT('',(-22.0519437743963,-1.55340336122338,0.000839947947065753));
#52393=CARTESIAN_POINT('',(-30.9400562256037,-1.5555,7.38654183493349E-13));
#52394=CARTESIAN_POINT('Ctrl Pts',(-22.1900562256037,-1.55760963761123,
0.00074552862925974));
#52395=CARTESIAN_POINT('Ctrl Pts',(-22.1560536665142,-1.55481158005176,
-0.472193740327524));
#52396=CARTESIAN_POINT('Ctrl Pts',(-22.0850023257989,-1.0726145744547,-1.46538056385827));
#52397=CARTESIAN_POINT('Ctrl Pts',(-21.9769022034578,0.617417326649948,
-1.73179823319959));
#52398=CARTESIAN_POINT('Ctrl Pts',(-21.8657558585803,1.78986590745487,-0.420368063834038));
#52399=CARTESIAN_POINT('Ctrl Pts',(-21.7546095137029,1.32380169026185,1.27588336481854));
#52400=CARTESIAN_POINT('Ctrl Pts',(-21.6434631688255,-0.35412203130582,
1.80414158610255));
#52401=CARTESIAN_POINT('Ctrl Pts',(-21.5552787394591,-1.4281958244136,0.912887756867582));
#52402=CARTESIAN_POINT('Ctrl Pts',(-21.5041430917185,-1.55462021069444,
0.198191676453029));
#52403=CARTESIAN_POINT('Ctrl Pts',(-21.4900562256037,-1.55353484309772,
0.000937949434483658));
#52404=CARTESIAN_POINT('Ctrl Pts',(-22.0519437743963,-1.55340336122338,
0.00083994794706577));
#52405=CARTESIAN_POINT('Ctrl Pts',(-22.0295237149225,-1.55186430247459,
-0.313167290949957));
#52406=CARTESIAN_POINT('Ctrl Pts',(-21.970054873823,-1.30694896568139,-1.14827399755797));
#52407=CARTESIAN_POINT('Ctrl Pts',(-21.8735372510976,0.056208890351046,
-1.83770773372074));
#52408=CARTESIAN_POINT('Ctrl Pts',(-21.7623909062202,1.57451836940432,-0.949326634167536));
#52409=CARTESIAN_POINT('Ctrl Pts',(-21.6512445613427,1.65145255424892,0.808104952958591));
#52410=CARTESIAN_POINT('Ctrl Pts',(-21.5400982164653,0.216582902754202,
1.82576586674362));
#52411=CARTESIAN_POINT('Ctrl Pts',(-21.4403312874831,-1.24935076014862,
1.23897870805919));
#52412=CARTESIAN_POINT('Ctrl Pts',(-21.3776131401268,-1.55153507749042,
0.357633668376339));
#52413=CARTESIAN_POINT('Ctrl Pts',(-21.3519437743963,-1.55439271669893,
-0.00130685278909071));
#52414=CARTESIAN_POINT('Origin',(-30.9400562256037,0.,0.));
#52415=CARTESIAN_POINT('',(-22.8900562256037,-1.5557675530206,-0.00140509975720526));
#52416=CARTESIAN_POINT('',(-22.7519437743963,-1.55745576654889,0.000858804331327935));
#52417=CARTESIAN_POINT('',(-30.9400562256037,-1.5555,7.38654183493349E-13));
#52418=CARTESIAN_POINT('Ctrl Pts',(-22.8900562256037,-1.5557675530206,-0.00140509975720522));
#52419=CARTESIAN_POINT('Ctrl Pts',(-22.8820618045615,-1.55679795835249,
-0.112941593296949));
#52420=CARTESIAN_POINT('Ctrl Pts',(-22.8370186018936,-1.49496159300788,
-0.740241469970251));
#52421=CARTESIAN_POINT('Ctrl Pts',(-22.7549266175997,-0.644023257663918,
-1.72208110126926));
#52422=CARTESIAN_POINT('Ctrl Pts',(-22.6437802727223,1.09764687597715,-1.47495783377641));
#52423=CARTESIAN_POINT('Ctrl Pts',(-22.5326339278449,1.83448840962079,0.122399145126971));
#52424=CARTESIAN_POINT('Ctrl Pts',(-22.4214875829675,0.891967972949703,
1.6077071906889));
#52425=CARTESIAN_POINT('Ctrl Pts',(-22.3103412380901,-0.867094604110294,
1.6212576054667));
#52426=CARTESIAN_POINT('Ctrl Pts',(-22.2331974523021,-1.53707761145306,
0.600544227981854));
#52427=CARTESIAN_POINT('Ctrl Pts',(-22.19310244814,-1.55786031009659,0.0431152295569864));
#52428=CARTESIAN_POINT('Ctrl Pts',(-22.1900562256037,-1.55760963761123,
0.00074552862925974));
#52429=CARTESIAN_POINT('Ctrl Pts',(-22.7519437743963,-1.55745576654889,
0.000858804331327978));
#52430=CARTESIAN_POINT('Ctrl Pts',(-22.718483071344,-1.55436544988659,-0.464665174858028));
#52431=CARTESIAN_POINT('Ctrl Pts',(-22.647973586666,-1.08543011851931,-1.45103340573419));
#52432=CARTESIAN_POINT('Ctrl Pts',(-22.5404153203621,0.592083708909288,
-1.74062231273063));
#52433=CARTESIAN_POINT('Ctrl Pts',(-22.4292689754847,1.78354194798782,-0.446438432148635));
#52434=CARTESIAN_POINT('Ctrl Pts',(-22.3181226306072,1.34227658728578,1.25643253585536));
#52435=CARTESIAN_POINT('Ctrl Pts',(-22.2069762857299,-0.327760916379816,
1.80911634109733));
#52436=CARTESIAN_POINT('Ctrl Pts',(-22.1182500003262,-1.42140316864343,
0.928249222998958));
#52437=CARTESIAN_POINT('Ctrl Pts',(-22.0665724965483,-1.55440757188741,
0.205724536095963));
#52438=CARTESIAN_POINT('Ctrl Pts',(-22.0519437743963,-1.55340336122338,
0.00083994794706577));
#52439=CARTESIAN_POINT('Origin',(-30.9400562256037,0.,0.));
#52440=CARTESIAN_POINT('',(-23.5900562256037,-1.55295484690924,0.000117396959615165));
#52441=CARTESIAN_POINT('',(-23.4519437743963,-1.55599709585984,-0.00137840470682826));
#52442=CARTESIAN_POINT('',(-30.9400562256037,-1.5555,7.38654183493349E-13));
#52443=CARTESIAN_POINT('Ctrl Pts',(-23.5900562256037,-1.55295484690924,
0.000117396959615351));
#52444=CARTESIAN_POINT('Ctrl Pts',(-23.5710211609831,-1.55277522915461,
-0.266673313363955));
#52445=CARTESIAN_POINT('Ctrl Pts',(-23.5149373147366,-1.36063644227694,
-1.05297300594233));
#52446=CARTESIAN_POINT('Ctrl Pts',(-23.4218046868643,-0.111301360173381,
-1.83519516209704));
#52447=CARTESIAN_POINT('Ctrl Pts',(-23.3106583419868,1.48156975859047,-1.08870580332383));
#52448=CARTESIAN_POINT('Ctrl Pts',(-23.1995119971095,1.7181543530587,0.654427150129224));
#52449=CARTESIAN_POINT('Ctrl Pts',(-23.088365652232,0.381873692818719,1.79847206219441));
#52450=CARTESIAN_POINT('Ctrl Pts',(-22.9852137283968,-1.1827299709617,1.33225802021393));
#52451=CARTESIAN_POINT('Ctrl Pts',(-22.9191105861873,-1.55202272048022,
0.403955273988205));
#52452=CARTESIAN_POINT('Ctrl Pts',(-22.8900562256037,-1.5557675530206,-0.00140509975720522));
#52453=CARTESIAN_POINT('Ctrl Pts',(-23.4519437743963,-1.55599709585984,
-0.00137840470682786));
#52454=CARTESIAN_POINT('Ctrl Pts',(-23.4444912093914,-1.55695391316923,
-0.105315627600081));
#52455=CARTESIAN_POINT('Ctrl Pts',(-23.3999898627606,-1.50008141400989,
-0.724912339526726));
#52456=CARTESIAN_POINT('Ctrl Pts',(-23.3184397345041,-0.669080796948889,
-1.71250110688599));
#52457=CARTESIAN_POINT('Ctrl Pts',(-23.2072933896267,1.07600957223555,-1.49081606993921));
#52458=CARTESIAN_POINT('Ctrl Pts',(-23.0961470447492,1.83607896999803,0.0956199239828239));
#52459=CARTESIAN_POINT('Ctrl Pts',(-22.9850006998718,0.91533033667428,1.59452172412145));
#52460=CARTESIAN_POINT('Ctrl Pts',(-22.8738543549944,-0.843347252550528,
1.633736381901));
#52461=CARTESIAN_POINT('Ctrl Pts',(-22.7961687131692,-1.53296174585945,
0.615807054296229));
#52462=CARTESIAN_POINT('Ctrl Pts',(-22.7555318529698,-1.5577871492752,0.0507781563724314));
#52463=CARTESIAN_POINT('Ctrl Pts',(-22.7519437743963,-1.55745576654889,
0.000858804331327978));
#52464=CARTESIAN_POINT('Origin',(-30.9400562256037,0.,0.));
#52465=CARTESIAN_POINT('',(-24.2900562256037,-1.55619855523662,0.00134484759808584));
#52466=CARTESIAN_POINT('',(-24.1519437743963,-1.55294665859264,-7.17666052784641E-6));
#52467=CARTESIAN_POINT('',(-30.9400562256037,-1.5555,7.38654183493349E-13));
#52468=CARTESIAN_POINT('Ctrl Pts',(-24.2900562256037,-1.55619855523662,
0.00134484759808597));
#52469=CARTESIAN_POINT('Ctrl Pts',(-24.2599805174046,-1.55237655783788,
-0.417966273389163));
#52470=CARTESIAN_POINT('Ctrl Pts',(-24.1928560275796,-1.16125933967721,
-1.36009004702387));
#52471=CARTESIAN_POINT('Ctrl Pts',(-24.0886827561288,0.431186030422094,
-1.78729065429483));
#52472=CARTESIAN_POINT('Ctrl Pts',(-23.9775364112514,1.73550088513296,-0.606931588783731));
#52473=CARTESIAN_POINT('Ctrl Pts',(-23.866390066374,1.45107079566491,1.12903623579104));
#52474=CARTESIAN_POINT('Ctrl Pts',(-23.7552437214966,-0.161725882381191,
1.83144042074233));
#52475=CARTESIAN_POINT('Ctrl Pts',(-23.6631324412398,-1.37561804845037,
1.02411005643153));
#52476=CARTESIAN_POINT('Ctrl Pts',(-23.6080699426089,-1.55312482707299,
0.252593154260171));
#52477=CARTESIAN_POINT('Ctrl Pts',(-23.5900562256037,-1.55295484690924,
0.000117396959615351));
#52478=CARTESIAN_POINT('Ctrl Pts',(-24.1519437743963,-1.55294681014799,
-7.1762345521878E-6));
#52479=CARTESIAN_POINT('Ctrl Pts',(-24.1334505658129,-1.55295747420179,
-0.259206697087362));
#52480=CARTESIAN_POINT('Ctrl Pts',(-24.0779085756037,-1.36865343867832,
-1.03766509684273));
#52481=CARTESIAN_POINT('Ctrl Pts',(-23.9853178037686,-0.138066012129827,
-1.83337582896308));
#52482=CARTESIAN_POINT('Ctrl Pts',(-23.8741714588912,1.46552720872477,-1.11020680704943));
#52483=CARTESIAN_POINT('Ctrl Pts',(-23.7630251140138,1.7275198787737,0.629288663788884));
#52484=CARTESIAN_POINT('Ctrl Pts',(-23.6518787691364,0.408073727971786,
1.79270884040625));
#52485=CARTESIAN_POINT('Ctrl Pts',(-23.5481849892639,-1.17141938223886,
1.34704401839563));
#52486=CARTESIAN_POINT('Ctrl Pts',(-23.4815399910172,-1.55219730715134,
0.411385329884918));
#52487=CARTESIAN_POINT('Ctrl Pts',(-23.4519437743963,-1.55599709585984,
-0.00137840470682786));
#52488=CARTESIAN_POINT('Origin',(-30.9400562256037,0.,0.));
#52489=CARTESIAN_POINT('',(-24.9900562256037,-1.55730549994698,-0.000951908650860188));
#52490=CARTESIAN_POINT('',(-24.8519437743963,-1.55597074695684,0.00138208519957782));
#52491=CARTESIAN_POINT('',(-30.9400562256037,-1.5555,7.38654183493349E-13));
#52492=CARTESIAN_POINT('Ctrl Pts',(-24.9900562256037,-1.55730549994698,
-0.000951908650860013));
#52493=CARTESIAN_POINT('Ctrl Pts',(-24.9859886554519,-1.55771297063508,
-0.0575565832609528));
#52494=CARTESIAN_POINT('Ctrl Pts',(-24.9448723036742,-1.52922029296496,
-0.629320969721004));
#52495=CARTESIAN_POINT('Ctrl Pts',(-24.8667071702708,-0.822183211067854,
-1.64448899151042));
#52496=CARTESIAN_POINT('Ctrl Pts',(-24.7555608253933,0.935841500540801,
-1.58257068139984));
#52497=CARTESIAN_POINT('Ctrl Pts',(-24.644414480516,1.8371605398714,-0.071905677802479));
#52498=CARTESIAN_POINT('Ctrl Pts',(-24.5332681356385,1.05667143702865,1.50458457719352));
#52499=CARTESIAN_POINT('Ctrl Pts',(-24.4221217907611,-0.691135756872815,
1.70371964869008));
#52500=CARTESIAN_POINT('Ctrl Pts',(-24.3410511540828,-1.50450533882819,
0.711353178426976));
#52501=CARTESIAN_POINT('Ctrl Pts',(-24.2970292990304,-1.55708468793618,
0.0985624165376092));
#52502=CARTESIAN_POINT('Ctrl Pts',(-24.2900562256037,-1.55619855523662,
0.00134484759808597));
#52503=CARTESIAN_POINT('Ctrl Pts',(-24.8519437743963,-1.55597074695684,
0.00138208519957779));
#52504=CARTESIAN_POINT('Ctrl Pts',(-24.8224099222344,-1.5521757198559,-0.41052982565668));
#52505=CARTESIAN_POINT('Ctrl Pts',(-24.7558272884467,-1.17273038095177,
-1.3453445318586));
#52506=CARTESIAN_POINT('Ctrl Pts',(-24.6521958730331,0.405062575138557,
-1.79339160925706));
#52507=CARTESIAN_POINT('Ctrl Pts',(-24.5410495281557,1.72646064975028,-0.632188879050662));
#52508=CARTESIAN_POINT('Ctrl Pts',(-24.4299031832783,1.46738956291618,1.10774411511692));
#52509=CARTESIAN_POINT('Ctrl Pts',(-24.3187568384009,-0.134986946113292,
1.83360510424424));
#52510=CARTESIAN_POINT('Ctrl Pts',(-24.2261037021069,-1.36773867089657,
1.03942751774699));
#52511=CARTESIAN_POINT('Ctrl Pts',(-24.1704993474387,-1.55293611013191,
0.260066440522905));
#52512=CARTESIAN_POINT('Ctrl Pts',(-24.1519437743963,-1.55294681014799,
-7.1762345521878E-6));
#52513=CARTESIAN_POINT('Origin',(-30.9400562256037,0.,0.));
#52514=CARTESIAN_POINT('',(-25.6900562256037,-1.55329993577148,-0.000747905064743873));
#52515=CARTESIAN_POINT('',(-25.5519437743963,-1.55747437566469,-0.000846187651558084));
#52516=CARTESIAN_POINT('',(-30.9400562256037,-1.5555,7.38654183493349E-13));
#52517=CARTESIAN_POINT('Ctrl Pts',(-25.6900562256037,-1.55329993577148,
-0.000747905064743624));
#52518=CARTESIAN_POINT('Ctrl Pts',(-25.6749480118734,-1.55421977858412,
-0.21238335774611));
#52519=CARTESIAN_POINT('Ctrl Pts',(-25.6227910165173,-1.41527094711558,
-0.941840467750138));
#52520=CARTESIAN_POINT('Ctrl Pts',(-25.5335852395354,-0.304375448471892,
-1.81319741399803));
#52521=CARTESIAN_POINT('Ctrl Pts',(-25.4224388946579,1.35838697931157,-1.23899721153737));
#52522=CARTESIAN_POINT('Ctrl Pts',(-25.3112925497805,1.77762918529204,0.469429180344255));
#52523=CARTESIAN_POINT('Ctrl Pts',(-25.200146204903,0.569560564207642,1.74812186058649));
#52524=CARTESIAN_POINT('Ctrl Pts',(-25.0930674301775,-1.09661346171798,
1.43828552764103));
#52525=CARTESIAN_POINT('Ctrl Pts',(-25.0230374370777,-1.55400159210223,
0.458017617145497));
#52526=CARTESIAN_POINT('Ctrl Pts',(-24.9900562256037,-1.55730549994698,
-0.000951908650860013));
#52527=CARTESIAN_POINT('Ctrl Pts',(-25.5519437743963,-1.55747437566469,
-0.000846187651558162));
#52528=CARTESIAN_POINT('Ctrl Pts',(-25.5484180602817,-1.55779615002965,
-0.0498963460263509));
#52529=CARTESIAN_POINT('Ctrl Pts',(-25.5078435645413,-1.53344150154939,
-0.614049915219279));
#52530=CARTESIAN_POINT('Ctrl Pts',(-25.4302202871752,-0.846089671080599,
-1.63231780680796));
#52531=CARTESIAN_POINT('Ctrl Pts',(-25.3190739422977,0.912651293186798,
-1.59605663150652));
#52532=CARTESIAN_POINT('Ctrl Pts',(-25.2079275974203,1.83591580205738,-0.0987031999860136));
#52533=CARTESIAN_POINT('Ctrl Pts',(-25.0967812525428,1.07851165011462,1.48900697597377));
#52534=CARTESIAN_POINT('Ctrl Pts',(-24.9856349076655,-0.666203972560349,
1.7136223098677));
#52535=CARTESIAN_POINT('Ctrl Pts',(-24.9040224149499,-1.4994986854534,0.726676294106424));
#52536=CARTESIAN_POINT('Ctrl Pts',(-24.8594587038602,-1.55693639684298,
0.10619363969844));
#52537=CARTESIAN_POINT('Ctrl Pts',(-24.8519437743963,-1.55597074695684,
0.00138208519957779));
#52538=CARTESIAN_POINT('Origin',(-30.9400562256037,0.,0.));
#52539=CARTESIAN_POINT('',(-26.3900562256037,-1.55457327774435,0.00134739417963825));
#52540=CARTESIAN_POINT('',(-26.2519437743963,-1.5534177173597,-0.000851565729181603));
#52541=CARTESIAN_POINT('',(-30.9400562256037,-1.5555,7.38654183493349E-13));
#52542=CARTESIAN_POINT('Ctrl Pts',(-26.3900562256037,-1.55457327774435,
0.00134739417963841));
#52543=CARTESIAN_POINT('Ctrl Pts',(-26.3639073682949,-1.55154654523881,
-0.364190570873877));
#52544=CARTESIAN_POINT('Ctrl Pts',(-26.3007097293602,-1.2403310165763,-1.25227730661038));
#52545=CARTESIAN_POINT('Ctrl Pts',(-26.2004633087999,0.240137974670818,
-1.8228173328443));
#52546=CARTESIAN_POINT('Ctrl Pts',(-26.0893169639224,1.66174866141038,-0.786715108572567));
#52547=CARTESIAN_POINT('Ctrl Pts',(-25.978170619045,1.56213005525038,0.969576694355506));
#52548=CARTESIAN_POINT('Ctrl Pts',(-25.8670242741676,0.032476899015307,
1.8382803177961));
#52549=CARTESIAN_POINT('Ctrl Pts',(-25.7709861430205,-1.3149385586997,1.13481601539216));
#52550=CARTESIAN_POINT('Ctrl Pts',(-25.7119967934992,-1.55196411447294,
0.306594981495643));
#52551=CARTESIAN_POINT('Ctrl Pts',(-25.6900562256037,-1.55329993577148,
-0.000747905064743624));
#52552=CARTESIAN_POINT('Ctrl Pts',(-26.2519437743963,-1.5534177173597,-0.00085156572918162));
#52553=CARTESIAN_POINT('Ctrl Pts',(-26.2373774167032,-1.55443203746226,
-0.204857978458031));
#52554=CARTESIAN_POINT('Ctrl Pts',(-26.1857622773843,-1.42219235049638,
-0.926481326314944));
#52555=CARTESIAN_POINT('Ctrl Pts',(-26.0970983564397,-0.330798585473345,
-1.80856336626222));
#52556=CARTESIAN_POINT('Ctrl Pts',(-25.9859520115622,1.340164710296,-1.25868491021684));
#52557=CARTESIAN_POINT('Ctrl Pts',(-25.8748056666848,1.78428915735557,0.443442619595842));
#52558=CARTESIAN_POINT('Ctrl Pts',(-25.7636593218074,0.595005980146546,
1.7396255452028));
#52559=CARTESIAN_POINT('Ctrl Pts',(-25.6560386910445,-1.08396473869043,
1.4526878959));
#52560=CARTESIAN_POINT('Ctrl Pts',(-25.5854668419075,-1.55441489227795,
0.465530755344284));
#52561=CARTESIAN_POINT('Ctrl Pts',(-25.5519437743963,-1.55747437566469,
-0.000846187651558162));
#52562=CARTESIAN_POINT('Origin',(-30.9400562256037,0.,0.));
#52563=CARTESIAN_POINT('',(-27.0900562256037,-1.5580501213287,-3.65571210202475E-5));
#52564=CARTESIAN_POINT('',(-26.9519437743963,-1.55436975637195,0.00130097926851286));
#52565=CARTESIAN_POINT('',(-30.9400562256037,-1.5555,7.38654183493349E-13));
#52566=CARTESIAN_POINT('Ctrl Pts',(-27.0900562256037,-1.5580501213287,-3.65571210204235E-5));
#52567=CARTESIAN_POINT('Ctrl Pts',(-27.0899155063422,-1.55805079701309,
-0.00199233735013099));
#52568=CARTESIAN_POINT('Ctrl Pts',(-27.0527260054549,-1.55716171500239,
-0.518868284418442));
#52569=CARTESIAN_POINT('Ctrl Pts',(-26.9784877229418,-0.991158593083783,
-1.54852636916561));
#52570=CARTESIAN_POINT('Ctrl Pts',(-26.8673413780644,0.763581882211757,
-1.67250470444365));
#52571=CARTESIAN_POINT('Ctrl Pts',(-26.756195033187,1.81930983338734,-0.265407245427431));
#52572=CARTESIAN_POINT('Ctrl Pts',(-26.6450486883096,1.20957087255313,1.38465431773148));
#52573=CARTESIAN_POINT('Ctrl Pts',(-26.5339023434321,-0.507456263538371,
1.76714951732695));
#52574=CARTESIAN_POINT('Ctrl Pts',(-26.4489048558636,-1.4652729107266,0.82253205856728));
#52575=CARTESIAN_POINT('Ctrl Pts',(-26.4009561499207,-1.55583494493112,
0.153718723718826));
#52576=CARTESIAN_POINT('Ctrl Pts',(-26.3900562256037,-1.55457327774435,
0.00134739417963841));
#52577=CARTESIAN_POINT('Ctrl Pts',(-26.9519437743963,-1.55436975637195,
0.00130097926851296));
#52578=CARTESIAN_POINT('Ctrl Pts',(-26.9263367731247,-1.55153485082019,
-0.356780851543248));
#52579=CARTESIAN_POINT('Ctrl Pts',(-26.8636809902274,-1.25051393155525,
-1.23724720927912));
#52580=CARTESIAN_POINT('Ctrl Pts',(-26.7639764257042,0.213516505753145,
-1.82612700980389));
#52581=CARTESIAN_POINT('Ctrl Pts',(-26.6528300808268,1.65009313818133,-0.810877172722089));
#52582=CARTESIAN_POINT('Ctrl Pts',(-26.5416837359494,1.5761103965168,0.946681135265884));
#52583=CARTESIAN_POINT('Ctrl Pts',(-26.4305373910719,0.0592949571880597,
1.83761074823246));
#52584=CARTESIAN_POINT('Ctrl Pts',(-26.3339574038876,-1.30590031967722,
1.15002320221466));
#52585=CARTESIAN_POINT('Ctrl Pts',(-26.274426198329,-1.55185216644918,0.314021840005712));
#52586=CARTESIAN_POINT('Ctrl Pts',(-26.2519437743963,-1.5534177173597,-0.00085156572918162));
#52587=CARTESIAN_POINT('Origin',(-30.9400562256037,0.,0.));
#52588=CARTESIAN_POINT('',(-27.7900562256037,-1.55446647382692,-0.00132458884794142));
#52589=CARTESIAN_POINT('',(-27.6519437743963,-1.55804245891508,0.000104104215403816));
#52590=CARTESIAN_POINT('',(-30.9400562256037,-1.5555,7.38654183493349E-13));
#52591=CARTESIAN_POINT('Ctrl Pts',(-27.7900562256037,-1.55446647382692,
-0.00132458884794144));
#52592=CARTESIAN_POINT('Ctrl Pts',(-27.7788748627637,-1.5557324439126,-0.157657369512062));
#52593=CARTESIAN_POINT('Ctrl Pts',(-27.730644718298,-1.46219237042214,-0.830509405833625));
#52594=CARTESIAN_POINT('Ctrl Pts',(-27.6453657922064,-0.494049365075557,
-1.77094447718388));
#52595=CARTESIAN_POINT('Ctrl Pts',(-27.534219447329,1.22002971701301,-1.37544786085574));
#52596=CARTESIAN_POINT('Ctrl Pts',(-27.4230731024515,1.81724620484857,0.279187250412826));
#52597=CARTESIAN_POINT('Ctrl Pts',(-27.3119267575741,0.750884899378822,
1.67824346299867));
#52598=CARTESIAN_POINT('Ctrl Pts',(-27.2009211319582,-1.00064524107714,
1.54114421983883));
#52599=CARTESIAN_POINT('Ctrl Pts',(-27.126964287968,-1.55787290179637,0.512928462058482));
#52600=CARTESIAN_POINT('Ctrl Pts',(-27.0900562256037,-1.5580501213287,-3.65571210204235E-5));
#52601=CARTESIAN_POINT('Ctrl Pts',(-27.6519437743963,-1.55804245891508,
0.000104104215403655));
#52602=CARTESIAN_POINT('Ctrl Pts',(-27.6152961295462,-1.5575504591777,-0.509248245460903));
#52603=CARTESIAN_POINT('Ctrl Pts',(-27.5415997030704,-1.00732110649725,
-1.53443975582773));
#52604=CARTESIAN_POINT('Ctrl Pts',(-27.4308544949688,0.739097826986148,
-1.68346772023046));
#52605=CARTESIAN_POINT('Ctrl Pts',(-27.3197081500913,1.81524370282257,-0.291923713345362));
#52606=CARTESIAN_POINT('Ctrl Pts',(-27.2085618052139,1.22964495869491,1.36685859779542));
#52607=CARTESIAN_POINT('Ctrl Pts',(-27.0974154603365,-0.48161855815431,
1.77436544145867));
#52608=CARTESIAN_POINT('Ctrl Pts',(-27.0118761167306,-1.45930897725486,
0.83789144882417));
#52609=CARTESIAN_POINT('Ctrl Pts',(-26.9633855547505,-1.55563645551818,
0.161299942581343));
#52610=CARTESIAN_POINT('Ctrl Pts',(-26.9519437743963,-1.55436975637195,
0.00130097926851296));
#52611=CARTESIAN_POINT('Origin',(-30.9400562256037,0.,0.));
#52612=CARTESIAN_POINT('',(-28.4900562256037,-1.55335883765056,0.000804378038691873));
#52613=CARTESIAN_POINT('',(-28.3519437743963,-1.55467403768283,-0.00136587788398465));
#52614=CARTESIAN_POINT('',(-30.9400562256037,-1.5555,7.38654183493349E-13));
#52615=CARTESIAN_POINT('Ctrl Pts',(-28.4900562256037,-1.55335883765056,
0.000804378038691943));
#52616=CARTESIAN_POINT('Ctrl Pts',(-28.4678342191853,-1.5519039872972,-0.310451991356807));
#52617=CARTESIAN_POINT('Ctrl Pts',(-28.408563431141,-1.31026523547163,-1.14272024251096));
#52618=CARTESIAN_POINT('Ctrl Pts',(-28.3122438614709,0.046407699775919,
-1.83797936794685));
#52619=CARTESIAN_POINT('Ctrl Pts',(-28.2010975165935,1.56943293437681,-0.95771133892945));
#52620=CARTESIAN_POINT('Ctrl Pts',(-28.089951171716,1.65573892814966,0.799286617882397));
#52621=CARTESIAN_POINT('Ctrl Pts',(-27.9788048268387,0.226316831424914,
1.82458457360074));
#52622=CARTESIAN_POINT('Ctrl Pts',(-27.8788398448012,-1.24564163566608,
1.24447484849783));
#52623=CARTESIAN_POINT('Ctrl Pts',(-27.8159236443895,-1.55153772722909,
0.360342013449946));
#52624=CARTESIAN_POINT('Ctrl Pts',(-27.7900562256037,-1.55446647382692,
-0.00132458884794144));
#52625=CARTESIAN_POINT('Ctrl Pts',(-28.3519437743963,-1.55467403768283,
-0.0013658778839847));
#52626=CARTESIAN_POINT('Ctrl Pts',(-28.3413042675936,-1.55592857918768,
-0.150072444919674));
#52627=CARTESIAN_POINT('Ctrl Pts',(-28.293615979165,-1.46809072386952,-0.815151663224704));
#52628=CARTESIAN_POINT('Ctrl Pts',(-28.2088789091108,-0.519835724455463,
-1.76354724094302));
#52629=CARTESIAN_POINT('Ctrl Pts',(-28.0977325642333,1.19983124114152,-1.39310245061395));
#52630=CARTESIAN_POINT('Ctrl Pts',(-27.9865862193559,1.82112625016851,0.252642976453954));
#52631=CARTESIAN_POINT('Ctrl Pts',(-27.8754398744784,0.775291433296788,
1.66710893100567));
#52632=CARTESIAN_POINT('Ctrl Pts',(-27.764293529601,-0.980275235800491,
1.55543873831543));
#52633=CARTESIAN_POINT('Ctrl Pts',(-27.6897948295736,-1.55549560212386,
0.526177148100607));
#52634=CARTESIAN_POINT('Ctrl Pts',(-27.6523449111721,-1.55804784423217,
0.00567935905418177));
#52635=CARTESIAN_POINT('Ctrl Pts',(-27.6519437743963,-1.55804245891508,
0.000104104215403655));
#52636=CARTESIAN_POINT('Origin',(-30.9400562256037,0.,0.));
#52637=CARTESIAN_POINT('',(-29.1900562256037,-1.55737653422887,0.00100621910560842));
#52638=CARTESIAN_POINT('',(-29.0519437743963,-1.55324480116086,0.000708030066551985));
#52639=CARTESIAN_POINT('',(-30.9400562256037,-1.5555,7.38654183493349E-13));
#52640=CARTESIAN_POINT('Ctrl Pts',(-29.1900562256037,-1.55737653422887,
0.00100621910560853));
#52641=CARTESIAN_POINT('Ctrl Pts',(-29.1567935756068,-1.55418812333816,
-0.461781077921097));
#52642=CARTESIAN_POINT('Ctrl Pts',(-29.086482143984,-1.09009726042822,-1.44594760124546));
#52643=CARTESIAN_POINT('Ctrl Pts',(-28.9791219307355,0.582808968573894,
-1.74365887083216));
#52644=CARTESIAN_POINT('Ctrl Pts',(-28.867975585858,1.78112695043666,-0.455994626000207));
#52645=CARTESIAN_POINT('Ctrl Pts',(-28.7568292409806,1.34896284622222,1.24928278177877));
#52646=CARTESIAN_POINT('Ctrl Pts',(-28.6456828961032,-0.318110417184717,
1.81082463803951));
#52647=CARTESIAN_POINT('Ctrl Pts',(-28.5567585576442,-1.41888362636568,
0.933866456267556));
#52648=CARTESIAN_POINT('Ctrl Pts',(-28.5048830008111,-1.55432953033886,
0.208478164733725));
#52649=CARTESIAN_POINT('Ctrl Pts',(-28.4900562256037,-1.55335883765056,
0.000804378038691943));
#52650=CARTESIAN_POINT('Ctrl Pts',(-29.0519437743963,-1.55324480116087,
0.00070803006655188));
#52651=CARTESIAN_POINT('Ctrl Pts',(-29.0302636240151,-1.55202060661361,
-0.303017220285967));
#52652=CARTESIAN_POINT('Ctrl Pts',(-28.971534692008,-1.31923084685054,-1.12752040336955));
#52653=CARTESIAN_POINT('Ctrl Pts',(-28.8757569783753,0.0195899148733162,
-1.83844939731259));
#52654=CARTESIAN_POINT('Ctrl Pts',(-28.7646106334978,1.55529006052317,-0.980514255533821));
#52655=CARTESIAN_POINT('Ctrl Pts',(-28.6534642886204,1.6672258610176,0.775046535726967));
#52656=CARTESIAN_POINT('Ctrl Pts',(-28.542317943743,0.252913801877688,1.82108657460817));
#52657=CARTESIAN_POINT('Ctrl Pts',(-28.4418111056683,-1.23537493202417,
1.25948986433566));
#52658=CARTESIAN_POINT('Ctrl Pts',(-28.3783530492194,-1.55156002760766,
0.367752039860246));
#52659=CARTESIAN_POINT('Ctrl Pts',(-28.3519437743963,-1.55467403768283,
-0.0013658778839847));
#52660=CARTESIAN_POINT('Origin',(-0.2,2.59090492670967E-16,0.));
#52661=CARTESIAN_POINT('',(-0.2,0.0853826423430817,1.95213365433479));
#52662=CARTESIAN_POINT('Ctrl Pts',(-0.200000000000004,1.33821259954893,
-0.797996165557001));
#52663=CARTESIAN_POINT('Ctrl Pts',(-0.200000000000003,1.36083146673087,
-0.769266098091291));
#52664=CARTESIAN_POINT('Ctrl Pts',(-0.199999999999999,1.38232620666805,
-0.739737377686227));
#52665=CARTESIAN_POINT('Ctrl Pts',(-0.199999999999999,1.40263605993815,
-0.709452586790428));
#52666=CARTESIAN_POINT('Ctrl Pts',(-0.2,1.43566749400714,-0.660198165280631));
#52667=CARTESIAN_POINT('Ctrl Pts',(-0.199999999999991,1.46556712027168,
-0.608945988984861));
#52668=CARTESIAN_POINT('Ctrl Pts',(-0.199999999999987,1.49239176656985,
-0.556021150339029));
#52669=CARTESIAN_POINT('Ctrl Pts',(-0.199999999999985,1.50784007518276,
-0.525541746003136));
#52670=CARTESIAN_POINT('Ctrl Pts',(-0.199999999999994,1.52226790514226,
-0.494506807866819));
#52671=CARTESIAN_POINT('Ctrl Pts',(-0.199999999999996,1.53568068894636,
-0.462973130619356));
#52672=CARTESIAN_POINT('Ctrl Pts',(-0.199999999999997,1.54263081553624,
-0.446633267700872));
#52673=CARTESIAN_POINT('Ctrl Pts',(-0.199999999999989,1.54930985473548,
-0.4301550048461));
#52674=CARTESIAN_POINT('Ctrl Pts',(-0.199999999999989,1.55570791547876,
-0.413573830206026));
#52675=CARTESIAN_POINT('Ctrl Pts',(-0.199999999999988,1.57814412154956,
-0.355428297356665));
#52676=CARTESIAN_POINT('Ctrl Pts',(-0.199999999999984,1.59715451942584,
-0.295963114431022));
#52677=CARTESIAN_POINT('Ctrl Pts',(-0.199999999999987,1.6127982700493,-0.235533509212285));
#52678=CARTESIAN_POINT('Ctrl Pts',(-0.19999999999999,1.62482864572664,-0.189061862462472));
#52679=CARTESIAN_POINT('Ctrl Pts',(-0.199999999999983,1.63486727068506,
-0.142018843352932));
#52680=CARTESIAN_POINT('Ctrl Pts',(-0.199999999999983,1.64292447455769,
-0.0945533019233128));
#52681=CARTESIAN_POINT('Ctrl Pts',(-0.199999999999983,1.64689952531549,
-0.0711360048793496));
#52682=CARTESIAN_POINT('Ctrl Pts',(-0.199999999999985,1.65039207440413,
-0.047615726128019));
#52683=CARTESIAN_POINT('Ctrl Pts',(-0.199999999999984,1.65340199272743,
-0.0240096709125676));
#52684=CARTESIAN_POINT('Ctrl Pts',(-0.199999999999984,1.65494614856356,
-0.0118992333479225));
#52685=CARTESIAN_POINT('Ctrl Pts',(-0.199999999999997,1.65636206949049,
0.000224531212346389));
#52686=CARTESIAN_POINT('Ctrl Pts',(-0.199999999999996,1.65765003815761,
0.0123570392677572));
#52687=CARTESIAN_POINT('Ctrl Pts',(-0.199999999999995,1.66448973811924,
0.0767861802857205));
#52688=CARTESIAN_POINT('Ctrl Pts',(-0.199999999999997,1.66772693008277,
0.141478210488262));
#52689=CARTESIAN_POINT('Ctrl Pts',(-0.199999999999996,1.6674177087189,0.206071916622556));
#52690=CARTESIAN_POINT('Ctrl Pts',(-0.199999999999995,1.66710248839164,
0.271918755053447));
#52691=CARTESIAN_POINT('Ctrl Pts',(-0.199999999999987,1.66310228737439,
0.337664448069482));
#52692=CARTESIAN_POINT('Ctrl Pts',(-0.199999999999986,1.65542859034139,
0.402950019404703));
#52693=CARTESIAN_POINT('Ctrl Pts',(-0.199999999999985,1.65047305117389,
0.445110298137822));
#52694=CARTESIAN_POINT('Ctrl Pts',(-0.199999999999992,1.64398454736424,
0.487079135065034));
#52695=CARTESIAN_POINT('Ctrl Pts',(-0.199999999999993,1.63595477654208,
0.528761747087024));
#52696=CARTESIAN_POINT('Ctrl Pts',(-0.199999999999993,1.6314372854833,0.552212083502153));
#52697=CARTESIAN_POINT('Ctrl Pts',(-0.199999999999989,1.62643180252044,
0.575571836727543));
#52698=CARTESIAN_POINT('Ctrl Pts',(-0.199999999999988,1.62093554824454,
0.598824048775656));
#52699=CARTESIAN_POINT('Ctrl Pts',(-0.199999999999988,1.61825461164952,
0.610165901438495));
#52700=CARTESIAN_POINT('Ctrl Pts',(-0.199999999999994,1.61545644305892,
0.621483904474924));
#52701=CARTESIAN_POINT('Ctrl Pts',(-0.199999999999994,1.61254205914868,
0.632770588829928));
#52702=CARTESIAN_POINT('Ctrl Pts',(-0.199999999999993,1.59558819313177,
0.698428697103724));
#52703=CARTESIAN_POINT('Ctrl Pts',(-0.199999999999995,1.57477263017097,
0.762771028666577));
#52704=CARTESIAN_POINT('Ctrl Pts',(-0.199999999999997,1.55012986044755,
0.82542185568922));
#52705=CARTESIAN_POINT('Ctrl Pts',(-0.199999999999998,1.54138328915035,
0.847658801111062));
#52706=CARTESIAN_POINT('Ctrl Pts',(-0.199999999999995,1.5321541065797,0.86968277159213));
#52707=CARTESIAN_POINT('Ctrl Pts',(-0.199999999999995,1.52244229463082,
0.891477201154086));
#52708=CARTESIAN_POINT('Ctrl Pts',(-0.199999999999995,1.49604924959517,
0.950706247596028));
#52709=CARTESIAN_POINT('Ctrl Pts',(-0.199999999999994,1.4660955787197,1.00824097839801));
#52710=CARTESIAN_POINT('Ctrl Pts',(-0.199999999999996,1.43287445271699,
1.06395280437091));
#52711=CARTESIAN_POINT('Ctrl Pts',(-0.199999999999997,1.41494791261197,
1.09401561086777));
#52712=CARTESIAN_POINT('Ctrl Pts',(-0.199999999999993,1.39606904617647,
1.123547433112));
#52713=CARTESIAN_POINT('Ctrl Pts',(-0.199999999999994,1.37627808156598,
1.15252619254564));
#52714=CARTESIAN_POINT('Ctrl Pts',(-0.199999999999995,1.3622243467481,1.17310425978223));
#52715=CARTESIAN_POINT('Ctrl Pts',(-0.199999999999992,1.34771059846554,
1.19340341412927));
#52716=CARTESIAN_POINT('Ctrl Pts',(-0.199999999999993,1.3327501250156,1.21341519986235));
#52717=CARTESIAN_POINT('Ctrl Pts',(-0.199999999999993,1.32597618088804,
1.22247632475938));
#52718=CARTESIAN_POINT('Ctrl Pts',(-0.199999999999993,1.31910926376118,
1.23148028792388));
#52719=CARTESIAN_POINT('Ctrl Pts',(-0.199999999999993,1.31215500866612,
1.24042055272821));
#52720=CARTESIAN_POINT('Ctrl Pts',(-0.199999999999992,1.27060407929176,
1.29383767740876));
#52721=CARTESIAN_POINT('Ctrl Pts',(-0.199999999999984,1.22606300839517,
1.3448257906629));
#52722=CARTESIAN_POINT('Ctrl Pts',(-0.199999999999985,1.17887277817311,
1.39325604164226));
#52723=CARTESIAN_POINT('Ctrl Pts',(-0.199999999999986,1.13064656854509,
1.44274949452599));
#52724=CARTESIAN_POINT('Ctrl Pts',(-0.199999999999989,1.07965311599888,
1.48957227465749));
#52725=CARTESIAN_POINT('Ctrl Pts',(-0.199999999999988,1.02620391534963,
1.5335686727213));
#52726=CARTESIAN_POINT('Ctrl Pts',(-0.199999999999988,0.97226644704798,
1.57796698545803));
#52727=CARTESIAN_POINT('Ctrl Pts',(-0.199999999999996,0.915827484062048,
1.61948781404837));
#52728=CARTESIAN_POINT('Ctrl Pts',(-0.199999999999996,0.857163347037397,
1.65794145013127));
#52729=CARTESIAN_POINT('Ctrl Pts',(-0.199999999999997,0.834333137919339,
1.67290637755794));
#52730=CARTESIAN_POINT('Ctrl Pts',(-0.200000000000002,0.81116551130864,
1.68740639452663));
#52731=CARTESIAN_POINT('Ctrl Pts',(-0.200000000000001,0.787675332375756,
1.70142872353338));
#52732=CARTESIAN_POINT('Ctrl Pts',(-0.200000000000001,0.778712552141178,
1.70677900433045));
#52733=CARTESIAN_POINT('Ctrl Pts',(-0.199999999999995,0.769704701380117,
1.71205854430649));
#52734=CARTESIAN_POINT('Ctrl Pts',(-0.199999999999995,0.760660445012377,
1.71726235891511));
#52735=CARTESIAN_POINT('Ctrl Pts',(-0.199999999999992,0.698085449280864,
1.75326627827364));
#52736=CARTESIAN_POINT('Ctrl Pts',(-0.19999999999998,0.633667777713838,
1.78570985411892));
#52737=CARTESIAN_POINT('Ctrl Pts',(-0.199999999999981,0.567740838726636,
1.81443271252908));
#52738=CARTESIAN_POINT('Ctrl Pts',(-0.199999999999982,0.501663825842382,
1.84322095470136));
#52739=CARTESIAN_POINT('Ctrl Pts',(-0.199999999999981,0.434069865483067,
1.86827227177555));
#52740=CARTESIAN_POINT('Ctrl Pts',(-0.199999999999979,0.365255754338618,
1.88939040512503));
#52741=CARTESIAN_POINT('Ctrl Pts',(-0.199999999999978,0.297913662913918,
1.91005679524601));
#52742=CARTESIAN_POINT('Ctrl Pts',(-0.199999999999988,0.229402198343265,
1.92695702889807));
#52743=CARTESIAN_POINT('Ctrl Pts',(-0.199999999999987,0.159974824830696,
1.93986449335383));
#52744=CARTESIAN_POINT('Ctrl Pts',(-0.199999999999987,0.135223669558322,
1.94446605957698));
#52745=CARTESIAN_POINT('Ctrl Pts',(-0.199999999999991,0.110355935852113,
1.9485597226482));
#52746=CARTESIAN_POINT('Ctrl Pts',(-0.199999999999991,0.0853826423429707,
1.9521336543348));
#52747=CARTESIAN_POINT('',(-0.200000000000025,-1.49576935231745,1.26229836271313));
#52748=CARTESIAN_POINT('Origin',(-0.2,0.,0.));
#52749=CARTESIAN_POINT('Ctrl Pts',(-0.199999999999997,-1.49578438409795,
1.26230645381927));
#52750=CARTESIAN_POINT('Ctrl Pts',(-0.199999999999997,-1.52168996012369,
1.22501433090188));
#52751=CARTESIAN_POINT('Ctrl Pts',(-0.199999999999991,-1.5461641556753,
1.18681013346276));
#52752=CARTESIAN_POINT('Ctrl Pts',(-0.199999999999995,-1.5691243985238,
1.14772495209047));
#52753=CARTESIAN_POINT('Ctrl Pts',(-0.199999999999999,-1.60551023262156,
1.08578541014067));
#52754=CARTESIAN_POINT('Ctrl Pts',(-0.199999999999998,-1.63809649512831,
1.02163357061851));
#52755=CARTESIAN_POINT('Ctrl Pts',(-0.199999999999997,-1.6668721870644,
0.955646304386221));
#52756=CARTESIAN_POINT('Ctrl Pts',(-0.199999999999997,-1.68055611898491,
0.924266858819843));
#52757=CARTESIAN_POINT('Ctrl Pts',(-0.199999999999998,-1.69337759315812,
0.892472194507605));
#52758=CARTESIAN_POINT('Ctrl Pts',(-0.199999999999999,-1.70533138078191,
0.860302523849142));
#52759=CARTESIAN_POINT('Ctrl Pts',(-0.199999999999999,-1.71156562096785,
0.843525125764171));
#52760=CARTESIAN_POINT('Ctrl Pts',(-0.200000000000005,-1.71756381466397,
0.826645730493394));
#52761=CARTESIAN_POINT('Ctrl Pts',(-0.200000000000006,-1.72332494158841,
0.809670073695925));
#52762=CARTESIAN_POINT('Ctrl Pts',(-0.200000000000007,-1.72807906609128,
0.795661636285706));
#52763=CARTESIAN_POINT('Ctrl Pts',(-0.2,-1.73266865506746,0.781596710180168));
#52764=CARTESIAN_POINT('Ctrl Pts',(-0.200000000000001,-1.73709291763167,
0.767481383246849));
#52765=CARTESIAN_POINT('Ctrl Pts',(-0.200000000000004,-1.75844509037697,
0.699358640832162));
#52766=CARTESIAN_POINT('Ctrl Pts',(-0.200000000000006,-1.77595779613622,
0.63004133653378));
#52767=CARTESIAN_POINT('Ctrl Pts',(-0.200000000000013,-1.78961532543345,
0.5599012489287));
#52768=CARTESIAN_POINT('Ctrl Pts',(-0.200000000000018,-1.79936972654671,
0.509806203644238));
#52769=CARTESIAN_POINT('Ctrl Pts',(-0.200000000000009,-1.80715648654673,
0.459291207712322));
#52770=CARTESIAN_POINT('Ctrl Pts',(-0.200000000000011,-1.81295369990729,
0.408493543644497));
#52771=CARTESIAN_POINT('Ctrl Pts',(-0.200000000000012,-1.81629536353796,
0.379212457029137));
#52772=CARTESIAN_POINT('Ctrl Pts',(-0.200000000000004,-1.8189757195653,
0.349837501668433));
#52773=CARTESIAN_POINT('Ctrl Pts',(-0.200000000000005,-1.8209885736095,
0.320395678757213));
#52774=CARTESIAN_POINT('Ctrl Pts',(-0.200000000000006,-1.82184695550393,
0.30784020917476));
#52775=CARTESIAN_POINT('Ctrl Pts',(-0.199999999999998,-1.822583285484,0.295281755485384));
#52776=CARTESIAN_POINT('Ctrl Pts',(-0.199999999999999,-1.82319746824128,
0.282724832221508));
#52777=CARTESIAN_POINT('Ctrl Pts',(-0.200000000000001,-1.82659875079537,
0.21318584968782));
#52778=CARTESIAN_POINT('Ctrl Pts',(-0.200000000000006,-1.82625986266907,
0.14366821824979));
#52779=CARTESIAN_POINT('Ctrl Pts',(-0.200000000000005,-1.82216318737456,
0.0745161284520812));
#52780=CARTESIAN_POINT('Ctrl Pts',(-0.200000000000004,-1.8181675098021,
0.00706888540006578));
#52781=CARTESIAN_POINT('Ctrl Pts',(-0.199999999999997,-1.81059674010245,
-0.0600315443553361));
#52782=CARTESIAN_POINT('Ctrl Pts',(-0.199999999999997,-1.79938824077835,
-0.126450987847281));
#52783=CARTESIAN_POINT('Ctrl Pts',(-0.199999999999997,-1.79202556984101,
-0.170080780929468));
#52784=CARTESIAN_POINT('Ctrl Pts',(-0.199999999999998,-1.7830923059571,
-0.213416399555303));
#52785=CARTESIAN_POINT('Ctrl Pts',(-0.199999999999999,-1.77256029454147,
-0.256356695069847));
#52786=CARTESIAN_POINT('Ctrl Pts',(-0.2,-1.76373011398598,-0.292358418533345));
#52787=CARTESIAN_POINT('Ctrl Pts',(-0.199999999999999,-1.75377596763092,
-0.328082194465782));
#52788=CARTESIAN_POINT('Ctrl Pts',(-0.199999999999999,-1.74267690704633,
-0.363464633981315));
#52789=CARTESIAN_POINT('Ctrl Pts',(-0.199999999999999,-1.73916265124264,
-0.374667649089508));
#52790=CARTESIAN_POINT('Ctrl Pts',(-0.200000000000003,-1.73553328373527,
-0.385837013750726));
#52791=CARTESIAN_POINT('Ctrl Pts',(-0.200000000000003,-1.73179339095667,
-0.39695567446876));
#52792=CARTESIAN_POINT('Ctrl Pts',(-0.200000000000004,-1.71101919172734,
-0.458717143739095));
#52793=CARTESIAN_POINT('Ctrl Pts',(-0.200000000000014,-1.6868039610115,
-0.519028807441265));
#52794=CARTESIAN_POINT('Ctrl Pts',(-0.20000000000001,-1.65909894074285,
-0.577585106880837));
#52795=CARTESIAN_POINT('Ctrl Pts',(-0.200000000000009,-1.65117900452078,
-0.594324389237043));
#52796=CARTESIAN_POINT('Ctrl Pts',(-0.200000000000001,-1.64297360684206,
-0.610920057491285));
#52797=CARTESIAN_POINT('Ctrl Pts',(-0.2,-1.63448095046,-0.62736452868523));
#52798=CARTESIAN_POINT('Ctrl Pts',(-0.199999999999999,-1.60296311633544,
-0.688393032846946));
#52799=CARTESIAN_POINT('Ctrl Pts',(-0.200000000000001,-1.56749183029575,
-0.74734272741049));
#52800=CARTESIAN_POINT('Ctrl Pts',(-0.2,-1.5283794937604,-0.803982051774627));
#52801=CARTESIAN_POINT('Ctrl Pts',(-0.2,-1.49327907548277,-0.854811640396796));
#52802=CARTESIAN_POINT('Ctrl Pts',(-0.199999999999996,-1.45524503473326,
-0.903780293871229));
#52803=CARTESIAN_POINT('Ctrl Pts',(-0.199999999999995,-1.41448352477257,
-0.950684824964385));
#52804=CARTESIAN_POINT('Ctrl Pts',(-0.199999999999995,-1.40761144044724,
-0.958592576498201));
#52805=CARTESIAN_POINT('Ctrl Pts',(-0.199999999999988,-1.40066422860217,
-0.966438706603342));
#52806=CARTESIAN_POINT('Ctrl Pts',(-0.199999999999989,-1.39364858464507,
-0.974216310602531));
#52807=CARTESIAN_POINT('Ctrl Pts',(-0.199999999999992,-1.35023790133332,
-1.0223417722419));
#52808=CARTESIAN_POINT('Ctrl Pts',(-0.199999999999999,-1.30414795222187,
-1.06791839072618));
#52809=CARTESIAN_POINT('Ctrl Pts',(-0.199999999999998,-1.25565993752712,
-1.11077072511639));
#52810=CARTESIAN_POINT('Ctrl Pts',(-0.199999999999997,-1.20735062750674,
-1.15346512537564));
#52811=CARTESIAN_POINT('Ctrl Pts',(-0.199999999999999,-1.15665986722067,
-1.19345575039044));
#52812=CARTESIAN_POINT('Ctrl Pts',(-0.199999999999997,-1.1038422938188,
-1.23052351620657));
#52813=CARTESIAN_POINT('Ctrl Pts',(-0.199999999999995,-1.05209684405534,
-1.26683885767989));
#52814=CARTESIAN_POINT('Ctrl Pts',(-0.199999999999999,-0.998309111883527,
-1.30034906703051));
#52815=CARTESIAN_POINT('Ctrl Pts',(-0.199999999999999,-0.9427105013579,
-1.33079909790533));
#52816=CARTESIAN_POINT('Ctrl Pts',(-0.199999999999999,-0.932046150008153,
-1.33663970839523));
#52817=CARTESIAN_POINT('Ctrl Pts',(-0.199999999999994,-0.921315174052189,
-1.34236757763251));
#52818=CARTESIAN_POINT('Ctrl Pts',(-0.199999999999994,-0.91051921515542,
-1.34798068133527));
#52819=CARTESIAN_POINT('Ctrl Pts',(-0.199999999999994,-0.901279475695472,
-1.35278466551778));
#52820=CARTESIAN_POINT('Ctrl Pts',(-0.199999999999999,-0.891995974411387,
-1.35750253557107));
#52821=CARTESIAN_POINT('Ctrl Pts',(-0.199999999999998,-0.882676839298332,
-1.36212988869321));
#52822=CARTESIAN_POINT('Ctrl Pts',(-0.199999999999997,-0.827091003392099,
-1.3897306572417));
#52823=CARTESIAN_POINT('Ctrl Pts',(-0.199999999999994,-0.770163374407926,
-1.41415423536456));
#52824=CARTESIAN_POINT('Ctrl Pts',(-0.199999999999995,-0.712128380617553,
-1.43521182130048));
#52825=CARTESIAN_POINT('Ctrl Pts',(-0.199999999999996,-0.65513448315741,
-1.45589165281601));
#52826=CARTESIAN_POINT('Ctrl Pts',(-0.199999999999996,-0.59707173077213,
-1.47332538287411));
#52827=CARTESIAN_POINT('Ctrl Pts',(-0.199999999999998,-0.538158279106556,
-1.48728460270676));
#52828=CARTESIAN_POINT('Ctrl Pts',(-0.200000000000001,-0.481127237836991,
-1.5007977957019));
#52829=CARTESIAN_POINT('Ctrl Pts',(-0.200000000000002,-0.42329831589911,
-1.51105499616133));
#52830=CARTESIAN_POINT('Ctrl Pts',(-0.200000000000004,-0.36487685774904,
-1.5178005978696));
#52831=CARTESIAN_POINT('Ctrl Pts',(-0.200000000000005,-0.34982964427313,
-1.51953801614265));
#52832=CARTESIAN_POINT('Ctrl Pts',(-0.199999999999997,-0.33474319067558,
-1.52104222117722));
#52833=CARTESIAN_POINT('Ctrl Pts',(-0.199999999999998,-0.319621170202251,
-1.52230829911636));
#52834=CARTESIAN_POINT('Ctrl Pts',(-29.8760740822721,-0.685825729128414,
1.3961458803669));
#52835=CARTESIAN_POINT('Ctrl Pts',(-29.8390253006463,-1.15011276588657,
1.16807516083303));
#52836=CARTESIAN_POINT('Ctrl Pts',(-29.7649277373946,-1.82525787394022,
0.216325049098126));
#52837=CARTESIAN_POINT('Ctrl Pts',(-29.6537813925172,-1.17030516464274,
-1.4195844951461));
#52838=CARTESIAN_POINT('Ctrl Pts',(-29.5426350476398,0.557509249428845,
-1.75143349164469));
#52839=CARTESIAN_POINT('Ctrl Pts',(-29.4314887027624,1.77417745764817,-0.482217988040945));
#52840=CARTESIAN_POINT('Ctrl Pts',(-29.320342357885,1.36710299288539,1.22961697865478));
#52841=CARTESIAN_POINT('Ctrl Pts',(-29.2091960130075,-0.291685088526501,
1.81519477428025));
#52842=CARTESIAN_POINT('Ctrl Pts',(-29.0980496681302,-1.68334061031966,
0.739397471666864));
#52843=CARTESIAN_POINT('Ctrl Pts',(-28.9869033232526,-1.534059973681,-1.01344370290772));
#52844=CARTESIAN_POINT('Ctrl Pts',(-28.8757569783753,0.0195899148733162,
-1.83844939731259));
#52845=CARTESIAN_POINT('Ctrl Pts',(-28.7646106334978,1.55529006052317,-0.980514255533821));
#52846=CARTESIAN_POINT('Ctrl Pts',(-28.6534642886204,1.6672258610176,0.775046535726967));
#52847=CARTESIAN_POINT('Ctrl Pts',(-28.542317943743,0.252913801877688,1.82108657460817));
#52848=CARTESIAN_POINT('Ctrl Pts',(-28.4311715988656,-1.39292299951968,
1.20004005839424));
#52849=CARTESIAN_POINT('Ctrl Pts',(-28.3200252539881,-1.76362521504133,
-0.519573359220225));
#52850=CARTESIAN_POINT('Ctrl Pts',(-28.2088789091108,-0.519835724455463,
-1.76354724094302));
#52851=CARTESIAN_POINT('Ctrl Pts',(-28.0977325642333,1.19983124114152,-1.39310245061395));
#52852=CARTESIAN_POINT('Ctrl Pts',(-27.9865862193559,1.82112625016851,0.252642976453954));
#52853=CARTESIAN_POINT('Ctrl Pts',(-27.8754398744784,0.775291433296788,
1.66710893100567));
#52854=CARTESIAN_POINT('Ctrl Pts',(-27.764293529601,-0.980275235800491,
1.55543873831543));
#52855=CARTESIAN_POINT('Ctrl Pts',(-27.6531471847236,-1.83845989126956,
0.019859410984222));
#52856=CARTESIAN_POINT('Ctrl Pts',(-27.5420008398462,-1.01364691392612,
-1.53389995281355));
#52857=CARTESIAN_POINT('Ctrl Pts',(-27.4308544949688,0.739097826986148,
-1.68346772023046));
#52858=CARTESIAN_POINT('Ctrl Pts',(-27.3197081500913,1.81524370282257,-0.291923713345362));
#52859=CARTESIAN_POINT('Ctrl Pts',(-27.2085618052139,1.22964495869491,1.36685859779542));
#52860=CARTESIAN_POINT('Ctrl Pts',(-27.0974154603365,-0.48161855815431,
1.77436544145867));
#52861=CARTESIAN_POINT('Ctrl Pts',(-26.9862691154591,-1.75198973384851,
0.557549214370556));
#52862=CARTESIAN_POINT('Ctrl Pts',(-26.8751227705816,-1.4185214322724,-1.16966922661718));
#52863=CARTESIAN_POINT('Ctrl Pts',(-26.7639764257042,0.213516505753145,
-1.82612700980389));
#52864=CARTESIAN_POINT('Ctrl Pts',(-26.6528300808268,1.65009313818133,-0.810877172722089));
#52865=CARTESIAN_POINT('Ctrl Pts',(-26.5416837359494,1.5761103965168,0.946681135265884));
#52866=CARTESIAN_POINT('Ctrl Pts',(-26.4305373910719,0.0592949571880597,
1.83761074823246));
#52867=CARTESIAN_POINT('Ctrl Pts',(-26.3193910461945,-1.51180138990354,
1.04632008076494));
#52868=CARTESIAN_POINT('Ctrl Pts',(-26.2082447013171,-1.69893600272116,
-0.702812644011505));
#52869=CARTESIAN_POINT('Ctrl Pts',(-26.0970983564397,-0.330798585473345,
-1.80856336626222));
#52870=CARTESIAN_POINT('Ctrl Pts',(-25.9859520115622,1.340164710296,-1.25868491021684));
#52871=CARTESIAN_POINT('Ctrl Pts',(-25.8748056666848,1.78428915735557,0.443442619595842));
#52872=CARTESIAN_POINT('Ctrl Pts',(-25.7636593218074,0.595005980146546,
1.7396255452028));
#52873=CARTESIAN_POINT('Ctrl Pts',(-25.65251297693,-1.13896879060324,1.44328765253607));
#52874=CARTESIAN_POINT('Ctrl Pts',(-25.5413666320525,-1.83028727511895,
-0.174291837069515));
#52875=CARTESIAN_POINT('Ctrl Pts',(-25.4302202871752,-0.846089671080599,
-1.63231780680796));
#52876=CARTESIAN_POINT('Ctrl Pts',(-25.3190739422977,0.912651293186798,
-1.59605663150652));
#52877=CARTESIAN_POINT('Ctrl Pts',(-25.2079275974203,1.83591580205738,-0.0987031999860136));
#52878=CARTESIAN_POINT('Ctrl Pts',(-25.0967812525428,1.07851165011462,1.48900697597377));
#52879=CARTESIAN_POINT('Ctrl Pts',(-24.9856349076655,-0.666203972560349,
1.7136223098677));
#52880=CARTESIAN_POINT('Ctrl Pts',(-24.874488562788,-1.80105059299849,0.369521197485718));
#52881=CARTESIAN_POINT('Ctrl Pts',(-24.7633422179106,-1.2871455197044,-1.31285397704253));
#52882=CARTESIAN_POINT('Ctrl Pts',(-24.6521958730331,0.405062575138557,
-1.79339160925706));
#52883=CARTESIAN_POINT('Ctrl Pts',(-24.5410495281557,1.72646064975028,-0.632188879050662));
#52884=CARTESIAN_POINT('Ctrl Pts',(-24.4299031832783,1.46738956291618,1.10774411511692));
#52885=CARTESIAN_POINT('Ctrl Pts',(-24.3187568384009,-0.134986946113292,
1.83360510424424));
#52886=CARTESIAN_POINT('Ctrl Pts',(-24.2076104935235,-1.61379115967188,
0.88091273511989));
#52887=CARTESIAN_POINT('Ctrl Pts',(-24.0964641486461,-1.61526824084304,
-0.878201380126073));
#52888=CARTESIAN_POINT('Ctrl Pts',(-23.9853178037686,-0.138066012129827,
-1.83337582896308));
#52889=CARTESIAN_POINT('Ctrl Pts',(-23.8741714588912,1.46552720872477,-1.11020680704943));
#52890=CARTESIAN_POINT('Ctrl Pts',(-23.7630251140138,1.7275198787737,0.629288663788884));
#52891=CARTESIAN_POINT('Ctrl Pts',(-23.6518787691364,0.408073727971786,
1.79270884040625));
#52892=CARTESIAN_POINT('Ctrl Pts',(-23.5407324242589,-1.28493896936505,
1.31501368773811));
#52893=CARTESIAN_POINT('Ctrl Pts',(-23.4295860793815,-1.8016686070705,-0.366496090331334));
#52894=CARTESIAN_POINT('Ctrl Pts',(-23.3184397345041,-0.669080796948889,
-1.71250110688599));
#52895=CARTESIAN_POINT('Ctrl Pts',(-23.2072933896267,1.07600957223555,-1.49081606993921));
#52896=CARTESIAN_POINT('Ctrl Pts',(-23.0961470447492,1.83607896999803,0.0956199239828239));
#52897=CARTESIAN_POINT('Ctrl Pts',(-22.9850006998718,0.91533033667428,1.59452172412145));
#52898=CARTESIAN_POINT('Ctrl Pts',(-22.8738543549944,-0.843347252550528,
1.633736381901));
#52899=CARTESIAN_POINT('Ctrl Pts',(-22.7627080101169,-1.82999199802708,
0.177365275881016));
#52900=CARTESIAN_POINT('Ctrl Pts',(-22.6515616652396,-1.14139096307257,
-1.44137289531467));
#52901=CARTESIAN_POINT('Ctrl Pts',(-22.5404153203621,0.592083708909288,
-1.74062231273063));
#52902=CARTESIAN_POINT('Ctrl Pts',(-22.4292689754847,1.78354194798782,-0.446438432148635));
#52903=CARTESIAN_POINT('Ctrl Pts',(-22.3181226306072,1.34227658728578,1.25643253585536));
#52904=CARTESIAN_POINT('Ctrl Pts',(-22.2069762857299,-0.327760916379816,
1.80911634109733));
#52905=CARTESIAN_POINT('Ctrl Pts',(-22.0958299408524,-1.69775334184427,
0.705664753397891));
#52906=CARTESIAN_POINT('Ctrl Pts',(-21.984683595975,-1.51355639095973,-1.04377976858935));
#52907=CARTESIAN_POINT('Ctrl Pts',(-21.8735372510976,0.056208890351046,
-1.83770773372074));
#52908=CARTESIAN_POINT('Ctrl Pts',(-21.7623909062202,1.57451836940432,-0.949326634167536));
#52909=CARTESIAN_POINT('Ctrl Pts',(-21.6512445613427,1.65145255424892,0.808104952958591));
#52910=CARTESIAN_POINT('Ctrl Pts',(-21.5400982164653,0.216582902754202,
1.82576586674362));
#52911=CARTESIAN_POINT('Ctrl Pts',(-21.4289518715879,-1.41655515338036,
1.17204976488333));
#52912=CARTESIAN_POINT('Ctrl Pts',(-21.3178055267105,-1.75292358101011,
-0.554606232448005));
#52913=CARTESIAN_POINT('Ctrl Pts',(-21.206659181833,-0.484597651685728,
-1.77355413503851));
#52914=CARTESIAN_POINT('Ctrl Pts',(-21.0955128369556,1.2273477973243,-1.36892166990471));
#52915=CARTESIAN_POINT('Ctrl Pts',(-20.9843664920782,1.81573138332858,0.288874882132692));
#52916=CARTESIAN_POINT('Ctrl Pts',(-20.8732201472008,0.741923909701551,
1.68222414265896));
#52917=CARTESIAN_POINT('Ctrl Pts',(-20.7620738023233,-1.01106953876495,
1.53560005916682));
#52918=CARTESIAN_POINT('Ctrl Pts',(-20.6509274574459,-1.83849064573244,
-0.0167719851482926));
#52919=CARTESIAN_POINT('Ctrl Pts',(-20.5397811125685,-0.982885979939318,
-1.55379030257311));
#52920=CARTESIAN_POINT('Ctrl Pts',(-20.4286347676911,0.772490702514734,
-1.66840860356802));
#52921=CARTESIAN_POINT('Ctrl Pts',(-20.3174884228136,1.82069938029707,-0.255700841839434));
#52922=CARTESIAN_POINT('Ctrl Pts',(-20.2063420779362,1.20216910098862,1.3910854059186));
#52923=CARTESIAN_POINT('Ctrl Pts',(-20.0951957330588,-0.516873484366524,
1.76441802164065));
#52924=CARTESIAN_POINT('Ctrl Pts',(-19.9840493881814,-1.7627499987032,0.52253382283197));
#52925=CARTESIAN_POINT('Ctrl Pts',(-19.872903043304,-1.39493667151811,-1.1976981407623));
#52926=CARTESIAN_POINT('Ctrl Pts',(-19.7617566984265,0.249855885875982,
-1.82151068902289));
#52927=CARTESIAN_POINT('Ctrl Pts',(-19.6506103535491,1.66592065703884,-0.777841576661194));
#52928=CARTESIAN_POINT('Ctrl Pts',(-19.5394640086717,1.55693692840167,0.977893938477322));
#52929=CARTESIAN_POINT('Ctrl Pts',(-19.4283176637942,0.0226726397870904,
1.83842734567798));
#52930=CARTESIAN_POINT('Ctrl Pts',(-19.3171713189168,-1.53234706424761,
1.01599292744745));
#52931=CARTESIAN_POINT('Ctrl Pts',(-19.2060249740394,-1.68459672540546,
-0.736520893583273));
#52932=CARTESIAN_POINT('Ctrl Pts',(-19.094878629162,-0.29470108811063,-1.81479487066663));
#52933=CARTESIAN_POINT('Ctrl Pts',(-18.9837322842846,1.36497537602827,-1.23173510819818));
#52934=CARTESIAN_POINT('Ctrl Pts',(-18.8725859394071,1.77510034401367,0.478902832121552));
#52935=CARTESIAN_POINT('Ctrl Pts',(-18.7614395945297,0.560229484500028,
1.75113451186034));
#52936=CARTESIAN_POINT('Ctrl Pts',(-18.6502932496523,-1.1674972131777,1.42030961806002));
#52937=CARTESIAN_POINT('Ctrl Pts',(-18.5391469047748,-1.82645159810784,
-0.210721887094827));
#52938=CARTESIAN_POINT('Ctrl Pts',(-18.4280005598975,-0.813401222257357,
-1.64885038907772));
#52939=CARTESIAN_POINT('Ctrl Pts',(-18.31685421502,0.94426823764005,-1.57755717782769));
#52940=CARTESIAN_POINT('Ctrl Pts',(-18.2057078701426,1.83751786269281,-0.0621068290635167));
#52941=CARTESIAN_POINT('Ctrl Pts',(-18.0945615252652,1.04863223837752,1.51019852422351));
#52942=CARTESIAN_POINT('Ctrl Pts',(-17.9834151803877,-0.700212082183364,
1.70000946876656));
#52943=CARTESIAN_POINT('Ctrl Pts',(-17.8722688355103,-1.80805505555301,
0.333565690712785));
#52944=CARTESIAN_POINT('Ctrl Pts',(-17.7611224906329,-1.26073417800543,
-1.33823708151452));
#52945=CARTESIAN_POINT('Ctrl Pts',(-17.6499761457555,0.440711752671261,
-1.78496563131869));
#52946=CARTESIAN_POINT('Ctrl Pts',(-17.5388298008781,1.73871302083308,-0.59766728630315));
#52947=CARTESIAN_POINT('Ctrl Pts',(-17.4276834560006,1.44502883098667,1.1367589153153));
#52948=CARTESIAN_POINT('Ctrl Pts',(-17.3165371111232,-0.171490898207203,
1.83055183640442));
#52949=CARTESIAN_POINT('Ctrl Pts',(-17.2053907662458,-1.63102119580044,
0.848586479258995));
#52950=CARTESIAN_POINT('Ctrl Pts',(-17.0942444213684,-1.5974513164508,-0.91020791333691));
#52951=CARTESIAN_POINT('Ctrl Pts',(-16.9830980764909,-0.101512432092709,
-1.83576261538962));
#52952=CARTESIAN_POINT('Ctrl Pts',(-16.8719517316135,1.48735487692949,-1.08078888965679));
#52953=CARTESIAN_POINT('Ctrl Pts',(-16.7608053867361,1.71463973954429,0.663580980368641));
#52954=CARTESIAN_POINT('Ctrl Pts',(-16.6496590418587,0.372276761224383,
1.80048303712748));
#52955=CARTESIAN_POINT('Ctrl Pts',(-16.5385126969812,-1.31088282935724,
1.28915296285113));
#52956=CARTESIAN_POINT('Ctrl Pts',(-16.4273663521038,-1.79400934280639,
-0.402317824431001));
#52957=CARTESIAN_POINT('Ctrl Pts',(-16.3162200072264,-0.634829996541143,
-1.72549124292854));
#52958=CARTESIAN_POINT('Ctrl Pts',(-16.205073662349,1.10549739525827,-1.46908293265175));
#52959=CARTESIAN_POINT('Ctrl Pts',(-16.0939273174715,1.83380951667369,0.132180976273241));
#52960=CARTESIAN_POINT('Ctrl Pts',(-15.9827809725941,0.883381152756941,
1.61244128354657));
#52961=CARTESIAN_POINT('Ctrl Pts',(-15.8716346277167,-0.875728642698206,
1.61661018748783));
#52962=CARTESIAN_POINT('Ctrl Pts',(-15.7604882828393,-1.83316241166559,
0.140871311443935));
#52963=CARTESIAN_POINT('Ctrl Pts',(-15.6493419379619,-1.11244808036887,
-1.46382663673507));
#52964=CARTESIAN_POINT('Ctrl Pts',(-15.5381955930844,0.626644448535124,
-1.72848080378452));
#52965=CARTESIAN_POINT('Ctrl Pts',(-15.427049248207,1.79208230060405,-0.410816481890913));
#52966=CARTESIAN_POINT('Ctrl Pts',(-15.3159029033296,1.31697838226697,1.28292521004654));
#52967=CARTESIAN_POINT('Ctrl Pts',(-15.2047565584522,-0.363738719182501,
1.80222731587859));
#52968=CARTESIAN_POINT('Ctrl Pts',(-15.0936102135747,-1.71147526380616,
0.671700510131698));
#52969=CARTESIAN_POINT('Ctrl Pts',(-14.9824638686973,-1.49246085154338,
-1.0737270419161));
#52970=CARTESIAN_POINT('Ctrl Pts',(-14.8713175238199,0.0928102146840508,
-1.83622313948545));
#52971=CARTESIAN_POINT('Ctrl Pts',(-14.7601711789425,1.59311920419314,-0.917769227618005));
#52972=CARTESIAN_POINT('Ctrl Pts',(-14.649024834065,1.63502497258126,0.840846295684967));
#52973=CARTESIAN_POINT('Ctrl Pts',(-14.5378784891876,0.180165351192192,
1.82971844833059));
#52974=CARTESIAN_POINT('Ctrl Pts',(-14.4267321443102,-1.43962463311105,
1.14359523856626));
#52975=CARTESIAN_POINT('Ctrl Pts',(-14.3155857994328,-1.74152629078552,
-0.589419487660784));
#52976=CARTESIAN_POINT('Ctrl Pts',(-14.2044394545554,-0.449167113826005,
-1.78285671263529));
#52977=CARTESIAN_POINT('Ctrl Pts',(-14.0932931096779,1.25437709178756,-1.34419762889618));
#52978=CARTESIAN_POINT('Ctrl Pts',(-13.9821467648005,1.80961576800425,0.324992193939892));
#52979=CARTESIAN_POINT('Ctrl Pts',(-13.8710004199231,0.708261856483432,
1.69667153467668));
#52980=CARTESIAN_POINT('Ctrl Pts',(-13.7598540750457,-1.04146247840172,
1.51515182737997));
#52981=CARTESIAN_POINT('Ctrl Pts',(-13.6487077301683,-1.83779159390846,
-0.0533967348337232));
#52982=CARTESIAN_POINT('Ctrl Pts',(-13.5375613852908,-0.951734875856344,
-1.57306385121844));
#52983=CARTESIAN_POINT('Ctrl Pts',(-13.4264150404134,0.805576927784317,
-1.65268719585804));
#52984=CARTESIAN_POINT('Ctrl Pts',(-13.315268695536,1.82543231055633,-0.219376465256566));
#52985=CARTESIAN_POINT('Ctrl Pts',(-13.2041223506585,1.1742160279774,1.41476000564494));
#52986=CARTESIAN_POINT('Ctrl Pts',(-13.0929760057811,-0.55192323148034,
1.75377019603021));
#52987=CARTESIAN_POINT('Ctrl Pts',(-12.9818296609037,-1.77281051953266,
0.487311005176181));
#52988=CARTESIAN_POINT('Ctrl Pts',(-12.8706833160263,-1.37079817438837,
-1.22525161457759));
#52989=CARTESIAN_POINT('Ctrl Pts',(-12.7595369711488,0.286096082776584,
-1.81617129846043));
#52990=CARTESIAN_POINT('Ctrl Pts',(-12.6483906262714,1.6810868693329,-0.74449720730706));
#52991=CARTESIAN_POINT('Ctrl Pts',(-12.537244281394,1.53714541606292,1.00871855530086));
#52992=CARTESIAN_POINT('Ctrl Pts',(-12.4260979365166,-0.0139586777784811,
1.83851415802169));
#52993=CARTESIAN_POINT('Ctrl Pts',(-12.3149515916392,-1.55228445560866,
0.985262463918737));
#52994=CARTESIAN_POINT('Ctrl Pts',(-12.2038052467617,-1.66958872783078,
-0.769936772619606));
#52995=CARTESIAN_POINT('Ctrl Pts',(-12.0926589018843,-0.258486605724834,
-1.82030597114671));
#52996=CARTESIAN_POINT('Ctrl Pts',(-11.9815125570069,1.38924419891378,-1.20429635460542));
#52997=CARTESIAN_POINT('Ctrl Pts',(-11.8703662121295,1.76520688394983,0.514172938599101));
#52998=CARTESIAN_POINT('Ctrl Pts',(-11.759219867252,0.525230599245605,1.76194834531198));
#52999=CARTESIAN_POINT('Ctrl Pts',(-11.6480735223746,-1.19556218415814,
1.39676777516613));
#53000=CARTESIAN_POINT('Ctrl Pts',(-11.5369271774972,-1.82189088989749,
-0.247068288616763));
#53001=CARTESIAN_POINT('Ctrl Pts',(-11.4257808326198,-0.780389884361033,
-1.66472844101327));
#53002=CARTESIAN_POINT('Ctrl Pts',(-11.3146344877423,0.975510343836714,
-1.55843149448383));
#53003=CARTESIAN_POINT('Ctrl Pts',(-11.2034881428649,1.83839049924661,-0.0254858041131052));
#53004=CARTESIAN_POINT('Ctrl Pts',(-11.0923417979875,1.01833655988029,1.53079058160895));
#53005=CARTESIAN_POINT('Ctrl Pts',(-10.9811954531101,-0.733942234478493,
1.68572178913967));
#53006=CARTESIAN_POINT('Ctrl Pts',(-10.8700491082326,-1.81434178962977,
0.297477771160369));
#53007=CARTESIAN_POINT('Ctrl Pts',(-10.7589027633552,-1.23382237321512,
-1.3630889572164));
#53008=CARTESIAN_POINT('Ctrl Pts',(-10.6477564184778,0.476185984549256,
-1.77583109051801));
#53009=CARTESIAN_POINT('Ctrl Pts',(-10.5366100736004,1.7502751895651,-0.562908442576898));
#53010=CARTESIAN_POINT('Ctrl Pts',(-10.4254637287229,1.4220944780604,1.16532246584438));
#53011=CARTESIAN_POINT('Ctrl Pts',(-10.3143173838456,-0.207926774994991,
1.82677190972811));
#53012=CARTESIAN_POINT('Ctrl Pts',(-10.2031710389681,-1.64760377910037,
0.815923367128113));
#53013=CARTESIAN_POINT('Ctrl Pts',(-10.0920246940907,-1.57900026518387,
-0.941853128932933));
#53014=CARTESIAN_POINT('Ctrl Pts',(-9.98087834921326,-0.0649185555153559,
-1.83742067450035));
#53015=CARTESIAN_POINT('Ctrl Pts',(-9.86973200433583,1.50859212232134,-1.05094194054737));
#53016=CARTESIAN_POINT('Ctrl Pts',(-9.75858565945843,1.70107895413302,0.697609880762318));
#53017=CARTESIAN_POINT('Ctrl Pts',(-9.64743931458098,0.33633201488792,1.80754251117172));
#53018=CARTESIAN_POINT('Ctrl Pts',(-9.53629296970358,-1.33630631916782,
1.26278049370572));
#53019=CARTESIAN_POINT('Ctrl Pts',(-9.42514662482614,-1.78563792567352,
-0.437979853792231));
#53020=CARTESIAN_POINT('Ctrl Pts',(-9.31400027994872,-0.600327192984703,
-1.73779642515878));
#53021=CARTESIAN_POINT('Ctrl Pts',(-9.20285393507129,1.13454637823559,-1.44676662581219));
#53022=CARTESIAN_POINT('Ctrl Pts',(-9.09170759019388,1.83081211133877,0.168689557788168));
#53023=CARTESIAN_POINT('Ctrl Pts',(-8.98056124531644,0.851081300419372,
1.62972076565527));
#53024=CARTESIAN_POINT('Ctrl Pts',(-8.86941490043904,-0.907762402178502,
1.59884226086334));
#53025=CARTESIAN_POINT('Ctrl Pts',(-8.7582685555616,-1.83560513016937,0.104321426501776));
#53026=CARTESIAN_POINT('Ctrl Pts',(-8.64712221068418,-1.08306359846452,
-1.48569929515115));
#53027=CARTESIAN_POINT('Ctrl Pts',(-8.53597586580675,0.660956434360724,
-1.71565315428517));
#53028=CARTESIAN_POINT('Ctrl Pts',(-8.42482952092933,1.79991126531332,-0.375031453253858));
#53029=CARTESIAN_POINT('Ctrl Pts',(-8.31368317605192,1.29115738736595,1.30890861215818));
#53030=CARTESIAN_POINT('Ctrl Pts',(-8.20253683117448,-0.399572131671196,
1.79462287557114));
#53031=CARTESIAN_POINT('Ctrl Pts',(-8.09139048629707,-1.7245177957616,0.637469627537685));
#53032=CARTESIAN_POINT('Ctrl Pts',(-7.98024414141963,-1.47077286243819,
-1.10324808680863));
#53033=CARTESIAN_POINT('Ctrl Pts',(-7.86909779654222,0.12937469692319,-1.83400963512396));
#53034=CARTESIAN_POINT('Ctrl Pts',(-7.75795145166479,1.61108763178959,-0.885847501902045));
#53035=CARTESIAN_POINT('Ctrl Pts',(-7.64680510678736,1.61794834873923,0.873253854697203));
#53036=CARTESIAN_POINT('Ctrl Pts',(-7.53565876190995,0.143676280899092,
1.83294470190416));
#53037=CARTESIAN_POINT('Ctrl Pts',(-7.42451241703252,-1.46212263710416,
1.11468674882187));
#53038=CARTESIAN_POINT('Ctrl Pts',(-7.3133660721551,-1.72943768144993,-0.623998765954385));
#53039=CARTESIAN_POINT('Ctrl Pts',(-7.20221972727767,-0.413558273857659,
-1.79145156452956));
#53040=CARTESIAN_POINT('Ctrl Pts',(-7.09107338240025,1.28090844667878,-1.31893999300895));
#53041=CARTESIAN_POINT('Ctrl Pts',(-6.97992703752282,1.80278180465922,0.360980496316825));
#53042=CARTESIAN_POINT('Ctrl Pts',(-6.8687806926454,0.674318650485929,1.71044541320042));
#53043=CARTESIAN_POINT('Ctrl Pts',(-6.75763434776798,-1.07144199739794,
1.49410213845754));
#53044=CARTESIAN_POINT('Ctrl Pts',(-6.64648800289056,-1.83636300934206,
-0.0900002880644057));
#53045=CARTESIAN_POINT('Ctrl Pts',(-6.53534165801313,-0.920205969547918,
-1.59171295387702));
#53046=CARTESIAN_POINT('Ctrl Pts',(-6.42419531313571,0.838343369925463,
-1.63630973474875));
#53047=CARTESIAN_POINT('Ctrl Pts',(-6.31304896825829,1.82944061423442,-0.182965004634956));
#53048=CARTESIAN_POINT('Ctrl Pts',(-6.20190262338086,1.14579683626047,1.43787299993672));
#53049=CARTESIAN_POINT('Ctrl Pts',(-6.09075627850344,-0.586753886249875,
1.74242619094817));
#53050=CARTESIAN_POINT('Ctrl Pts',(-5.97960993362602,-1.78216730261277,
0.451894743750581));
#53051=CARTESIAN_POINT('Ctrl Pts',(-5.86846358874859,-1.34611552298411,
-1.25231871051771));
#53052=CARTESIAN_POINT('Ctrl Pts',(-5.75731724387117,0.322222710510533,
-1.81011095758319));
#53053=CARTESIAN_POINT('Ctrl Pts',(-5.64617089899375,1.69558575464707,-0.710857301129708));
#53054=CARTESIAN_POINT('Ctrl Pts',(-5.53502455411632,1.51674371597785,1.03914274956487));
#53055=CARTESIAN_POINT('Ctrl Pts',(-5.4238782092389,-0.0505844542846405,
1.83787115079273));
#53056=CARTESIAN_POINT('Ctrl Pts',(-5.31273186436147,-1.57160564960563,
0.954140888998658));
#53057=CARTESIAN_POINT('Ctrl Pts',(-5.20158551948405,-1.65391796759717,
-0.803047016301529));
#53058=CARTESIAN_POINT('Ctrl Pts',(-5.09043917460663,-0.22216951407526,
-1.82509448000564));
#53059=CARTESIAN_POINT('Ctrl Pts',(-4.9792928297292,1.4129615451609,-1.17637954157153));
#53060=CARTESIAN_POINT('Ctrl Pts',(-4.86814648485178,1.75461270448817,0.549238938150095));
#53061=CARTESIAN_POINT('Ctrl Pts',(-4.75700013997435,0.490023217597568,
1.7720627528806));
#53062=CARTESIAN_POINT('Ctrl Pts',(-4.64585379509693,-1.22315256282799,
1.37267146906276));
#53063=CARTESIAN_POINT('Ctrl Pts',(-4.53470745021951,-1.81660696091404,
-0.28331661350876));
#53064=CARTESIAN_POINT('Ctrl Pts',(-4.42356110534208,-0.747068761626052,
-1.67994565963717));
#53065=CARTESIAN_POINT('Ctrl Pts',(-4.31241476046467,1.00636520985961,-1.53868717363749));
#53066=CARTESIAN_POINT('Ctrl Pts',(-4.20126841558724,1.83853336531533,0.0111453377239352));
#53067=CARTESIAN_POINT('Ctrl Pts',(-4.09012207070981,0.987636640845155,
1.55077497387288));
#53068=CARTESIAN_POINT('Ctrl Pts',(-3.9789757258324,-0.767381039870437,
1.6707649426488));
#53069=CARTESIAN_POINT('Ctrl Pts',(-3.86782938095496,-1.81990829963504,
0.26127176434536));
#53070=CARTESIAN_POINT('Ctrl Pts',(-3.75668303607755,-1.20642078829025,
-1.38739973890271));
#53071=CARTESIAN_POINT('Ctrl Pts',(-3.64553669120012,0.511471188869394,
-1.7659916129257));
#53072=CARTESIAN_POINT('Ctrl Pts',(-3.5343903463227,1.76114256619831,-0.527926145782834));
#53073=CARTESIAN_POINT('Ctrl Pts',(-3.42324400144528,1.3985956082158,1.19342342803983));
#53074=CARTESIAN_POINT('Ctrl Pts',(-3.31209765656785,-0.244280112870538,
1.82226682475983));
#53075=CARTESIAN_POINT('Ctrl Pts',(-3.20095131169043,-1.66353232684867,
0.782936364617715));
#53076=CARTESIAN_POINT('Ctrl Pts',(-3.089804966813,-1.55992241154186,-0.973124464765563));
#53077=CARTESIAN_POINT('Ctrl Pts',(-2.97865862193558,-0.0282989084957232,
-1.83834934851334));
#53078=CARTESIAN_POINT('Ctrl Pts',(-2.86751227705816,1.52923051402139,-1.02067780704635));
#53079=CARTESIAN_POINT('Ctrl Pts',(-2.75636593218073,1.6868429066166,0.731361855340862));
#53080=CARTESIAN_POINT('Ctrl Pts',(-2.64521958730331,0.300253755811285,
1.81388446297849));
#53081=CARTESIAN_POINT('Ctrl Pts',(-2.53407324242589,-1.36119934315438,
1.23590674387245));
#53082=CARTESIAN_POINT('Ctrl Pts',(-2.42292689754847,-1.77655768544653,
-0.473468011899886));
#53083=CARTESIAN_POINT('Ctrl Pts',(-2.31178055267104,-0.565586069932105,
-1.74941178802327));
#53084=CARTESIAN_POINT('Ctrl Pts',(-2.20063420779361,1.16314496579956,-1.42387597174662));
#53085=CARTESIAN_POINT('Ctrl Pts',(-2.08948786291619,1.82708798956902,0.205131106799974));
#53086=CARTESIAN_POINT('Ctrl Pts',(-1.97834151803877,0.818443514495715,
1.64635344282621));
#53087=CARTESIAN_POINT('Ctrl Pts',(-1.86719517316135,-0.939435649392642,
1.58043940475681));
#53088=CARTESIAN_POINT('Ctrl Pts',(-1.75604882828392,-1.83731949853668,
0.067730606360174));
#53089=CARTESIAN_POINT('Ctrl Pts',(-1.6449024834065,-1.05324858333434,-1.50698309414738));
#53090=CARTESIAN_POINT('Ctrl Pts',(-1.53375613852907,0.695004907338835,
-1.70214273260888));
#53091=CARTESIAN_POINT('Ctrl Pts',(-1.42260979365165,1.80702789992282,-0.339100830268501));
#53092=CARTESIAN_POINT('Ctrl Pts',(-1.31146344877422,1.26481973322455,1.33437866444013));
#53093=CARTESIAN_POINT('Ctrl Pts',(-1.2003171038968,-0.43523909383229,1.78629417578513));
#53094=CARTESIAN_POINT('Ctrl Pts',(-1.08917075901938,-1.73689066467127,
0.603008259306024));
#53095=CARTESIAN_POINT('Ctrl Pts',(-0.978024414141956,-1.44847268249357,
-1.13237410758484));
#53096=CARTESIAN_POINT('Ctrl Pts',(-0.866878069264529,0.165833894051307,
-1.83098644971143));
#53097=CARTESIAN_POINT('Ctrl Pts',(-0.755731724387107,1.62851911260145,
-0.853729469588644));
#53098=CARTESIAN_POINT('Ctrl Pts',(-0.644585379509683,1.60003419765428,
0.9056105153729));
#53099=CARTESIAN_POINT('Ctrl Pts',(-0.533439034632261,0.107502597833407,
1.83487847835014));
#53100=CARTESIAN_POINT('Ctrl Pts',(-0.422292689754837,-1.48475723354389,
1.08643005973131));
#53101=CARTESIAN_POINT('Ctrl Pts',(-0.311146344877411,-1.71522461751901,
-0.660581065959966));
#53102=CARTESIAN_POINT('Ctrl Pts',(-0.237048781625798,-0.82586340403187,
-1.41601857102626));
#53103=CARTESIAN_POINT('Ctrl Pts',(-0.199999999999991,-0.319621170202164,
-1.52230829911638));
#53104=CARTESIAN_POINT('Ctrl Pts',(-29.7993827215147,-0.74439243930905,
1.51537102412048));
#53105=CARTESIAN_POINT('Ctrl Pts',(-29.7623339398889,-1.24832768867796,
1.26782399863261));
#53106=CARTESIAN_POINT('Ctrl Pts',(-29.6882363766373,-1.98112742558818,
0.234798322871887));
#53107=CARTESIAN_POINT('Ctrl Pts',(-29.5770900317599,-1.27024443564024,
-1.54081120066757));
#53108=CARTESIAN_POINT('Ctrl Pts',(-29.4659436868824,0.605118257442928,
-1.90099874320803));
#53109=CARTESIAN_POINT('Ctrl Pts',(-29.354797342005,1.92568495081712,-0.523397430499743));
#53110=CARTESIAN_POINT('Ctrl Pts',(-29.2436509971276,1.48384799292067,1.33462123580558));
#53111=CARTESIAN_POINT('Ctrl Pts',(-29.1325046522502,-0.316593801218701,
1.97020497840553));
#53112=CARTESIAN_POINT('Ctrl Pts',(-29.0213583073727,-1.82709100852228,
0.802538989390837));
#53113=CARTESIAN_POINT('Ctrl Pts',(-28.9102119624953,-1.66506241652075,
-1.09998764710766));
#53114=CARTESIAN_POINT('Ctrl Pts',(-28.7990656176179,0.0212628134219854,
-1.9954454510636));
#53115=CARTESIAN_POINT('Ctrl Pts',(-28.6879192727405,1.68810546588451,-1.06424615970824));
#53116=CARTESIAN_POINT('Ctrl Pts',(-28.5767729278631,1.80960012558748,0.84123233761007));
#53117=CARTESIAN_POINT('Ctrl Pts',(-28.4656265829856,0.274511605380939,
1.97659991436632));
#53118=CARTESIAN_POINT('Ctrl Pts',(-28.3544802381082,-1.51187292244025,
1.30251856761311));
#53119=CARTESIAN_POINT('Ctrl Pts',(-28.2433338932308,-1.91423158988198,
-0.563942797482219));
#53120=CARTESIAN_POINT('Ctrl Pts',(-28.1321875483534,-0.564227567634542,
-1.91414695711486));
#53121=CARTESIAN_POINT('Ctrl Pts',(-28.0210412034759,1.3022919182218,-1.51206769792338));
#53122=CARTESIAN_POINT('Ctrl Pts',(-27.9098948585985,1.9766429780571,0.274217652574654));
#53123=CARTESIAN_POINT('Ctrl Pts',(-27.798748513721,0.841498148429855,1.8094732102312));
#53124=CARTESIAN_POINT('Ctrl Pts',(-27.6876021688437,-1.06398672866812,
1.68826684015161));
#53125=CARTESIAN_POINT('Ctrl Pts',(-27.5764558239662,-1.99545684116154,
0.0215553233975659));
#53126=CARTESIAN_POINT('Ctrl Pts',(-27.4653094790888,-1.10020821151516,
-1.66488873052626));
#53127=CARTESIAN_POINT('Ctrl Pts',(-27.3541631342114,0.802213756280972,
-1.82722897309913));
#53128=CARTESIAN_POINT('Ctrl Pts',(-27.243016789334,1.97025808524513,-0.316852803620255));
#53129=CARTESIAN_POINT('Ctrl Pts',(-27.1318704444566,1.3346516052265,1.48358272749042));
#53130=CARTESIAN_POINT('Ctrl Pts',(-27.0207240995791,-0.522746811754401,
1.92588898767558));
#53131=CARTESIAN_POINT('Ctrl Pts',(-26.9095777547017,-1.90160248621939,
0.605161635226943));
#53132=CARTESIAN_POINT('Ctrl Pts',(-26.7984314098243,-1.53965735657548,
-1.26955419111032));
#53133=CARTESIAN_POINT('Ctrl Pts',(-26.6872850649469,0.231749941420772,
-1.98207078209722));
#53134=CARTESIAN_POINT('Ctrl Pts',(-26.5761387200694,1.79100433834535,-0.880122764349528));
#53135=CARTESIAN_POINT('Ctrl Pts',(-26.464992375192,1.7107037733542,1.02752382944862));
#53136=CARTESIAN_POINT('Ctrl Pts',(-26.3538460303146,0.0643585038373884,
1.99453518478462));
#53137=CARTESIAN_POINT('Ctrl Pts',(-26.2426996854372,-1.64090304079323,
1.13567153307063));
#53138=CARTESIAN_POINT('Ctrl Pts',(-26.1315533405598,-1.84401818360282,
-0.76282996719567));
#53139=CARTESIAN_POINT('Ctrl Pts',(-26.0204069956823,-0.359047430712987,
-1.96300727528516));
#53140=CARTESIAN_POINT('Ctrl Pts',(-25.9092606508049,1.45460929125672,-1.36617144974778));
#53141=CARTESIAN_POINT('Ctrl Pts',(-25.7981143059275,1.93666014829227,0.481310804297285));
#53142=CARTESIAN_POINT('Ctrl Pts',(-25.68696796105,0.645817055489537,1.88818244647001));
#53143=CARTESIAN_POINT('Ctrl Pts',(-25.5758216161726,-1.23623206351777,
1.56653851068145));
#53144=CARTESIAN_POINT('Ctrl Pts',(-25.4646752712952,-1.9865863170422,-0.189175646578258));
#53145=CARTESIAN_POINT('Ctrl Pts',(-25.3535289264178,-0.91834226594298,
-1.77171106642719));
#53146=CARTESIAN_POINT('Ctrl Pts',(-25.2423825815403,0.990587978140239,
-1.73235333517204));
#53147=CARTESIAN_POINT('Ctrl Pts',(-25.1312362366629,1.99269549714361,-0.107132049272218));
#53148=CARTESIAN_POINT('Ctrl Pts',(-25.0200898917855,1.17061213068258,1.61616207721148));
#53149=CARTESIAN_POINT('Ctrl Pts',(-24.9089435469081,-0.723095065041999,
1.85995864126857));
#53150=CARTESIAN_POINT('Ctrl Pts',(-24.7977972020306,-1.95485294193452,
0.401076795299436));
#53151=CARTESIAN_POINT('Ctrl Pts',(-24.6866508571532,-1.39706247879622,
-1.42496633316633));
#53152=CARTESIAN_POINT('Ctrl Pts',(-24.5755045122758,0.439653261132996,
-1.94653991232978));
#53153=CARTESIAN_POINT('Ctrl Pts',(-24.4643581673984,1.87389332282981,-0.686175221770339));
#53154=CARTESIAN_POINT('Ctrl Pts',(-24.353211822521,1.59269862555882,1.20234092854762));
#53155=CARTESIAN_POINT('Ctrl Pts',(-24.2420654776435,-0.146514278809422,
1.9901874751949));
#53156=CARTESIAN_POINT('Ctrl Pts',(-24.1309191327661,-1.75160231945531,
0.956139077120314));
#53157=CARTESIAN_POINT('Ctrl Pts',(-24.0197727878887,-1.75320553731272,
-0.95319618350774));
#53158=CARTESIAN_POINT('Ctrl Pts',(-23.9086264430113,-0.149856284460993,
-1.98993862074318));
#53159=CARTESIAN_POINT('Ctrl Pts',(-23.7974800981338,1.59067723394218,-1.20501392429124));
#53160=CARTESIAN_POINT('Ctrl Pts',(-23.6863337532564,1.87504300567635,0.683027339995933));
#53161=CARTESIAN_POINT('Ctrl Pts',(-23.575187408379,0.442921554093378,1.94579883781372));
#53162=CARTESIAN_POINT('Ctrl Pts',(-23.4640410635016,-1.39466749808941,
1.4273104743155));
#53163=CARTESIAN_POINT('Ctrl Pts',(-23.3528947186241,-1.95552373187871,
-0.397793356375988));
#53164=CARTESIAN_POINT('Ctrl Pts',(-23.2417483737467,-0.726217558458331,
-1.85874169214136));
#53165=CARTESIAN_POINT('Ctrl Pts',(-23.1306020288693,1.16789638559377,-1.61812566039685));
#53166=CARTESIAN_POINT('Ctrl Pts',(-23.0194556839919,1.99287259895853,0.103785474118366));
#53167=CARTESIAN_POINT('Ctrl Pts',(-22.9083093391144,0.993495800976093,
1.73068735297875));
#53168=CARTESIAN_POINT('Ctrl Pts',(-22.797162994237,-0.915365656095304,
1.77325078202687));
#53169=CARTESIAN_POINT('Ctrl Pts',(-22.6860166493596,-1.98626582449528,
0.192511544484518));
#53170=CARTESIAN_POINT('Ctrl Pts',(-22.5748703044822,-1.2388610796019,-1.56446024103054));
#53171=CARTESIAN_POINT('Ctrl Pts',(-22.4637239596048,0.642645234249625,
-1.8892643338649));
#53172=CARTESIAN_POINT('Ctrl Pts',(-22.3525776147273,1.93584913030288,-0.484562446980071));
#53173=CARTESIAN_POINT('Ctrl Pts',(-22.2414312698499,1.45690151389741,1.36372673183492));
#53174=CARTESIAN_POINT('Ctrl Pts',(-22.1302849249725,-0.355750357112206,
1.96360747190783));
#53175=CARTESIAN_POINT('Ctrl Pts',(-22.0191385800951,-1.84273452832774,
0.765925635049822));
#53176=CARTESIAN_POINT('Ctrl Pts',(-21.9079922352176,-1.64280791175631,
-1.13291428863289));
#53177=CARTESIAN_POINT('Ctrl Pts',(-21.7968458903402,0.0610088995239246,
-1.99464045243663));
#53178=CARTESIAN_POINT('Ctrl Pts',(-21.6856995454628,1.70897579364258,-1.03039524312831));
#53179=CARTESIAN_POINT('Ctrl Pts',(-21.5745532005853,1.79247984298095,0.877113808365062));
#53180=CARTESIAN_POINT('Ctrl Pts',(-21.463406855708,0.235078196174796,1.98167879889778));
#53181=CARTESIAN_POINT('Ctrl Pts',(-21.3522605108305,-1.53752316551414,
1.27213801760072));
#53182=CARTESIAN_POINT('Ctrl Pts',(-21.2411141659531,-1.90261608010631,
-0.601967334693983));
#53183=CARTESIAN_POINT('Ctrl Pts',(-21.1299678210757,-0.525980307679819,
-1.92500839900785));
#53184=CARTESIAN_POINT('Ctrl Pts',(-21.0188214761983,1.33215827567724,-1.48582197751358));
#53185=CARTESIAN_POINT('Ctrl Pts',(-20.9076751313208,1.97078741167024,0.313543614701046));
#53186=CARTESIAN_POINT('Ctrl Pts',(-20.7965287864434,0.80528117489297,1.82587919909306));
#53187=CARTESIAN_POINT('Ctrl Pts',(-20.685382441566,-1.09741073906456,1.66673401900348));
#53188=CARTESIAN_POINT('Ctrl Pts',(-20.5742360966886,-1.99549022192967,
-0.0182042440322412));
#53189=CARTESIAN_POINT('Ctrl Pts',(-20.4630897518111,-1.06682041967049,
-1.68647763474402));
#53190=CARTESIAN_POINT('Ctrl Pts',(-20.3519434069337,0.838458246702548,
-1.81088386951074));
#53191=CARTESIAN_POINT('Ctrl Pts',(-20.2407970620563,1.97617965524583,-0.277536647148052));
#53192=CARTESIAN_POINT('Ctrl Pts',(-20.1296507171789,1.30482942173087,1.50987840586691));
#53193=CARTESIAN_POINT('Ctrl Pts',(-20.0185043723015,-0.561012364366608,
1.91509209891992));
#53194=CARTESIAN_POINT('Ctrl Pts',(-19.907358027424,-1.91328163365087,0.567156072569076));
#53195=CARTESIAN_POINT('Ctrl Pts',(-19.7962116825466,-1.51405855378528,
-1.29997665980099));
#53196=CARTESIAN_POINT('Ctrl Pts',(-19.6850653376692,0.271192555868894,
-1.97706024641613));
#53197=CARTESIAN_POINT('Ctrl Pts',(-19.5739189927918,1.80818346253121,-0.844266063599836));
#53198=CARTESIAN_POINT('Ctrl Pts',(-19.4627726479143,1.68989296953911,1.06140207830021));
#53199=CARTESIAN_POINT('Ctrl Pts',(-19.3516263030369,0.0246087904256447,
1.99542151630965));
#53200=CARTESIAN_POINT('Ctrl Pts',(-19.2404799581595,-1.66320323163278,
1.10275456498897));
#53201=CARTESIAN_POINT('Ctrl Pts',(-19.129333613282,-1.82845439069506,-0.79941676331289));
#53202=CARTESIAN_POINT('Ctrl Pts',(-19.0181872684046,-0.319867354822673,
-1.96977092466014));
#53203=CARTESIAN_POINT('Ctrl Pts',(-18.9070409235272,1.48153868629239,-1.33692024494236));
#53204=CARTESIAN_POINT('Ctrl Pts',(-18.7958945786498,1.92668664790082,0.519799173833923));
#53205=CARTESIAN_POINT('Ctrl Pts',(-18.6847482337724,0.60807078945512,1.90067423177386));
#53206=CARTESIAN_POINT('Ctrl Pts',(-18.5736018888949,-1.26719669661316,
1.54159824611032));
#53207=CARTESIAN_POINT('Ctrl Pts',(-18.4624555440175,-1.98242308891378,
-0.228716673767415));
#53208=CARTESIAN_POINT('Ctrl Pts',(-18.3513091991401,-0.882862357384166,
-1.78965546355487));
#53209=CARTESIAN_POINT('Ctrl Pts',(-18.2401628542626,1.02490488024154,-1.71227410386737));
#53210=CARTESIAN_POINT('Ctrl Pts',(-18.1290165093853,1.99443436720007,-0.0674104980620086));
#53211=CARTESIAN_POINT('Ctrl Pts',(-18.0178701645078,1.13818113947967,1.63916329694466));
#53212=CARTESIAN_POINT('Ctrl Pts',(-17.9067238196304,-0.760007328031514,
1.84518331925479));
#53213=CARTESIAN_POINT('Ctrl Pts',(-17.7955774747529,-1.9624555569219,0.362050835414104));
#53214=CARTESIAN_POINT('Ctrl Pts',(-17.6844311298756,-1.36839571661786,
-1.45251705086709));
#53215=CARTESIAN_POINT('Ctrl Pts',(-17.5732847849981,0.478346732514791,
-1.93739439036303));
#53216=CARTESIAN_POINT('Ctrl Pts',(-17.4621384401207,1.88719199625409,-0.64870562629918));
#53217=CARTESIAN_POINT('Ctrl Pts',(-17.3509920952433,1.56842837864508,1.23383347392527));
#53218=CARTESIAN_POINT('Ctrl Pts',(-17.2398457503659,-0.186135519001358,
1.98687347077861));
#53219=CARTESIAN_POINT('Ctrl Pts',(-17.1286994054884,-1.77030373014666,
0.92105229132037));
#53220=CARTESIAN_POINT('Ctrl Pts',(-17.017553060611,-1.73386712050211,-0.987935943651935));
#53221=CARTESIAN_POINT('Ctrl Pts',(-16.9064067157336,-0.110181178302628,
-1.99252922896141));
#53222=CARTESIAN_POINT('Ctrl Pts',(-16.7952603708562,1.61436889567086,-1.1730838371609));
#53223=CARTESIAN_POINT('Ctrl Pts',(-16.6841140259787,1.8610629552752,0.720248080053035));
#53224=CARTESIAN_POINT('Ctrl Pts',(-16.5729676811013,0.40406767290285,1.95423691911513));
#53225=CARTESIAN_POINT('Ctrl Pts',(-16.4618213362239,-1.42282685753662,
1.3992413493712));
#53226=CARTESIAN_POINT('Ctrl Pts',(-16.3506749913465,-1.94721039779585,
-0.43667411994929));
#53227=CARTESIAN_POINT('Ctrl Pts',(-16.239528646469,-0.689041879884402,
-1.87284113263327));
#53228=CARTESIAN_POINT('Ctrl Pts',(-16.1283823015916,1.19990234800887,-1.59453660213884));
#53229=CARTESIAN_POINT('Ctrl Pts',(-16.0172359567142,1.99040934360917,0.143468690629876));
#53230=CARTESIAN_POINT('Ctrl Pts',(-15.9060896118368,0.958818287520326,
1.75013716943395));
#53231=CARTESIAN_POINT('Ctrl Pts',(-15.7949432669594,-0.950512284424457,
1.75466208070839));
#53232=CARTESIAN_POINT('Ctrl Pts',(-15.6837969220819,-1.98970697848199,
0.152901144854428));
#53233=CARTESIAN_POINT('Ctrl Pts',(-15.5726505772045,-1.20744659317862,
-1.588831440065));
#53234=CARTESIAN_POINT('Ctrl Pts',(-15.4615042323271,0.680157319582284,
-1.87608598975003));
#53235=CARTESIAN_POINT('Ctrl Pts',(-15.3503578874496,1.94511879407684,-0.445898527971097));
#53236=CARTESIAN_POINT('Ctrl Pts',(-15.2392115425722,1.42944294571563,1.39248177196742));
#53237=CARTESIAN_POINT('Ctrl Pts',(-15.1280651976948,-0.394800517016975,
1.95613015213222));
#53238=CARTESIAN_POINT('Ctrl Pts',(-15.0169188528174,-1.85762824626129,
0.729060984424456));
#53239=CARTESIAN_POINT('Ctrl Pts',(-14.9057725079399,-1.61991089961792,
-1.16541893652745));
#53240=CARTESIAN_POINT('Ctrl Pts',(-14.7946261630626,0.100735827145627,
-1.99302907993009));
#53241=CARTESIAN_POINT('Ctrl Pts',(-14.6834798181851,1.72916506358908,-0.99614296322402));
#53242=CARTESIAN_POINT('Ctrl Pts',(-14.5723334733077,1.77464941307702,0.912651127749848));
#53243=CARTESIAN_POINT('Ctrl Pts',(-14.4611871284303,0.195550734766548,
1.98596891477434));
#53244=CARTESIAN_POINT('Ctrl Pts',(-14.3500407835529,-1.56256268439037,
1.24125359120065));
#53245=CARTESIAN_POINT('Ctrl Pts',(-14.2388944386754,-1.89024550794569,
-0.639753499411164));
#53246=CARTESIAN_POINT('Ctrl Pts',(-14.127748093798,-0.487524146904184,
-1.93510537865592));
#53247=CARTESIAN_POINT('Ctrl Pts',(-14.0166017489206,1.36149576125667,-1.4589866045985));
#53248=CARTESIAN_POINT('Ctrl Pts',(-13.9054554040432,1.96414954782845,0.352745197108303));
#53249=CARTESIAN_POINT('Ctrl Pts',(-13.7943090591657,0.768744520108917,
1.84156033925587));
#53250=CARTESIAN_POINT('Ctrl Pts',(-13.6831627142883,-1.13039911134791,
1.64453959191672));
#53251=CARTESIAN_POINT('Ctrl Pts',(-13.5720163694109,-1.99473147394114,
-0.0579565974355843));
#53252=CARTESIAN_POINT('Ctrl Pts',(-13.4608700245335,-1.0330091388004,-1.70739706555697));
#53253=CARTESIAN_POINT('Ctrl Pts',(-13.349723679656,0.874369900188122,-1.7938199179301));
#53254=CARTESIAN_POINT('Ctrl Pts',(-13.2385773347786,1.98131675837734,-0.238110317480801));
#53255=CARTESIAN_POINT('Ctrl Pts',(-13.1274309899012,1.27448927069651,1.53557471950966));
#53256=CARTESIAN_POINT('Ctrl Pts',(-13.0162846450238,-0.599055216425213,
1.90353499258393));
#53257=CARTESIAN_POINT('Ctrl Pts',(-12.9051383001463,-1.92420128178143,
0.528925370452593));
#53258=CARTESIAN_POINT('Ctrl Pts',(-12.7939919552689,-1.48785872779961,
-1.32988308750365));
#53259=CARTESIAN_POINT('Ctrl Pts',(-12.6828456103915,0.310527517253561,
-1.97126489375378));
#53260=CARTESIAN_POINT('Ctrl Pts',(-12.5716992655141,1.82464480727981,-0.808074221581474));
#53261=CARTESIAN_POINT('Ctrl Pts',(-12.4605529206366,1.66841134305336,1.09485899123521));
#53262=CARTESIAN_POINT('Ctrl Pts',(-12.3494065757592,-0.0151506917279239,
1.99551574207219));
#53263=CARTESIAN_POINT('Ctrl Pts',(-12.2382602308818,-1.68484319461224,
1.0693998456548));
#53264=CARTESIAN_POINT('Ctrl Pts',(-12.1271138860044,-1.81216477155529,
-0.835686221647619));
#53265=CARTESIAN_POINT('Ctrl Pts',(-12.0159675411269,-0.280560303867124,
-1.97575265056427));
#53266=CARTESIAN_POINT('Ctrl Pts',(-11.9048211962496,1.50787996731995,-1.30713833409968));
#53267=CARTESIAN_POINT('Ctrl Pts',(-11.7936748513721,1.91594832684148,0.55808120304399));
#53268=CARTESIAN_POINT('Ctrl Pts',(-11.6825285064947,0.570083142650521,
1.91241152234122));
#53269=CARTESIAN_POINT('Ctrl Pts',(-11.5713821616172,-1.29765830124531,
1.51604602619013));
#53270=CARTESIAN_POINT('Ctrl Pts',(-11.4602358167399,-1.97747291488927,
-0.26816690921338));
#53271=CARTESIAN_POINT('Ctrl Pts',(-11.3490894718624,-0.847031986347007,
-1.8068894361368));
#53272=CARTESIAN_POINT('Ctrl Pts',(-11.237943126985,1.05881493443335,-1.69151516544742));
#53273=CARTESIAN_POINT('Ctrl Pts',(-11.1267967821076,1.99538152334385,-0.0276621874708096));
#53274=CARTESIAN_POINT('Ctrl Pts',(-11.0156504372301,1.10529833403908,1.66151383174746));
#53275=CARTESIAN_POINT('Ctrl Pts',(-10.9045040923527,-0.79661789727502,
1.82967553026728));
#53276=CARTESIAN_POINT('Ctrl Pts',(-10.7933577474753,-1.96927915235719,
0.322881155239884));
#53277=CARTESIAN_POINT('Ctrl Pts',(-10.6822114025979,-1.33918575384856,
-1.4794911750351));
#53278=CARTESIAN_POINT('Ctrl Pts',(-10.5710650577204,0.516850318599018,
-1.92747979716568));
#53279=CARTESIAN_POINT('Ctrl Pts',(-10.459918712843,1.89974152687182,-0.610978519586766));
#53280=CARTESIAN_POINT('Ctrl Pts',(-10.3487723679656,1.54353552584929,1.26483623475882));
#53281=CARTESIAN_POINT('Ctrl Pts',(-10.2376260230882,-0.225682870534658,
1.9827707538354));
#53282=CARTESIAN_POINT('Ctrl Pts',(-10.1264796782107,-1.78830239818783,
0.885599883103732));
#53283=CARTESIAN_POINT('Ctrl Pts',(-10.0153333333333,-1.7138404249772,-1.02228353113588));
#53284=CARTESIAN_POINT('Ctrl Pts',(-9.9041869884559,-0.07046233444443,-1.99432887953376));
#53285=CARTESIAN_POINT('Ctrl Pts',(-9.79304064357848,1.63741971489506,-1.1406880807612));
#53286=CARTESIAN_POINT('Ctrl Pts',(-9.68189429870107,1.84634413429414,0.757182909259928));
#53287=CARTESIAN_POINT('Ctrl Pts',(-9.57074795382363,0.365053392351222,
1.96189924334829));
#53288=CARTESIAN_POINT('Ctrl Pts',(-9.45960160894621,-1.4504214093186,1.37061677930337));
#53289=CARTESIAN_POINT('Ctrl Pts',(-9.3484552640688,-1.93812409590406,-0.475381540653165));
#53290=CARTESIAN_POINT('Ctrl Pts',(-9.23730891919136,-0.651592678124332,
-1.88619712706082));
#53291=CARTESIAN_POINT('Ctrl Pts',(-9.12616257431395,1.23143199523488,-1.5703145740359));
#53292=CARTESIAN_POINT('Ctrl Pts',(-9.01501622943651,1.98715597212704,0.183094955576432));
#53293=CARTESIAN_POINT('Ctrl Pts',(-8.9038698845591,0.923760159996531,1.76889224858976));
#53294=CARTESIAN_POINT('Ctrl Pts',(-8.79272353968166,-0.985281595850083,
1.73537684587435));
#53295=CARTESIAN_POINT('Ctrl Pts',(-8.68157719480427,-1.99235829514795,
0.113230049337008));
#53296=CARTESIAN_POINT('Ctrl Pts',(-8.57043084992681,-1.17555279679042,
-1.61257193398495));
#53297=CARTESIAN_POINT('Ctrl Pts',(-8.45928450504942,0.717399408558318,
-1.86216291148704));
#53298=CARTESIAN_POINT('Ctrl Pts',(-8.34813816017196,1.9536163203283,-0.407057604356679));
#53299=CARTESIAN_POINT('Ctrl Pts',(-8.23699181529457,1.40141694353548,1.42068405026924));
#53300=CARTESIAN_POINT('Ctrl Pts',(-8.12584547041712,-0.433693956265927,
1.94787632374751));
#53301=CARTESIAN_POINT('Ctrl Pts',(-8.01469912553972,-1.8717845570626,0.691906924564031));
#53302=CARTESIAN_POINT('Ctrl Pts',(-7.90355278066229,-1.59637084501215,
-1.19746095782407));
#53303=CARTESIAN_POINT('Ctrl Pts',(-7.79240643578486,0.140422766509441,
-1.99062655135601));
#53304=CARTESIAN_POINT('Ctrl Pts',(-7.68126009090745,1.74866792135743,-0.961495252787647));
#53305=CARTESIAN_POINT('Ctrl Pts',(-7.57011374603,1.75611451545356,0.947826159657482));
#53306=CARTESIAN_POINT('Ctrl Pts',(-7.4589674011526,0.155945647220306,1.98947067719803));
#53307=CARTESIAN_POINT('Ctrl Pts',(-7.34782105627516,-1.58698192584009,
1.20987643475463));
#53308=CARTESIAN_POINT('Ctrl Pts',(-7.23667471139775,-1.87712458085155,
-0.677285706537936));
#53309=CARTESIAN_POINT('Ctrl Pts',(-7.12552836652031,-0.448874457749643,
-1.9444341957232));
#53310=CARTESIAN_POINT('Ctrl Pts',(-7.0143820216429,1.39029278526267,-1.43157206998609));
#53311=CARTESIAN_POINT('Ctrl Pts',(-6.90323567676547,1.95673199198518,0.391806753207983));
#53312=CARTESIAN_POINT('Ctrl Pts',(-6.79208933188805,0.731902703248883,
1.85651045062901));
#53313=CARTESIAN_POINT('Ctrl Pts',(-6.68094298701063,-1.16293875856013,
1.62169234571676));
#53314=CARTESIAN_POINT('Ctrl Pts',(-6.5697966421332,-1.99318089409997,-0.0976859442937018));
#53315=CARTESIAN_POINT('Ctrl Pts',(-6.45865029725579,-0.998787792941156,
-1.72763872525175));
#53316=CARTESIAN_POINT('Ctrl Pts',(-6.34750395237835,0.909934462374966,
-1.77604388867507));
#53317=CARTESIAN_POINT('Ctrl Pts',(-6.23635760750093,1.98566735478354,-0.198589467154337));
#53318=CARTESIAN_POINT('Ctrl Pts',(-6.12521126262351,1.2436431963268,1.5606614689124));
#53319=CARTESIAN_POINT('Ctrl Pts',(-6.01406491774608,-0.63686026655008,
1.89122225589894));
#53320=CARTESIAN_POINT('Ctrl Pts',(-5.90291857286866,-1.93435709583923,
0.490484705260119));
#53321=CARTESIAN_POINT('Ctrl Pts',(-5.79177222799124,-1.4610682789916,-1.35926160265134));
#53322=CARTESIAN_POINT('Ctrl Pts',(-5.6806258831138,0.349739211129583,-1.96468702457062));
#53323=CARTESIAN_POINT('Ctrl Pts',(-5.5694795382364,1.84038183805583,-0.77156160510482));
#53324=CARTESIAN_POINT('Ctrl Pts',(-5.45833319335896,1.64626742128525,1.12788128716304));
#53325=CARTESIAN_POINT('Ctrl Pts',(-5.34718684848155,-0.0549041596382843,
1.99481782465771));
#53326=CARTESIAN_POINT('Ctrl Pts',(-5.23604050360411,-1.70581433949485,
1.03562061561725));
#53327=CARTESIAN_POINT('Ctrl Pts',(-5.12489415872671,-1.7951557925382,-0.871623944619641));
#53328=CARTESIAN_POINT('Ctrl Pts',(-5.01374781384927,-0.241141881236654,
-1.98095007848036));
#53329=CARTESIAN_POINT('Ctrl Pts',(-4.90260146897185,1.53362267786139,-1.2768375394963));
#53330=CARTESIAN_POINT('Ctrl Pts',(-4.79145512409443,1.90444944781581,0.596141695431386));
#53331=CARTESIAN_POINT('Ctrl Pts',(-4.680308779217,0.53186919471367,1.92338965891789));
#53332=CARTESIAN_POINT('Ctrl Pts',(-4.56916243433959,-1.32760478532606,
1.48989199417179));
#53333=CARTESIAN_POINT('Ctrl Pts',(-4.45801608946215,-1.97173775999777,
-0.307510692686641));
#53334=CARTESIAN_POINT('Ctrl Pts',(-4.34686974458474,-0.810865376113923,
-1.82340614294705));
#53335=CARTESIAN_POINT('Ctrl Pts',(-4.2357233997073,1.09230467972553,-1.67008476041437));
#53336=CARTESIAN_POINT('Ctrl Pts',(-4.12457705482989,1.99553658959009,0.0120971039477285));
#53337=CARTESIAN_POINT('Ctrl Pts',(-4.01343070995246,1.07197676757322,1.68320480931454));
#53338=CARTESIAN_POINT('Ctrl Pts',(-3.90228436507504,-0.832912239782294,
1.81344143030452));
#53339=CARTESIAN_POINT('Ctrl Pts',(-3.79113802019761,-1.97532101953316,
0.283583303634182));
#53340=CARTESIAN_POINT('Ctrl Pts',(-3.67999167532019,-1.30944418572589,
-1.50587799797332));
#53341=CARTESIAN_POINT('Ctrl Pts',(-3.56884533044276,0.555148734945638,
-1.91680006845999));
#53342=CARTESIAN_POINT('Ctrl Pts',(-3.45769898556535,1.91153693298929,-0.573008877829148));
#53343=CARTESIAN_POINT('Ctrl Pts',(-3.34655264068792,1.51802994870092,1.29533690410844));
#53344=CARTESIAN_POINT('Ctrl Pts',(-3.2354062958105,-0.265140634670444,
1.97788095305015));
#53345=CARTESIAN_POINT('Ctrl Pts',(-3.12425995093307,-1.80559117871824,
0.84979592559486));
#53346=CARTESIAN_POINT('Ctrl Pts',(-3.01311360605565,-1.69313340071988,
-1.05622531105494));
#53347=CARTESIAN_POINT('Ctrl Pts',(-2.90196726117823,-0.0307155194536576,
-1.99533685850639));
#53348=CARTESIAN_POINT('Ctrl Pts',(-2.7908209163008,1.65982054077328,-1.10783951413039));
#53349=CARTESIAN_POINT('Ctrl Pts',(-2.67967457142338,1.83089238658801,0.793817164320537));
#53350=CARTESIAN_POINT('Ctrl Pts',(-2.56852822654595,0.325894197617876,
1.96878277188174));
#53351=CARTESIAN_POINT('Ctrl Pts',(-2.45738188166853,-1.47744019566639,
1.34144812122869));
#53352=CARTESIAN_POINT('Ctrl Pts',(-2.34623553679111,-1.92826844032713,
-0.513900242210063));
#53353=CARTESIAN_POINT('Ctrl Pts',(-2.23508919191368,-0.613884805358574,
-1.89880439437223));
#53354=CARTESIAN_POINT('Ctrl Pts',(-2.12394284703626,1.2624727851227,-1.54546915180465));
#53355=CARTESIAN_POINT('Ctrl Pts',(-2.01279650215884,1.98311382560099,0.222648463718466));
#53356=CARTESIAN_POINT('Ctrl Pts',(-1.90165015728141,0.888335240741561,
1.78694528831349));
#53357=CARTESIAN_POINT('Ctrl Pts',(-1.790503812404,-1.01965960873761,1.71540246117927));
#53358=CARTESIAN_POINT('Ctrl Pts',(-1.67935746752656,-1.9942190635569,0.0735145229216604));
#53359=CARTESIAN_POINT('Ctrl Pts',(-1.56821112264915,-1.14319170140108,
-1.6356732823008));
#53360=CARTESIAN_POINT('Ctrl Pts',(-1.45706477777171,0.754355481768247,
-1.84749875509779));
#53361=CARTESIAN_POINT('Ctrl Pts',(-1.3459184328943,1.96134068640505,-0.368058653232534));
#53362=CARTESIAN_POINT('Ctrl Pts',(-1.23477208801687,1.3728301615305,1.44832914076707));
#53363=CARTESIAN_POINT('Ctrl Pts',(-1.12362574313945,-0.472406731010585,
1.93883638708916));
#53364=CARTESIAN_POINT('Ctrl Pts',(-1.01247939826202,-1.88521401833496,
0.654502696535881));
#53365=CARTESIAN_POINT('Ctrl Pts',(-0.901333053384601,-1.57216632097497,
-1.22907422156167));
#53366=CARTESIAN_POINT('Ctrl Pts',(-0.790186708507175,0.179995429844686,
-1.98734519828315));
#53367=CARTESIAN_POINT('Ctrl Pts',(-0.679040363629751,1.76758797928351,
-0.926634471973894));
#53368=CARTESIAN_POINT('Ctrl Pts',(-0.567894018752328,1.73667056918864,
0.982945946718963));
#53369=CARTESIAN_POINT('Ctrl Pts',(-0.456747673874906,0.116682879679813,
1.99156959023754));
#53370=CARTESIAN_POINT('Ctrl Pts',(-0.345601328997482,-1.61154942417229,
1.17920674007046));
#53371=CARTESIAN_POINT('Ctrl Pts',(-0.234454984120056,-1.86169777943505,
-0.71699198523252));
#53372=CARTESIAN_POINT('Ctrl Pts',(-0.160357420868444,-0.896388758474477,
-1.53694076122322));
#53373=CARTESIAN_POINT('Ctrl Pts',(-0.123308639242636,-0.346915509926856,
-1.652307197048));
#53374=CARTESIAN_POINT('Ctrl Pts',(-29.7226913607574,-0.802959149489686,
1.63459616787406));
#53375=CARTESIAN_POINT('Ctrl Pts',(-29.6856425791315,-1.34654261146935,
1.36757283643219));
#53376=CARTESIAN_POINT('Ctrl Pts',(-29.6115450158799,-2.13699697723614,
0.253271596645648));
#53377=CARTESIAN_POINT('Ctrl Pts',(-29.5003986710025,-1.37018370663775,
-1.66203790618904));
#53378=CARTESIAN_POINT('Ctrl Pts',(-29.3892523261251,0.652727265457014,
-2.05056399477137));
#53379=CARTESIAN_POINT('Ctrl Pts',(-29.2781059812477,2.07719244398607,-0.56457687295854));
#53380=CARTESIAN_POINT('Ctrl Pts',(-29.1669596363702,1.60059299295594,1.43962549295637));
#53381=CARTESIAN_POINT('Ctrl Pts',(-29.0558132914928,-0.341502513910902,
2.12521518253081));
#53382=CARTESIAN_POINT('Ctrl Pts',(-28.9446669466154,-1.9708414067249,0.865680507114811));
#53383=CARTESIAN_POINT('Ctrl Pts',(-28.8335206017379,-1.7960648593605,-1.18653159130759));
#53384=CARTESIAN_POINT('Ctrl Pts',(-28.7223742568606,0.0229357119706541,
-2.15244150481461));
#53385=CARTESIAN_POINT('Ctrl Pts',(-28.6112279119831,1.82092087124584,-1.14797806388266));
#53386=CARTESIAN_POINT('Ctrl Pts',(-28.5000815671057,1.95197439015737,0.907418139493177));
#53387=CARTESIAN_POINT('Ctrl Pts',(-28.3889352222283,0.296109408884188,
2.13211325412446));
#53388=CARTESIAN_POINT('Ctrl Pts',(-28.2777888773509,-1.63082284536082,
1.40499707683198));
#53389=CARTESIAN_POINT('Ctrl Pts',(-28.1666425324734,-2.06483796472262,
-0.608312235744213));
#53390=CARTESIAN_POINT('Ctrl Pts',(-28.055496187596,-0.60861941081362,-2.0647466732867));
#53391=CARTESIAN_POINT('Ctrl Pts',(-27.9443498427186,1.40475259530209,-1.6310329452328));
#53392=CARTESIAN_POINT('Ctrl Pts',(-27.8332034978412,2.13215970594569,0.295792328695355));
#53393=CARTESIAN_POINT('Ctrl Pts',(-27.7220571529637,0.907704863562922,
1.95183748945672));
#53394=CARTESIAN_POINT('Ctrl Pts',(-27.6109108080863,-1.14769822153575,
1.82109494198778));
#53395=CARTESIAN_POINT('Ctrl Pts',(-27.4997644632089,-2.15245379105352,
0.0232512358109067));
#53396=CARTESIAN_POINT('Ctrl Pts',(-27.3886181183314,-1.1867695091042,-1.79587750823898));
#53397=CARTESIAN_POINT('Ctrl Pts',(-27.2774717734541,0.865329685575796,
-1.97099022596782));
#53398=CARTESIAN_POINT('Ctrl Pts',(-27.1663254285766,2.12527246766768,-0.341781893895144));
#53399=CARTESIAN_POINT('Ctrl Pts',(-27.0551790836992,1.43965825175809,1.60030685718542));
#53400=CARTESIAN_POINT('Ctrl Pts',(-26.9440327388218,-0.563875065354492,
2.07741253389249));
#53401=CARTESIAN_POINT('Ctrl Pts',(-26.8328863939443,-2.05121523859028,
0.652774056083331));
#53402=CARTESIAN_POINT('Ctrl Pts',(-26.721740049067,-1.66079328087856,-1.36943915560345));
#53403=CARTESIAN_POINT('Ctrl Pts',(-26.6105937041895,0.249983377088396,
-2.13801455439055));
#53404=CARTESIAN_POINT('Ctrl Pts',(-26.4994473593121,1.93191553850937,-0.949368355976965));
#53405=CARTESIAN_POINT('Ctrl Pts',(-26.3883010144347,1.84529715019161,1.10836652363136));
#53406=CARTESIAN_POINT('Ctrl Pts',(-26.2771546695572,0.0694220504867175,
2.15145962133678));
#53407=CARTESIAN_POINT('Ctrl Pts',(-26.1660083246798,-1.77000469168292,
1.22502298537633));
#53408=CARTESIAN_POINT('Ctrl Pts',(-26.0548619798024,-1.98910036448447,
-0.822847290379835));
#53409=CARTESIAN_POINT('Ctrl Pts',(-25.943715634925,-0.387296275952628,
-2.1174511843081));
#53410=CARTESIAN_POINT('Ctrl Pts',(-25.8325692900475,1.56905387221744,-1.47365798927873));
#53411=CARTESIAN_POINT('Ctrl Pts',(-25.7214229451701,2.08903113922897,0.519178988998727));
#53412=CARTESIAN_POINT('Ctrl Pts',(-25.6102766002927,0.696628130832529,
2.03673934773722));
#53413=CARTESIAN_POINT('Ctrl Pts',(-25.4991302554153,-1.3334953364323,1.68978936882682));
#53414=CARTESIAN_POINT('Ctrl Pts',(-25.3879839105379,-2.14288535896546,
-0.204059456087));
#53415=CARTESIAN_POINT('Ctrl Pts',(-25.2768375656604,-0.990594860805363,
-1.91110432604642));
#53416=CARTESIAN_POINT('Ctrl Pts',(-25.165691220783,1.06852466309368,-1.86865003883757));
#53417=CARTESIAN_POINT('Ctrl Pts',(-25.0545448759056,2.14947519222985,-0.115560898558425));
#53418=CARTESIAN_POINT('Ctrl Pts',(-24.9433985310282,1.26271261125054,1.74331717844919));
#53419=CARTESIAN_POINT('Ctrl Pts',(-24.8322521861507,-0.779986157523649,
2.00629497266944));
#53420=CARTESIAN_POINT('Ctrl Pts',(-24.7211058412733,-2.10865529087055,
0.432632393113157));
#53421=CARTESIAN_POINT('Ctrl Pts',(-24.6099594963959,-1.50697943788803,
-1.53707868929012));
#53422=CARTESIAN_POINT('Ctrl Pts',(-24.4988131515184,0.474243947127435,
-2.09968821540251));
#53423=CARTESIAN_POINT('Ctrl Pts',(-24.3876668066411,2.02132599590933,-0.740161564490013));
#53424=CARTESIAN_POINT('Ctrl Pts',(-24.2765204617636,1.71800768820146,1.29693774197832));
#53425=CARTESIAN_POINT('Ctrl Pts',(-24.1653741168862,-0.158041611505553,
2.14676984614558));
#53426=CARTESIAN_POINT('Ctrl Pts',(-24.0542277720087,-1.88941347923875,
1.03136541912073));
#53427=CARTESIAN_POINT('Ctrl Pts',(-23.9430814271314,-1.89114283378241,
-1.0281909868894));
#53428=CARTESIAN_POINT('Ctrl Pts',(-23.8319350822539,-0.161646556792161,
-2.14650141252327));
#53429=CARTESIAN_POINT('Ctrl Pts',(-23.7207887373765,1.71582725915959,-1.29982104153306));
#53430=CARTESIAN_POINT('Ctrl Pts',(-23.6096423924991,2.02256613257899,0.73676601620298));
#53431=CARTESIAN_POINT('Ctrl Pts',(-23.4984960476216,0.477769380214973,
2.09888883522119));
#53432=CARTESIAN_POINT('Ctrl Pts',(-23.3873497027443,-1.50439602681377,
1.53960726089289));
#53433=CARTESIAN_POINT('Ctrl Pts',(-23.2762033578667,-2.10937885668692,
-0.42909062242064));
#53434=CARTESIAN_POINT('Ctrl Pts',(-23.1650570129894,-0.783354319967773,
-2.00498227739674));
#53435=CARTESIAN_POINT('Ctrl Pts',(-23.0539106681119,1.259783198952,-1.74543525085448));
#53436=CARTESIAN_POINT('Ctrl Pts',(-22.9427643232346,2.14966622791904,0.111951024253906));
#53437=CARTESIAN_POINT('Ctrl Pts',(-22.8316179783571,1.0716612652779,1.86685298183605));
#53438=CARTESIAN_POINT('Ctrl Pts',(-22.7204716334797,-0.987384059640079,
1.91276518215275));
#53439=CARTESIAN_POINT('Ctrl Pts',(-22.6093252886022,-2.14253965096347,
0.207657813088019));
#53440=CARTESIAN_POINT('Ctrl Pts',(-22.4981789437248,-1.33633119613124,
-1.68754758674641));
#53441=CARTESIAN_POINT('Ctrl Pts',(-22.3870325988474,0.693206759589962,
-2.03790635499916));
#53442=CARTESIAN_POINT('Ctrl Pts',(-22.27588625397,2.08815631261794,-0.522686461811507));
#53443=CARTESIAN_POINT('Ctrl Pts',(-22.1647399090925,1.57152644050903,1.47102092781448));
#53444=CARTESIAN_POINT('Ctrl Pts',(-22.0535935642152,-0.383739797844597,
2.11809860271834));
#53445=CARTESIAN_POINT('Ctrl Pts',(-21.9424472193377,-1.9877157148112,0.826186516701757));
#53446=CARTESIAN_POINT('Ctrl Pts',(-21.8313008744603,-1.77205943255289,
-1.22204880867642));
#53447=CARTESIAN_POINT('Ctrl Pts',(-21.7201545295828,0.0658089086968051,
-2.15157317115252));
#53448=CARTESIAN_POINT('Ctrl Pts',(-21.6090081847055,1.84343321788083,-1.11146385208909));
#53449=CARTESIAN_POINT('Ctrl Pts',(-21.497861839828,1.93350713171299,0.946122663771537));
#53450=CARTESIAN_POINT('Ctrl Pts',(-21.3867154949506,0.253573489595389,
2.13759173105193));
#53451=CARTESIAN_POINT('Ctrl Pts',(-21.2755691500732,-1.65849117764792,
1.37222627031812));
#53452=CARTESIAN_POINT('Ctrl Pts',(-21.1644228051957,-2.05230857920252,
-0.649328436939962));
#53453=CARTESIAN_POINT('Ctrl Pts',(-21.0532764603183,-0.567362963673909,
-2.07646266297719));
#53454=CARTESIAN_POINT('Ctrl Pts',(-20.9421301154409,1.43696875403018,-1.60272228512245));
#53455=CARTESIAN_POINT('Ctrl Pts',(-20.8309837705635,2.12584344001191,0.3382123472694));
#53456=CARTESIAN_POINT('Ctrl Pts',(-20.7198374256861,0.868638440084387,
1.96953425552716));
#53457=CARTESIAN_POINT('Ctrl Pts',(-20.6086910808086,-1.18375193936417,
1.79786797884015));
#53458=CARTESIAN_POINT('Ctrl Pts',(-20.4975447359312,-2.1524897981269,-0.0196365029161898));
#53459=CARTESIAN_POINT('Ctrl Pts',(-20.3863983910538,-1.15075485940167,
-1.81916496691493));
#53460=CARTESIAN_POINT('Ctrl Pts',(-20.2752520461764,0.904425790890365,
-1.95335913545346));
#53461=CARTESIAN_POINT('Ctrl Pts',(-20.1641057012989,2.1316599301946,-0.299372452456672));
#53462=CARTESIAN_POINT('Ctrl Pts',(-20.0529593564215,1.40748974247311,1.62867140581522));
#53463=CARTESIAN_POINT('Ctrl Pts',(-19.9418130115441,-0.605151244366693,
2.06576617619918));
#53464=CARTESIAN_POINT('Ctrl Pts',(-19.8306666666667,-2.06381326859854,
0.611778322306184));
#53465=CARTESIAN_POINT('Ctrl Pts',(-19.7195203217892,-1.63318043605245,
-1.40225517883968));
#53466=CARTESIAN_POINT('Ctrl Pts',(-19.6083739769118,0.292529225861806,
-2.13260980380937));
#53467=CARTESIAN_POINT('Ctrl Pts',(-19.4972276320344,1.95044626802358,-0.91069055053848));
#53468=CARTESIAN_POINT('Ctrl Pts',(-19.386081287157,1.82284901067655,1.1449102181231));
#53469=CARTESIAN_POINT('Ctrl Pts',(-19.2749349422795,0.0265449410641972,
2.15241568694131));
#53470=CARTESIAN_POINT('Ctrl Pts',(-19.1637885974022,-1.79405939901794,
1.1895162025305));
#53471=CARTESIAN_POINT('Ctrl Pts',(-19.0526422525247,-1.97231205598467,
-0.862312633042507));
#53472=CARTESIAN_POINT('Ctrl Pts',(-18.9414959076473,-0.345033621534715,
-2.12474697865364));
#53473=CARTESIAN_POINT('Ctrl Pts',(-18.8303495627699,1.5981019965565,-1.44210538168655));
#53474=CARTESIAN_POINT('Ctrl Pts',(-18.7192032178924,2.07827295178796,0.560695515546295));
#53475=CARTESIAN_POINT('Ctrl Pts',(-18.608056873015,0.655912094410212,2.05021395168738));
#53476=CARTESIAN_POINT('Ctrl Pts',(-18.4969105281376,-1.36689618004863,
1.66288687416061));
#53477=CARTESIAN_POINT('Ctrl Pts',(-18.3857641832601,-2.13839457971973,
-0.246711460440006));
#53478=CARTESIAN_POINT('Ctrl Pts',(-18.2746178383827,-0.952323492510973,
-1.93046053803202));
#53479=CARTESIAN_POINT('Ctrl Pts',(-18.1634714935053,1.10554152284303,-1.84699102990705));
#53480=CARTESIAN_POINT('Ctrl Pts',(-18.0523251486279,2.15135087170732,-0.0727141670605007));
#53481=CARTESIAN_POINT('Ctrl Pts',(-17.9411788037505,1.22773004058181,1.76812806966582));
#53482=CARTESIAN_POINT('Ctrl Pts',(-17.830032458873,-0.819802573879665,
1.99035716974302));
#53483=CARTESIAN_POINT('Ctrl Pts',(-17.7188861139956,-2.11685605829079,
0.390535980115425));
#53484=CARTESIAN_POINT('Ctrl Pts',(-17.6077397691182,-1.47605725523029,
-1.56679702021966));
#53485=CARTESIAN_POINT('Ctrl Pts',(-17.4965934242408,0.515981712358321,
-2.08982314940737));
#53486=CARTESIAN_POINT('Ctrl Pts',(-17.3854470793633,2.03567097167509,-0.699743966295212));
#53487=CARTESIAN_POINT('Ctrl Pts',(-17.2743007344859,1.69182792630349,1.33090803253524));
#53488=CARTESIAN_POINT('Ctrl Pts',(-17.1631543896085,-0.200780139795509,
2.14319510515279));
#53489=CARTESIAN_POINT('Ctrl Pts',(-17.0520080447311,-1.90958626449289,
0.993518103381745));
#53490=CARTESIAN_POINT('Ctrl Pts',(-16.9408616998537,-1.87028292455343,
-1.06566397396696));
#53491=CARTESIAN_POINT('Ctrl Pts',(-16.8297153549762,-0.118849924512552,
-2.14929584253321));
#53492=CARTESIAN_POINT('Ctrl Pts',(-16.7185690100988,1.74138291441223,-1.26537878466501));
#53493=CARTESIAN_POINT('Ctrl Pts',(-16.6074226652214,2.0074861710061,0.776915179737431));
#53494=CARTESIAN_POINT('Ctrl Pts',(-16.496276320344,0.435858584581321,2.10799080110278));
#53495=CARTESIAN_POINT('Ctrl Pts',(-16.3851299754665,-1.53477088571601,
1.50932973589128));
#53496=CARTESIAN_POINT('Ctrl Pts',(-16.2739836305891,-2.1004114527853,-0.471030415467579));
#53497=CARTESIAN_POINT('Ctrl Pts',(-16.1628372857117,-0.743253763227663,
-2.020191022338));
#53498=CARTESIAN_POINT('Ctrl Pts',(-16.0516909408343,1.29430730075948,-1.71999027162594));
#53499=CARTESIAN_POINT('Ctrl Pts',(-15.9405445959568,2.14700917054466,0.15475640498651));
#53500=CARTESIAN_POINT('Ctrl Pts',(-15.8293982510794,1.03425542228371,1.88783305532134));
#53501=CARTESIAN_POINT('Ctrl Pts',(-15.718251906202,-1.02529592615071,1.89271397392895));
#53502=CARTESIAN_POINT('Ctrl Pts',(-15.6071055613246,-2.1462515452984,0.16493097826492));
#53503=CARTESIAN_POINT('Ctrl Pts',(-15.4959592164472,-1.30244510598838,
-1.71383624339494));
#53504=CARTESIAN_POINT('Ctrl Pts',(-15.3848128715697,0.733670190629446,
-2.02369117571553));
#53505=CARTESIAN_POINT('Ctrl Pts',(-15.2736665266923,2.09815528754964,-0.480980574051286));
#53506=CARTESIAN_POINT('Ctrl Pts',(-15.1625201818149,1.54190750916428,1.5020383338883));
#53507=CARTESIAN_POINT('Ctrl Pts',(-15.0513738369374,-0.425862314851449,
2.11003298838585));
#53508=CARTESIAN_POINT('Ctrl Pts',(-14.94022749206,-2.00378122871642,0.786421458717215));
#53509=CARTESIAN_POINT('Ctrl Pts',(-14.8290811471826,-1.74736094769246,
-1.2571108311388));
#53510=CARTESIAN_POINT('Ctrl Pts',(-14.7179348023052,0.108661439607204,
-2.14983502037473));
#53511=CARTESIAN_POINT('Ctrl Pts',(-14.6067884574278,1.86521092298501,-1.07451669883004));
#53512=CARTESIAN_POINT('Ctrl Pts',(-14.4956421125503,1.91427385357279,0.984455959814731));
#53513=CARTESIAN_POINT('Ctrl Pts',(-14.3844957676729,0.210936118340905,
2.14221938121809));
#53514=CARTESIAN_POINT('Ctrl Pts',(-14.2733494227955,-1.68550073566969,
1.33891194383504));
#53515=CARTESIAN_POINT('Ctrl Pts',(-14.1622030779181,-2.03896472510586,
-0.690087511161547));
#53516=CARTESIAN_POINT('Ctrl Pts',(-14.0510567330406,-0.525881179982363,
-2.08735404467654));
#53517=CARTESIAN_POINT('Ctrl Pts',(-13.9399103881632,1.46861443072578,-1.57377558030083));
#53518=CARTESIAN_POINT('Ctrl Pts',(-13.8287640432858,2.11868332765266,0.380498200276715));
#53519=CARTESIAN_POINT('Ctrl Pts',(-13.7176176984084,0.829227183734402,
1.98644914383506));
#53520=CARTESIAN_POINT('Ctrl Pts',(-13.606471353531,-1.2193357442941,1.77392735645346));
#53521=CARTESIAN_POINT('Ctrl Pts',(-13.4953250086535,-2.15167135397382,
-0.0625164600374452));
#53522=CARTESIAN_POINT('Ctrl Pts',(-13.3841786637761,-1.11428340174446,
-1.8417302798955));
#53523=CARTESIAN_POINT('Ctrl Pts',(-13.2730323188987,0.943162872591929,
-1.93495264000216));
#53524=CARTESIAN_POINT('Ctrl Pts',(-13.1618859740213,2.13720120619835,-0.256844169705039));
#53525=CARTESIAN_POINT('Ctrl Pts',(-13.0507396291438,1.37476251341562,1.65638943337438));
#53526=CARTESIAN_POINT('Ctrl Pts',(-12.9395932842664,-0.646187201370086,
2.05329978913764));
#53527=CARTESIAN_POINT('Ctrl Pts',(-12.828446939389,-2.07559204403019,0.570539735729004));
#53528=CARTESIAN_POINT('Ctrl Pts',(-12.7173005945115,-1.60491928121084,
-1.4345145604297));
#53529=CARTESIAN_POINT('Ctrl Pts',(-12.6061542496342,0.334958951730538,
-2.12635848904713));
#53530=CARTESIAN_POINT('Ctrl Pts',(-12.4950079047567,1.96820274522673,-0.871651235855885));
#53531=CARTESIAN_POINT('Ctrl Pts',(-12.3838615598793,1.7996772700438,1.18099942716957));
#53532=CARTESIAN_POINT('Ctrl Pts',(-12.2727152150019,-0.0163427056773679,
2.15251732612268));
#53533=CARTESIAN_POINT('Ctrl Pts',(-12.1615688701244,-1.81740193361583,
1.15353722739085));
#53534=CARTESIAN_POINT('Ctrl Pts',(-12.050422525247,-1.9547408152798,-0.901435670675633));
#53535=CARTESIAN_POINT('Ctrl Pts',(-11.9392761803696,-0.302634002009415,
-2.13119932998182));
#53536=CARTESIAN_POINT('Ctrl Pts',(-11.8281298354922,1.62651573572611,-1.40998031359395));
#53537=CARTESIAN_POINT('Ctrl Pts',(-11.7169834906148,2.06668976973314,0.60198946748888));
#53538=CARTESIAN_POINT('Ctrl Pts',(-11.6058371457373,0.614935686055437,
2.06287469937045));
#53539=CARTESIAN_POINT('Ctrl Pts',(-11.4946908008599,-1.39975441833248,
1.63532427721413));
#53540=CARTESIAN_POINT('Ctrl Pts',(-11.3835444559825,-2.13305493988104,
-0.289265529810001));
#53541=CARTESIAN_POINT('Ctrl Pts',(-11.2723981111051,-0.913674088332984,
-1.94905043126032));
#53542=CARTESIAN_POINT('Ctrl Pts',(-11.1612517662276,1.14211952503,-1.82459883641102));
#53543=CARTESIAN_POINT('Ctrl Pts',(-11.0501054213502,2.15237254744109,-0.0298385708285128));
#53544=CARTESIAN_POINT('Ctrl Pts',(-10.9389590764728,1.19226010819787,1.79223708188598));
#53545=CARTESIAN_POINT('Ctrl Pts',(-10.8278127315954,-0.859293560071549,
1.9736292713949));
#53546=CARTESIAN_POINT('Ctrl Pts',(-10.7166663867179,-2.12421651508461,
0.348284539319401));
#53547=CARTESIAN_POINT('Ctrl Pts',(-10.6055200418405,-1.44454913448201,
-1.5958933928538));
#53548=CARTESIAN_POINT('Ctrl Pts',(-10.4943736969631,0.557514652648782,
-2.07912850381334));
#53549=CARTESIAN_POINT('Ctrl Pts',(-10.3832273520857,2.04920786417854,-0.659048596596637));
#53550=CARTESIAN_POINT('Ctrl Pts',(-10.2720810072083,1.66497657363818,1.36435000367326));
#53551=CARTESIAN_POINT('Ctrl Pts',(-10.1609346623308,-0.243438966074324,
2.13876959794267));
#53552=CARTESIAN_POINT('Ctrl Pts',(-10.0497883174534,-1.9290010172753,0.955276399079356));
#53553=CARTESIAN_POINT('Ctrl Pts',(-9.93864197257598,-1.84868058477054,
-1.10271393333884));
#53554=CARTESIAN_POINT('Ctrl Pts',(-9.82749562769855,-0.0760061133735042,
-2.15123708456717));
#53555=CARTESIAN_POINT('Ctrl Pts',(-9.71634928282113,1.76624730746878,-1.23043422097504));
#53556=CARTESIAN_POINT('Ctrl Pts',(-9.60520293794371,1.99160931445526,0.816755937757542));
#53557=CARTESIAN_POINT('Ctrl Pts',(-9.49405659306628,0.393774769814524,
2.11625597552487));
#53558=CARTESIAN_POINT('Ctrl Pts',(-9.38291024818886,-1.56453649946938,
1.47845306490103));
#53559=CARTESIAN_POINT('Ctrl Pts',(-9.27176390331143,-2.0906102661346,-0.512783227514099));
#53560=CARTESIAN_POINT('Ctrl Pts',(-9.16061755843402,-0.70285816326396,
-2.03459782896287));
#53561=CARTESIAN_POINT('Ctrl Pts',(-9.04947121355658,1.32831761223416,-1.69386252225961));
#53562=CARTESIAN_POINT('Ctrl Pts',(-8.93832486867917,2.14349983291531,0.197500353364697));
#53563=CARTESIAN_POINT('Ctrl Pts',(-8.82717852380173,0.996439019573689,
1.90806373152424));
#53564=CARTESIAN_POINT('Ctrl Pts',(-8.71603217892433,-1.06280078952167,
1.87191143088536));
#53565=CARTESIAN_POINT('Ctrl Pts',(-8.60488583404689,-2.14911146012652,
0.122138672172239));
#53566=CARTESIAN_POINT('Ctrl Pts',(-8.49373948916947,-1.26804199511632,
-1.73944457281875));
#53567=CARTESIAN_POINT('Ctrl Pts',(-8.38259314429205,0.773842382755913,
-2.0086726686889));
#53568=CARTESIAN_POINT('Ctrl Pts',(-8.27144679941462,2.10732137534329,-0.439083755459502));
#53569=CARTESIAN_POINT('Ctrl Pts',(-8.16030045453719,1.511676499705,1.53245948838031));
#53570=CARTESIAN_POINT('Ctrl Pts',(-8.04915410965979,-0.46781578086066,
2.10112977192388));
#53571=CARTESIAN_POINT('Ctrl Pts',(-7.93800776478234,-2.0190513183636,0.746344221590376));
#53572=CARTESIAN_POINT('Ctrl Pts',(-7.82686141990494,-1.72196882758612,
-1.2916738288395));
#53573=CARTESIAN_POINT('Ctrl Pts',(-7.71571507502751,0.151470836095693,
-2.14724346758807));
#53574=CARTESIAN_POINT('Ctrl Pts',(-7.60456873015009,1.88624821092527,-1.03714300367325));
#53575=CARTESIAN_POINT('Ctrl Pts',(-7.49342238527265,1.89428068216789,1.02239846461776));
#53576=CARTESIAN_POINT('Ctrl Pts',(-7.38227604039525,0.168215013541517,
2.1459966524919));
#53577=CARTESIAN_POINT('Ctrl Pts',(-7.2711296955178,-1.71184121457602,1.30506612068739));
#53578=CARTESIAN_POINT('Ctrl Pts',(-7.15998335064039,-2.02481148025317,
-0.730572647121488));
#53579=CARTESIAN_POINT('Ctrl Pts',(-7.04883700576296,-0.484190641641625,
-2.09741682691683));
#53580=CARTESIAN_POINT('Ctrl Pts',(-6.93769066088555,1.49967712384657,-1.54420414696323));
#53581=CARTESIAN_POINT('Ctrl Pts',(-6.82654431600811,2.11068217931116,0.422633010099142));
#53582=CARTESIAN_POINT('Ctrl Pts',(-6.7153979711307,0.789486756011834,2.0025754880576));
#53583=CARTESIAN_POINT('Ctrl Pts',(-6.60425162625327,-1.25443551972232,
1.74928255297597));
#53584=CARTESIAN_POINT('Ctrl Pts',(-6.49310528137585,-2.14999877885788,
-0.105371600522998));
#53585=CARTESIAN_POINT('Ctrl Pts',(-6.38195893649842,-1.07736961633439,
-1.86356449662648));
#53586=CARTESIAN_POINT('Ctrl Pts',(-6.270812591621,0.98152555482447,-1.9157780426014));
#53587=CARTESIAN_POINT('Ctrl Pts',(-6.15966624674358,2.14189409533265,-0.214213929673716));
#53588=CARTESIAN_POINT('Ctrl Pts',(-6.04851990186615,1.34148955639313,1.68344993788808));
#53589=CARTESIAN_POINT('Ctrl Pts',(-5.93737355698873,-0.686966646850282,
2.0400183208497));
#53590=CARTESIAN_POINT('Ctrl Pts',(-5.82622721211131,-2.08654688906569,
0.529074666769661));
#53591=CARTESIAN_POINT('Ctrl Pts',(-5.71508086723388,-1.57602103499908,
-1.46620449478496));
#53592=CARTESIAN_POINT('Ctrl Pts',(-5.60393452235647,0.37725571174863,-2.11926309155805));
#53593=CARTESIAN_POINT('Ctrl Pts',(-5.49278817747903,1.9851779214646,-0.832265909079935));
#53594=CARTESIAN_POINT('Ctrl Pts',(-5.38164183260162,1.77579112659265,1.21661982476122));
#53595=CARTESIAN_POINT('Ctrl Pts',(-5.27049548772418,-0.0592238649919277,
2.15176449852268));
#53596=CARTESIAN_POINT('Ctrl Pts',(-5.15934914284677,-1.84002302938406,
1.11710034223584));
#53597=CARTESIAN_POINT('Ctrl Pts',(-5.04820279796934,-1.93639361747923,
-0.940200872937754));
#53598=CARTESIAN_POINT('Ctrl Pts',(-4.93705645309191,-0.260114248398049,
-2.13680567695508));
#53599=CARTESIAN_POINT('Ctrl Pts',(-4.8259101082145,1.65428381056188,-1.37729553742109));
#53600=CARTESIAN_POINT('Ctrl Pts',(-4.71476376333707,2.05428619114345,0.643044452712678));
#53601=CARTESIAN_POINT('Ctrl Pts',(-4.60361741845965,0.573715171829774,
2.07471656495518));
#53602=CARTESIAN_POINT('Ctrl Pts',(-4.49247107358222,-1.43205700782412,
1.60711251928082));
#53603=CARTESIAN_POINT('Ctrl Pts',(-4.3813247287048,-2.12686855908149,-0.331704771864523));
#53604=CARTESIAN_POINT('Ctrl Pts',(-4.27017838382738,-0.874661990601799,
-1.96686662625693));
#53605=CARTESIAN_POINT('Ctrl Pts',(-4.15903203894995,1.17824414959146,-1.80148234719126));
#53606=CARTESIAN_POINT('Ctrl Pts',(-4.04788569407253,2.15253981386485,0.0130488701715242));
#53607=CARTESIAN_POINT('Ctrl Pts',(-3.9367393491951,1.15631689430128,1.8156346447562));
#53608=CARTESIAN_POINT('Ctrl Pts',(-3.82559300431768,-0.89844343969415,
1.95611791796024));
#53609=CARTESIAN_POINT('Ctrl Pts',(-3.71444665944026,-2.13073373943129,
0.305894842923001));
#53610=CARTESIAN_POINT('Ctrl Pts',(-3.60330031456283,-1.41246758316153,
-1.62435625704392));
#53611=CARTESIAN_POINT('Ctrl Pts',(-3.49215396968542,0.59882628102188,-2.06760852399429));
#53612=CARTESIAN_POINT('Ctrl Pts',(-3.38100762480798,2.06193129978027,-0.618091609875463));
#53613=CARTESIAN_POINT('Ctrl Pts',(-3.26986127993057,1.63746428918603,1.39725038017704));
#53614=CARTESIAN_POINT('Ctrl Pts',(-3.15871493505314,-0.286001156470349,
2.13349508134046));
#53615=CARTESIAN_POINT('Ctrl Pts',(-3.04756859017572,-1.94765003058781,
0.916655486572005));
#53616=CARTESIAN_POINT('Ctrl Pts',(-2.93642224529829,-1.8263443898979,-1.13932615734432));
#53617=CARTESIAN_POINT('Ctrl Pts',(-2.82527590042087,-0.0331321304115914,
-2.15232436849944));
#53618=CARTESIAN_POINT('Ctrl Pts',(-2.71412955554345,1.79041056752518,-1.19500122121443));
#53619=CARTESIAN_POINT('Ctrl Pts',(-2.60298321066602,1.97494186655942,0.856272473300212));
#53620=CARTESIAN_POINT('Ctrl Pts',(-2.4918368657886,0.351534639424466,2.12368108078498));
#53621=CARTESIAN_POINT('Ctrl Pts',(-2.38069052091118,-1.59368104817839,
1.44698949858494));
#53622=CARTESIAN_POINT('Ctrl Pts',(-2.26954417603376,-2.07997919520774,
-0.55433247252024));
#53623=CARTESIAN_POINT('Ctrl Pts',(-2.15839783115633,-0.662183540785041,
-2.04819700072118));
#53624=CARTESIAN_POINT('Ctrl Pts',(-2.0472514862789,1.36180060444583,-1.66706233186268));
#53625=CARTESIAN_POINT('Ctrl Pts',(-1.93610514140148,2.13913966163297,0.240165820636954));
#53626=CARTESIAN_POINT('Ctrl Pts',(-1.82495879652405,0.958226966987404,
1.92753713380078));
#53627=CARTESIAN_POINT('Ctrl Pts',(-1.71381245164664,-1.09988356808257,
1.85036551760173));
#53628=CARTESIAN_POINT('Ctrl Pts',(-1.60266610676921,-2.15111862857713,
0.0792984394831497));
#53629=CARTESIAN_POINT('Ctrl Pts',(-1.49151976189179,-1.23313481946782,
-1.76436347045422));
#53630=CARTESIAN_POINT('Ctrl Pts',(-1.38037341701436,0.813706056197659,
-1.9928547775867));
#53631=CARTESIAN_POINT('Ctrl Pts',(-1.26922707213695,2.11565347288727,-0.397016476196565));
#53632=CARTESIAN_POINT('Ctrl Pts',(-1.15808072725951,1.48084058983645,1.562279617094));
#53633=CARTESIAN_POINT('Ctrl Pts',(-1.04693438238209,-0.509574368188878,
2.0913785983932));
#53634=CARTESIAN_POINT('Ctrl Pts',(-0.935788037504666,-2.03353737199865,
0.705997133765736));
#53635=CARTESIAN_POINT('Ctrl Pts',(-0.824641692627246,-1.69585995945638,
-1.32577433553849));
#53636=CARTESIAN_POINT('Ctrl Pts',(-0.71349534774982,0.194156965638061,
-2.14370394685488));
#53637=CARTESIAN_POINT('Ctrl Pts',(-0.602349002872396,1.90665684596558,
-0.999539474359144));
#53638=CARTESIAN_POINT('Ctrl Pts',(-0.491202657994974,1.87330694072299,
1.06028137806503));
#53639=CARTESIAN_POINT('Ctrl Pts',(-0.38005631311755,0.125863161526222,
2.14826070212494));
#53640=CARTESIAN_POINT('Ctrl Pts',(-0.268909968240128,-1.7383416148007,
1.27198342040961));
#53641=CARTESIAN_POINT('Ctrl Pts',(-0.157763623362701,-2.00817094135109,
-0.773402904505074));
#53642=CARTESIAN_POINT('Ctrl Pts',(-0.0836660601110885,-0.966914112917088,
-1.65786295142018));
#53643=CARTESIAN_POINT('Ctrl Pts',(-0.0466172784852814,-0.374209849651548,
-1.78230609497963));
#53644=CARTESIAN_POINT('Ctrl Pts',(-29.646,-0.861525859670322,1.75382131162764));
#53645=CARTESIAN_POINT('Ctrl Pts',(-29.6089512183742,-1.44475753426074,
1.46732167423177));
#53646=CARTESIAN_POINT('Ctrl Pts',(-29.5348536551226,-2.29286652888411,
0.271744870419408));
#53647=CARTESIAN_POINT('Ctrl Pts',(-29.4237073102451,-1.47012297763525,
-1.78326461171051));
#53648=CARTESIAN_POINT('Ctrl Pts',(-29.3125609653677,0.700336273471097,
-2.2001292463347));
#53649=CARTESIAN_POINT('Ctrl Pts',(-29.2014146204903,2.22869993715502,-0.605756315417338));
#53650=CARTESIAN_POINT('Ctrl Pts',(-29.0902682756129,1.71733799299121,1.54462975010717));
#53651=CARTESIAN_POINT('Ctrl Pts',(-28.9791219307354,-0.366411226603099,
2.2802253866561));
#53652=CARTESIAN_POINT('Ctrl Pts',(-28.8679755858581,-2.11459180492753,
0.928822024838786));
#53653=CARTESIAN_POINT('Ctrl Pts',(-28.7568292409806,-1.92706730220025,
-1.27307553550754));
#53654=CARTESIAN_POINT('Ctrl Pts',(-28.6456828961032,0.0246086105193235,
-2.30943755856561));
#53655=CARTESIAN_POINT('Ctrl Pts',(-28.5345365512257,1.95373627660718,-1.23170996805708));
#53656=CARTESIAN_POINT('Ctrl Pts',(-28.4233902063484,2.09434865472725,0.973603941376282));
#53657=CARTESIAN_POINT('Ctrl Pts',(-28.3122438614709,0.317707212387436,
2.28762659388261));
#53658=CARTESIAN_POINT('Ctrl Pts',(-28.2010975165935,-1.74977276828138,
1.50747558605084));
#53659=CARTESIAN_POINT('Ctrl Pts',(-28.0899511717161,-2.21544433956327,
-0.652681674006207));
#53660=CARTESIAN_POINT('Ctrl Pts',(-27.9788048268387,-0.653011253992698,
-2.21534638945854));
#53661=CARTESIAN_POINT('Ctrl Pts',(-27.8676584819612,1.50721327238238,-1.74999819254223));
#53662=CARTESIAN_POINT('Ctrl Pts',(-27.7565121370838,2.28767643383428,0.317367004816054));
#53663=CARTESIAN_POINT('Ctrl Pts',(-27.6453657922064,0.973911578695988,
2.09420176868224));
#53664=CARTESIAN_POINT('Ctrl Pts',(-27.534219447329,-1.23140971440338,1.95392304382396));
#53665=CARTESIAN_POINT('Ctrl Pts',(-27.4230731024515,-2.3094507409455,0.0249471482242496));
#53666=CARTESIAN_POINT('Ctrl Pts',(-27.3119267575742,-1.27333080669325,
-1.92686628595169));
#53667=CARTESIAN_POINT('Ctrl Pts',(-27.2007804126966,0.928445614870621,
-2.1147514788365));
#53668=CARTESIAN_POINT('Ctrl Pts',(-27.0896340678193,2.28028685009023,-0.366710984170037));
#53669=CARTESIAN_POINT('Ctrl Pts',(-26.9784877229418,1.54466489828968,1.71703098688042));
#53670=CARTESIAN_POINT('Ctrl Pts',(-26.8673413780645,-0.605003318954584,
2.22893608010939));
#53671=CARTESIAN_POINT('Ctrl Pts',(-26.756195033187,-2.20082799096117,0.70038647693972));
#53672=CARTESIAN_POINT('Ctrl Pts',(-26.6450486883096,-1.78192920518164,
-1.46932412009659));
#53673=CARTESIAN_POINT('Ctrl Pts',(-26.5339023434321,0.268216812756021,
-2.29395832668387));
#53674=CARTESIAN_POINT('Ctrl Pts',(-26.4227559985547,2.07282673867339,-1.01861394760441));
#53675=CARTESIAN_POINT('Ctrl Pts',(-26.3116096536773,1.97989052702902,1.18920921781411));
#53676=CARTESIAN_POINT('Ctrl Pts',(-26.2004633087999,0.0744855971360473,
2.30838405788893));
#53677=CARTESIAN_POINT('Ctrl Pts',(-26.0893169639225,-1.89910634257262,
1.31437443768203));
#53678=CARTESIAN_POINT('Ctrl Pts',(-25.978170619045,-2.13418254536613,-0.882864613564002));
#53679=CARTESIAN_POINT('Ctrl Pts',(-25.8670242741676,-0.41554512119227,
-2.27189509333105));
#53680=CARTESIAN_POINT('Ctrl Pts',(-25.7558779292902,1.68349845317816,-1.58114452880967));
#53681=CARTESIAN_POINT('Ctrl Pts',(-25.6447315844128,2.24140213016567,0.557047173700168));
#53682=CARTESIAN_POINT('Ctrl Pts',(-25.5335852395353,0.747439206175521,
2.18529624900443));
#53683=CARTESIAN_POINT('Ctrl Pts',(-25.4224388946579,-1.43075860934684,
1.8130402269722));
#53684=CARTESIAN_POINT('Ctrl Pts',(-25.3112925497805,-2.29918440088871,
-0.218943265595743));
#53685=CARTESIAN_POINT('Ctrl Pts',(-25.2001462049031,-1.06284745566775,
-2.05049758566565));
#53686=CARTESIAN_POINT('Ctrl Pts',(-25.0889998600256,1.14646134804713,-2.00494674250309));
#53687=CARTESIAN_POINT('Ctrl Pts',(-24.9778535151482,2.30625488731607,-0.12398974784463));
#53688=CARTESIAN_POINT('Ctrl Pts',(-24.8667071702708,1.3548130918185,1.87047227968689));
#53689=CARTESIAN_POINT('Ctrl Pts',(-24.7555608253934,-0.8368772500053,2.15263130407031));
#53690=CARTESIAN_POINT('Ctrl Pts',(-24.6444144805159,-2.26245763980657,
0.464187990926873));
#53691=CARTESIAN_POINT('Ctrl Pts',(-24.5332681356385,-1.61689639697985,
-1.64919104541392));
#53692=CARTESIAN_POINT('Ctrl Pts',(-24.4221217907611,0.508834633121875,
-2.25283651847523));
#53693=CARTESIAN_POINT('Ctrl Pts',(-24.3109754458837,2.16875866898886,-0.794147907209686));
#53694=CARTESIAN_POINT('Ctrl Pts',(-24.1998291010062,1.84331675084411,1.39153455540902));
#53695=CARTESIAN_POINT('Ctrl Pts',(-24.0886827561289,-0.169568944201683,
2.30335221709625));
#53696=CARTESIAN_POINT('Ctrl Pts',(-23.9775364112514,-2.02722463902219,
1.10659176112116));
#53697=CARTESIAN_POINT('Ctrl Pts',(-23.866390066374,-2.02908013025209,-1.10318579027107));
#53698=CARTESIAN_POINT('Ctrl Pts',(-23.7552437214965,-0.173436829123328,
-2.30306420430337));
#53699=CARTESIAN_POINT('Ctrl Pts',(-23.6440973766192,1.84097728437699,-1.39462815877487));
#53700=CARTESIAN_POINT('Ctrl Pts',(-23.5329510317417,2.17008925948164,0.790504692410032));
#53701=CARTESIAN_POINT('Ctrl Pts',(-23.4218046868643,0.512617206336567,
2.25197883262866));
#53702=CARTESIAN_POINT('Ctrl Pts',(-23.3106583419869,-1.61412455553813,
1.65190404747029));
#53703=CARTESIAN_POINT('Ctrl Pts',(-23.1995119971095,-2.26323398149513,
-0.460387888465295));
#53704=CARTESIAN_POINT('Ctrl Pts',(-23.088365652232,-0.840491081477214,
-2.15122286265211));
#53705=CARTESIAN_POINT('Ctrl Pts',(-22.9772193073546,1.35167001231022,-1.87274484131212));
#53706=CARTESIAN_POINT('Ctrl Pts',(-22.8660729624772,2.30645985687955,0.120116574389448));
#53707=CARTESIAN_POINT('Ctrl Pts',(-22.7549266175997,1.14982672957971,2.00301861069334));
#53708=CARTESIAN_POINT('Ctrl Pts',(-22.6437802727223,-1.05940246318485,
2.05227958227862));
#53709=CARTESIAN_POINT('Ctrl Pts',(-22.5326339278449,-2.29881347743167,
0.222804081691522));
#53710=CARTESIAN_POINT('Ctrl Pts',(-22.4214875829675,-1.43380131266057,
-1.81063493246228));
#53711=CARTESIAN_POINT('Ctrl Pts',(-22.3103412380901,0.743768284930297,
-2.18654837613342));
#53712=CARTESIAN_POINT('Ctrl Pts',(-22.1991948932126,2.240463494933,-0.560810476642942));
#53713=CARTESIAN_POINT('Ctrl Pts',(-22.0880485483352,1.68615136712066,1.57831512379404));
#53714=CARTESIAN_POINT('Ctrl Pts',(-21.9769022034578,-0.411729238576987,
2.27258973352884));
#53715=CARTESIAN_POINT('Ctrl Pts',(-21.8657558585804,-2.13269690129466,
0.886447398353686));
#53716=CARTESIAN_POINT('Ctrl Pts',(-21.7546095137029,-1.90131095334948,
-1.31118332871995));
#53717=CARTESIAN_POINT('Ctrl Pts',(-21.6434631688255,0.070608917869684,
-2.30850588986841));
#53718=CARTESIAN_POINT('Ctrl Pts',(-21.5323168239481,1.97789064211908,-1.19253246104986));
#53719=CARTESIAN_POINT('Ctrl Pts',(-21.4211704790707,2.07453442044502,1.01513151917801));
#53720=CARTESIAN_POINT('Ctrl Pts',(-21.3100241341932,0.272068783015987,
2.29350466320609));
#53721=CARTESIAN_POINT('Ctrl Pts',(-21.1988777893159,-1.77945918978171,
1.47231452303552));
#53722=CARTESIAN_POINT('Ctrl Pts',(-21.0877314444384,-2.20200107829871,
-0.69668953918594));
#53723=CARTESIAN_POINT('Ctrl Pts',(-20.976585099561,-0.608745619668004,
-2.22791692694654));
#53724=CARTESIAN_POINT('Ctrl Pts',(-20.8654387546836,1.54177923238312,-1.71962259273132));
#53725=CARTESIAN_POINT('Ctrl Pts',(-20.7542924098061,2.28089946835357,0.362881079837752));
#53726=CARTESIAN_POINT('Ctrl Pts',(-20.6431460649287,0.931995705275805,
2.11318931196126));
#53727=CARTESIAN_POINT('Ctrl Pts',(-20.5319997200513,-1.27009313966377,
1.92900193867681));
#53728=CARTESIAN_POINT('Ctrl Pts',(-20.4208533751739,-2.30948937432413,
-0.0210687618001371));
#53729=CARTESIAN_POINT('Ctrl Pts',(-20.3097070302964,-1.23468929913284,
-1.95185229908585));
#53730=CARTESIAN_POINT('Ctrl Pts',(-20.198560685419,0.970393335078177,-2.09583440139618));
#53731=CARTESIAN_POINT('Ctrl Pts',(-20.0874143405416,2.28714020514337,-0.32120825776529));
#53732=CARTESIAN_POINT('Ctrl Pts',(-19.9762679956642,1.51015006321536,1.74746440576353));
#53733=CARTESIAN_POINT('Ctrl Pts',(-19.8651216507867,-0.649290124366777,
2.21644025347845));
#53734=CARTESIAN_POINT('Ctrl Pts',(-19.7539753059093,-2.21434490354622,
0.65640057204329));
#53735=CARTESIAN_POINT('Ctrl Pts',(-19.6428289610319,-1.75230231831962,
-1.50453369787837));
#53736=CARTESIAN_POINT('Ctrl Pts',(-19.5316826161545,0.313865895854717,
-2.28815936120261));
#53737=CARTESIAN_POINT('Ctrl Pts',(-19.420536271277,2.09270907351595,-0.97711503747712));
#53738=CARTESIAN_POINT('Ctrl Pts',(-19.3093899263996,1.95580505181399,1.22841835794599));
#53739=CARTESIAN_POINT('Ctrl Pts',(-19.1982435815222,0.028481091702752,
2.30940985757298));
#53740=CARTESIAN_POINT('Ctrl Pts',(-19.0870972366448,-1.9249155664031,1.27627784007202));
#53741=CARTESIAN_POINT('Ctrl Pts',(-18.9759508917673,-2.11616972127427,
-0.925208502772121));
#53742=CARTESIAN_POINT('Ctrl Pts',(-18.8648045468899,-0.370199888246757,
-2.27972303264715));
#53743=CARTESIAN_POINT('Ctrl Pts',(-18.7536582020125,1.71466530682062,-1.54729051843073));
#53744=CARTESIAN_POINT('Ctrl Pts',(-18.6425118571351,2.22985925567511,0.601591857258662));
#53745=CARTESIAN_POINT('Ctrl Pts',(-18.5313655122576,0.7037533993653,2.1997536716009));
#53746=CARTESIAN_POINT('Ctrl Pts',(-18.4202191673802,-1.46659566348409,
1.78417550221091));
#53747=CARTESIAN_POINT('Ctrl Pts',(-18.3090728225028,-2.29436607052567,
-0.264706247112593));
#53748=CARTESIAN_POINT('Ctrl Pts',(-18.1979264776254,-1.02178462763778,
-2.07126561250917));
#53749=CARTESIAN_POINT('Ctrl Pts',(-18.086780132748,1.18617816544452,-1.98170795594672));
#53750=CARTESIAN_POINT('Ctrl Pts',(-17.9756337878705,2.30826737621457,-0.0780178360589921));
#53751=CARTESIAN_POINT('Ctrl Pts',(-17.8644874429931,1.31727894168396,1.89709284238697));
#53752=CARTESIAN_POINT('Ctrl Pts',(-17.7533410981157,-0.879597819727813,
2.13553102023126));
#53753=CARTESIAN_POINT('Ctrl Pts',(-17.6421947532383,-2.27125655965968,
0.419021124816741));
#53754=CARTESIAN_POINT('Ctrl Pts',(-17.5310484083608,-1.58371879384272,
-1.68107698957223));
#53755=CARTESIAN_POINT('Ctrl Pts',(-17.4199020634834,0.553616692201852,
-2.24225190845172));
#53756=CARTESIAN_POINT('Ctrl Pts',(-17.308755718606,2.18414994709609,-0.75078230629124));
#53757=CARTESIAN_POINT('Ctrl Pts',(-17.1976093737286,1.8152274739619,1.42798259114521));
#53758=CARTESIAN_POINT('Ctrl Pts',(-17.0864630288511,-0.215424760589663,
2.29951673952697));
#53759=CARTESIAN_POINT('Ctrl Pts',(-16.9753166839737,-2.0488687988391,1.06598391544312));
#53760=CARTESIAN_POINT('Ctrl Pts',(-16.8641703390963,-2.00669872860475,
-1.14339200428198));
#53761=CARTESIAN_POINT('Ctrl Pts',(-16.7530239942189,-0.127518670722472,
-2.306062456105));
#53762=CARTESIAN_POINT('Ctrl Pts',(-16.6418776493414,1.8683969331536,-1.35767373216913));
#53763=CARTESIAN_POINT('Ctrl Pts',(-16.530731304464,2.15390938673701,0.833582279421827));
#53764=CARTESIAN_POINT('Ctrl Pts',(-16.4195849595866,0.467649496259791,
2.26174468309042));
#53765=CARTESIAN_POINT('Ctrl Pts',(-16.3084386147092,-1.6467149138954,1.61941812241135));
#53766=CARTESIAN_POINT('Ctrl Pts',(-16.1972922698318,-2.25361250777475,
-0.505386710985868));
#53767=CARTESIAN_POINT('Ctrl Pts',(-16.0861459249543,-0.797465646570921,
-2.16754091204274));
#53768=CARTESIAN_POINT('Ctrl Pts',(-15.9749995800769,1.38871225351008,-1.84544394111303));
#53769=CARTESIAN_POINT('Ctrl Pts',(-15.8638532351995,2.30360899748014,0.166044119343147));
#53770=CARTESIAN_POINT('Ctrl Pts',(-15.7527068903221,1.1096925570471,2.02552894120872));
#53771=CARTESIAN_POINT('Ctrl Pts',(-15.6415605454446,-1.10007956787695,
2.03076586714951));
#53772=CARTESIAN_POINT('Ctrl Pts',(-15.5304142005672,-2.30279611211481,
0.17696081167541));
#53773=CARTESIAN_POINT('Ctrl Pts',(-15.4192678556898,-1.39744361879813,
-1.83884104672487));
#53774=CARTESIAN_POINT('Ctrl Pts',(-15.3081215108124,0.787183061676606,
-2.17129636168103));
#53775=CARTESIAN_POINT('Ctrl Pts',(-15.1969751659349,2.25119178102243,-0.516062620131469));
#53776=CARTESIAN_POINT('Ctrl Pts',(-15.0858288210575,1.65437207261294,1.61159489580918));
#53777=CARTESIAN_POINT('Ctrl Pts',(-14.9746824761801,-0.45692411268592,
2.26393582463948));
#53778=CARTESIAN_POINT('Ctrl Pts',(-14.8635361313027,-2.14993421117156,
0.843781933009972));
#53779=CARTESIAN_POINT('Ctrl Pts',(-14.7523897864253,-1.87481099576699,
-1.34880272575014));
#53780=CARTESIAN_POINT('Ctrl Pts',(-14.6412434415478,0.116587052068778,
-2.30664096081938));
#53781=CARTESIAN_POINT('Ctrl Pts',(-14.5300970966704,2.00125678238095,-1.15289043443605));
#53782=CARTESIAN_POINT('Ctrl Pts',(-14.418950751793,2.05389829406855,1.05626079187961));
#53783=CARTESIAN_POINT('Ctrl Pts',(-14.3078044069156,0.226321501915263,
2.29846984766184));
#53784=CARTESIAN_POINT('Ctrl Pts',(-14.1966580620381,-1.80843878694902,
1.43657029646943));
#53785=CARTESIAN_POINT('Ctrl Pts',(-14.0855117171607,-2.18768394226603,
-0.740421522911927));
#53786=CARTESIAN_POINT('Ctrl Pts',(-13.9743653722833,-0.564238213060542,
-2.23960271069716));
#53787=CARTESIAN_POINT('Ctrl Pts',(-13.8632190274059,1.57573310019489,-1.68856455600315));
#53788=CARTESIAN_POINT('Ctrl Pts',(-13.7520726825284,2.27321710747686,0.408251203445124));
#53789=CARTESIAN_POINT('Ctrl Pts',(-13.640926337651,0.889709847359887,2.13133794841426));
#53790=CARTESIAN_POINT('Ctrl Pts',(-13.5297799927736,-1.30827237724028,
1.90331512099021));
#53791=CARTESIAN_POINT('Ctrl Pts',(-13.4186336478962,-2.3086112340065,-0.067076322639307));
#53792=CARTESIAN_POINT('Ctrl Pts',(-13.3074873030187,-1.19555766468852,
-1.97606349423402));
#53793=CARTESIAN_POINT('Ctrl Pts',(-13.1963409581413,1.01195584499574,-2.07608536207423));
#53794=CARTESIAN_POINT('Ctrl Pts',(-13.0851946132639,2.29308565401936,-0.275578021929272));
#53795=CARTESIAN_POINT('Ctrl Pts',(-12.9740482683865,1.47503575613473,1.7772041472391));
#53796=CARTESIAN_POINT('Ctrl Pts',(-12.862901923509,-0.693319186314957,
2.20306458569137));
#53797=CARTESIAN_POINT('Ctrl Pts',(-12.7517555786316,-2.22698280627896,
0.612154101005415));
#53798=CARTESIAN_POINT('Ctrl Pts',(-12.6406092337542,-1.72197983462208,
-1.53914603335576));
#53799=CARTESIAN_POINT('Ctrl Pts',(-12.5294628888768,0.359390386207514,
-2.28145208434048));
#53800=CARTESIAN_POINT('Ctrl Pts',(-12.4183165439994,2.11176068317365,-0.935228250130298));
#53801=CARTESIAN_POINT('Ctrl Pts',(-12.3071701991219,1.93094319703423,1.26713986310393));
#53802=CARTESIAN_POINT('Ctrl Pts',(-12.1960238542445,-0.0175347196268082,
2.30951891017318));
#53803=CARTESIAN_POINT('Ctrl Pts',(-12.0848775093671,-1.94996067261942,
1.23767460912692));
#53804=CARTESIAN_POINT('Ctrl Pts',(-11.9737311644897,-2.0973168590043,-0.967185119703648));
#53805=CARTESIAN_POINT('Ctrl Pts',(-11.8625848196123,-0.324707700151707,
-2.28664600939937));
#53806=CARTESIAN_POINT('Ctrl Pts',(-11.7514384747348,1.74515150413228,-1.51282229308821));
#53807=CARTESIAN_POINT('Ctrl Pts',(-11.6402921298574,2.21743121262479,0.645897731933769));
#53808=CARTESIAN_POINT('Ctrl Pts',(-11.52914578498,0.659788229460352,2.21333787639969));
#53809=CARTESIAN_POINT('Ctrl Pts',(-11.4179994401025,-1.50185053541965,
1.75460252823812));
#53810=CARTESIAN_POINT('Ctrl Pts',(-11.3068530952251,-2.28863696487281,
-0.31036415040662));
#53811=CARTESIAN_POINT('Ctrl Pts',(-11.1957067503477,-0.980316190318959,
-2.09121142638385));
#53812=CARTESIAN_POINT('Ctrl Pts',(-11.0845604054703,1.22542411562664,-1.95768250737462));
#53813=CARTESIAN_POINT('Ctrl Pts',(-10.9734140605928,2.30936357153834,-0.0320149541862179));
#53814=CARTESIAN_POINT('Ctrl Pts',(-10.8622677157154,1.27922188235666,1.92296033202449));
#53815=CARTESIAN_POINT('Ctrl Pts',(-10.751121370838,-0.921969222868076,
2.11758301252251));
#53816=CARTESIAN_POINT('Ctrl Pts',(-10.6399750259606,-2.27915387781204,
0.37368792339892));
#53817=CARTESIAN_POINT('Ctrl Pts',(-10.5288286810831,-1.54991251511545,
-1.71229561067251));
#53818=CARTESIAN_POINT('Ctrl Pts',(-10.4176823362058,0.598178986698543,
-2.23077721046101));
#53819=CARTESIAN_POINT('Ctrl Pts',(-10.3065359913283,2.19867420148525,-0.707118673606509));
#53820=CARTESIAN_POINT('Ctrl Pts',(-10.1953896464509,1.78641762142706,1.4638637725877));
#53821=CARTESIAN_POINT('Ctrl Pts',(-10.0842433015735,-0.261195061613987,
2.29476844204995));
#53822=CARTESIAN_POINT('Ctrl Pts',(-9.97309695669604,-2.06969963636276,
1.02495291505498));
#53823=CARTESIAN_POINT('Ctrl Pts',(-9.86195061181862,-1.98352074456387,
-1.18314433554179));
#53824=CARTESIAN_POINT('Ctrl Pts',(-9.7508042669412,-0.0815498923025786,
-2.30814528960058));
#53825=CARTESIAN_POINT('Ctrl Pts',(-9.63965792206376,1.8950749000425,-1.32018036118887));
#53826=CARTESIAN_POINT('Ctrl Pts',(-9.52851157718637,2.13687449461638,0.876328966255154));
#53827=CARTESIAN_POINT('Ctrl Pts',(-9.41736523230891,0.422496147277826,
2.27061270770145));
#53828=CARTESIAN_POINT('Ctrl Pts',(-9.30621888743152,-1.67865158962016,
1.58628935049869));
#53829=CARTESIAN_POINT('Ctrl Pts',(-9.19507254255407,-2.24309643636514,
-0.55018491437503));
#53830=CARTESIAN_POINT('Ctrl Pts',(-9.08392619767667,-0.754123648403588,
-2.18299853086491));
#53831=CARTESIAN_POINT('Ctrl Pts',(-8.97277985279923,1.42520322923344,-1.81741047048332));
#53832=CARTESIAN_POINT('Ctrl Pts',(-8.86163350792181,2.29984369370358,0.211905751152958));
#53833=CARTESIAN_POINT('Ctrl Pts',(-8.75048716304439,1.06911787915085,2.04723521445874));
#53834=CARTESIAN_POINT('Ctrl Pts',(-8.63934081816696,-1.14031998319325,
2.00844601589637));
#53835=CARTESIAN_POINT('Ctrl Pts',(-8.52819447328954,-2.3058646251051,0.131047295007472));
#53836=CARTESIAN_POINT('Ctrl Pts',(-8.41704812841211,-1.36053119344223,
-1.86631721165256));
#53837=CARTESIAN_POINT('Ctrl Pts',(-8.3059017835347,0.830285356953508,-2.15518242589077));
#53838=CARTESIAN_POINT('Ctrl Pts',(-8.19475543865726,2.26102643035827,-0.471109906562324));
#53839=CARTESIAN_POINT('Ctrl Pts',(-8.08360909377985,1.62193605587453,1.64423492649137));
#53840=CARTESIAN_POINT('Ctrl Pts',(-7.97246274890242,-0.50193760545539,
2.25438322010025));
#53841=CARTESIAN_POINT('Ctrl Pts',(-7.861316404025,-2.1663180796646,0.800781518616722));
#53842=CARTESIAN_POINT('Ctrl Pts',(-7.75017005914758,-1.84756681016008,
-1.38588669985493));
#53843=CARTESIAN_POINT('Ctrl Pts',(-7.63902371427016,0.162518905681942,
-2.30386038382012));
#53844=CARTESIAN_POINT('Ctrl Pts',(-7.52787736939272,2.02382850049311,-1.11279075455885));
#53845=CARTESIAN_POINT('Ctrl Pts',(-7.41673102451531,2.03244684888222,1.09697076957804));
#53846=CARTESIAN_POINT('Ctrl Pts',(-7.30558467963787,0.18048437986273,2.30252262778576));
#53847=CARTESIAN_POINT('Ctrl Pts',(-7.19443833476047,-1.83670050331195,
1.40025580662016));
#53848=CARTESIAN_POINT('Ctrl Pts',(-7.08329198988302,-2.1724983796548,-0.783859587705042));
#53849=CARTESIAN_POINT('Ctrl Pts',(-6.97214564500562,-0.519506825533608,
-2.25039945811047));
#53850=CARTESIAN_POINT('Ctrl Pts',(-6.86099930012817,1.60906146243046,-1.65683622394037));
#53851=CARTESIAN_POINT('Ctrl Pts',(-6.74985295525077,2.26463236663712,0.453459266990303));
#53852=CARTESIAN_POINT('Ctrl Pts',(-6.63870661037333,0.847070808774789,
2.14864052548618));
#53853=CARTESIAN_POINT('Ctrl Pts',(-6.52756026549592,-1.34593228088452,
1.87687276023519));
#53854=CARTESIAN_POINT('Ctrl Pts',(-6.41641392061849,-2.30681666361579,
-0.113057256752296));
#53855=CARTESIAN_POINT('Ctrl Pts',(-6.30526757574106,-1.15595143972763,
-1.9994902680012));
#53856=CARTESIAN_POINT('Ctrl Pts',(-6.19412123086365,1.05311664727397,-2.05551219652773));
#53857=CARTESIAN_POINT('Ctrl Pts',(-6.08297488598622,2.29812083588177,-0.229838392193094));
#53858=CARTESIAN_POINT('Ctrl Pts',(-5.97182854110879,1.43933591645946,1.80623840686375));
#53859=CARTESIAN_POINT('Ctrl Pts',(-5.86068219623138,-0.737073027150487,
2.18881438580046));
#53860=CARTESIAN_POINT('Ctrl Pts',(-5.74953585135395,-2.23873668229215,
0.5676646282792));
#53861=CARTESIAN_POINT('Ctrl Pts',(-5.63838950647653,-1.69097379100657,
-1.57314738691859));
#53862=CARTESIAN_POINT('Ctrl Pts',(-5.5272431615991,0.404772212367679,-2.27383915854548));
#53863=CARTESIAN_POINT('Ctrl Pts',(-5.41609681672169,2.12997400487336,-0.892970213055048));
#53864=CARTESIAN_POINT('Ctrl Pts',(-5.30495047184425,1.90531483190004,1.3053583623594));
#53865=CARTESIAN_POINT('Ctrl Pts',(-5.19380412696684,-0.0635435703455707,
2.30871117238765));
#53866=CARTESIAN_POINT('Ctrl Pts',(-5.0826577820894,-1.97423171927328,1.19858006885444));
#53867=CARTESIAN_POINT('Ctrl Pts',(-4.97151143721199,-2.07763144242026,
-1.00877780125587));
#53868=CARTESIAN_POINT('Ctrl Pts',(-4.86036509233456,-0.279086615559442,
-2.2926612754298));
#53869=CARTESIAN_POINT('Ctrl Pts',(-4.74921874745714,1.77494494326237,-1.47775353534586));
#53870=CARTESIAN_POINT('Ctrl Pts',(-4.63807240257972,2.20412293447108,0.689947209993967));
#53871=CARTESIAN_POINT('Ctrl Pts',(-4.52692605770229,0.615561148945878,
2.22604347099247));
#53872=CARTESIAN_POINT('Ctrl Pts',(-4.41577971282487,-1.53650923032218,
1.72433304438984));
#53873=CARTESIAN_POINT('Ctrl Pts',(-4.30463336794745,-2.28199935816521,
-0.355898851042403));
#53874=CARTESIAN_POINT('Ctrl Pts',(-4.19348702307002,-0.938458605089674,
-2.11032710956682));
#53875=CARTESIAN_POINT('Ctrl Pts',(-4.0823406781926,1.26418361945739,-1.93287993396815));
#53876=CARTESIAN_POINT('Ctrl Pts',(-3.97119433331517,2.3095430381396,0.0140006363953164));
#53877=CARTESIAN_POINT('Ctrl Pts',(-3.86004798843775,1.24065702102934,1.94806448019787));
#53878=CARTESIAN_POINT('Ctrl Pts',(-3.74890164356033,-0.96397463960601,
2.09879440561595));
#53879=CARTESIAN_POINT('Ctrl Pts',(-3.63775529868291,-2.28614645932942,
0.328206382211824));
#53880=CARTESIAN_POINT('Ctrl Pts',(-3.52660895380548,-1.51549098059717,
-1.74283451611452));
#53881=CARTESIAN_POINT('Ctrl Pts',(-3.41546260892806,0.642503827098123,
-2.21841697952858));
#53882=CARTESIAN_POINT('Ctrl Pts',(-3.30431626405063,2.21232566657125,-0.663174341921778));
#53883=CARTESIAN_POINT('Ctrl Pts',(-3.19316991917321,1.75689862967114,1.49916385624564));
#53884=CARTESIAN_POINT('Ctrl Pts',(-3.08202357429578,-0.306861678270252,
2.28910920963077));
#53885=CARTESIAN_POINT('Ctrl Pts',(-2.97087722941836,-2.08970888245738,
0.98351504754915));
#53886=CARTESIAN_POINT('Ctrl Pts',(-2.85973088454094,-1.95955537907592,
-1.22242700363369));
#53887=CARTESIAN_POINT('Ctrl Pts',(-2.74858453966352,-0.0355487413695248,
-2.30931187849249));
#53888=CARTESIAN_POINT('Ctrl Pts',(-2.63743819478609,1.92100059427707,-1.28216292829847));
#53889=CARTESIAN_POINT('Ctrl Pts',(-2.52629184990867,2.11899134653083,0.918727782279886));
#53890=CARTESIAN_POINT('Ctrl Pts',(-2.41514550503124,0.377175081231055,
2.27857938968823));
#53891=CARTESIAN_POINT('Ctrl Pts',(-2.30399916015382,-1.70992190069039,
1.55253087594118));
#53892=CARTESIAN_POINT('Ctrl Pts',(-2.1928528152764,-2.23168995008835,-0.594764702830417));
#53893=CARTESIAN_POINT('Ctrl Pts',(-2.08170647039897,-0.710482276211509,
-2.19758960707013));
#53894=CARTESIAN_POINT('Ctrl Pts',(-1.97056012552155,1.46112842376896,-1.78865551192071));
#53895=CARTESIAN_POINT('Ctrl Pts',(-1.85941378064413,2.29516549766495,0.257683177555444));
#53896=CARTESIAN_POINT('Ctrl Pts',(-1.7482674357667,1.02811869323325,2.06812897928806));
#53897=CARTESIAN_POINT('Ctrl Pts',(-1.63712109088928,-1.18010752742753,
1.98532857402419));
#53898=CARTESIAN_POINT('Ctrl Pts',(-1.52597474601185,-2.30801819359736,
0.0850823560446368));
#53899=CARTESIAN_POINT('Ctrl Pts',(-1.41482840113444,-1.32307793753456,
-1.89305365860764));
#53900=CARTESIAN_POINT('Ctrl Pts',(-1.303682056257,0.873056630627069,-2.13821080007561));
#53901=CARTESIAN_POINT('Ctrl Pts',(-1.19253571137959,2.2699662593695,-0.425974299160599));
#53902=CARTESIAN_POINT('Ctrl Pts',(-1.08138936650216,1.58885101814241,1.67623009342094));
#53903=CARTESIAN_POINT('Ctrl Pts',(-0.970243021624737,-0.546742005367173,
2.24392080969723));
#53904=CARTESIAN_POINT('Ctrl Pts',(-0.859096676747312,-2.18186072566234,
0.757491570995594));
#53905=CARTESIAN_POINT('Ctrl Pts',(-0.74795033186989,-1.81955359793778,
-1.42247444951531));
#53906=CARTESIAN_POINT('Ctrl Pts',(-0.636803986992465,0.208318501431441,
-2.30006269542661));
#53907=CARTESIAN_POINT('Ctrl Pts',(-0.525657642115041,2.04572571264764,
-1.07244447674439));
#53908=CARTESIAN_POINT('Ctrl Pts',(-0.414511297237619,2.00994331225735,
1.13761680941109));
#53909=CARTESIAN_POINT('Ctrl Pts',(-0.303364952360196,0.13504344337263,
2.30495181401234));
#53910=CARTESIAN_POINT('Ctrl Pts',(-0.192218607482772,-1.8651338054291,
1.36476010074876));
#53911=CARTESIAN_POINT('Ctrl Pts',(-0.0810722626053462,-2.15464410326713,
-0.829813823777627));
#53912=CARTESIAN_POINT('Ctrl Pts',(-0.00697469935373359,-1.03743946735969,
-1.77878514161715));
#53913=CARTESIAN_POINT('Ctrl Pts',(0.0300740822720735,-0.401504189376239,
-1.91230499291126));
#53914=CARTESIAN_POINT('Ctrl Pts',(-0.821869692124218,-1.95215209727744,
0.00149476428280041));
#53915=CARTESIAN_POINT('Ctrl Pts',(-0.797229905372775,-1.94905050159948,
-0.431580103628319));
#53916=CARTESIAN_POINT('Ctrl Pts',(-0.772590118621332,-1.80689620255586,
-0.8665002741731));
#53917=CARTESIAN_POINT('Ctrl Pts',(-0.747950331869889,-1.54195943599701,
-1.20541148708205));
#53918=CARTESIAN_POINT('Ctrl Pts',(-0.710901550244083,-1.14359623148139,
-1.71500386481906));
#53919=CARTESIAN_POINT('Ctrl Pts',(-0.673852768618274,-0.467638865024983,
-2.00753328012283));
#53920=CARTESIAN_POINT('Ctrl Pts',(-0.636803986992467,0.176574353405899,
-1.94919495132769));
#53921=CARTESIAN_POINT('Ctrl Pts',(-0.599755205366656,0.820787571836855,
-1.89085662253254));
#53922=CARTESIAN_POINT('Ctrl Pts',(-0.562706423740843,1.43325664224232,
-1.4816505496384));
#53923=CARTESIAN_POINT('Ctrl Pts',(-0.525657642115033,1.73352744404662,
-0.908703965498717));
#53924=CARTESIAN_POINT('Ctrl Pts',(-0.488608860489229,2.03379824585086,
-0.335757381359131));
#53925=CARTESIAN_POINT('Ctrl Pts',(-0.451560078863429,2.02187077905411,
0.400929714025867));
#53926=CARTESIAN_POINT('Ctrl Pts',(-0.414511297237625,1.703423734175,0.963829095818625));
#53927=CARTESIAN_POINT('Ctrl Pts',(-0.377462515611816,1.38497668929586,
1.52672847761145));
#53928=CARTESIAN_POINT('Ctrl Pts',(-0.340413733986006,0.760010066334254,
1.91584014581191));
#53929=CARTESIAN_POINT('Ctrl Pts',(-0.303364952360198,0.114163880053164,
1.95369736103487));
#53930=CARTESIAN_POINT('Ctrl Pts',(-0.268909968240138,-0.486466400236942,
1.98890418004745));
#53931=CARTESIAN_POINT('Ctrl Pts',(-0.234454984120076,-1.10515501358679,
1.72031777295108));
#53932=CARTESIAN_POINT('Ctrl Pts',(-0.200000000000016,-1.49578438409774,
1.26230645381953));
#53933=CARTESIAN_POINT('',(-29.646,-0.903606778650365,-1.26612599672272));
#53934=CARTESIAN_POINT('Ctrl Pts',(-29.646,-0.905547027071384,-1.26790990717737));
#53935=CARTESIAN_POINT('Ctrl Pts',(-29.646,-0.937793378787907,-1.25067033643914));
#53936=CARTESIAN_POINT('Ctrl Pts',(-29.646,-0.969330541631396,-1.23224815777297));
#53937=CARTESIAN_POINT('Ctrl Pts',(-29.646,-1.0000857755141,-1.212657994507));
#53938=CARTESIAN_POINT('Ctrl Pts',(-29.646,-1.05010530373861,-1.18079705245915));
#53939=CARTESIAN_POINT('Ctrl Pts',(-29.646,-1.09805783850725,-1.14584956138978));
#53940=CARTESIAN_POINT('Ctrl Pts',(-29.646,-1.14386498430002,-1.10813609735372));
#53941=CARTESIAN_POINT('Ctrl Pts',(-29.646,-1.17024530883727,-1.08641692224519));
#53942=CARTESIAN_POINT('Ctrl Pts',(-29.646,-1.19591382840587,-1.06377941838232));
#53943=CARTESIAN_POINT('Ctrl Pts',(-29.646,-1.22085272934429,-1.04027778754456));
#53944=CARTESIAN_POINT('Ctrl Pts',(-29.646,-1.23377538328808,-1.02809988751677));
#53945=CARTESIAN_POINT('Ctrl Pts',(-29.646,-1.24650526559313,-1.01568644027074));
#53946=CARTESIAN_POINT('Ctrl Pts',(-29.646,-1.25901907626856,-1.00306598282231));
#53947=CARTESIAN_POINT('Ctrl Pts',(-29.646,-1.30290144787354,-0.958809631344597));
#53948=CARTESIAN_POINT('Ctrl Pts',(-29.646,-1.34417543373733,-0.911969878856539));
#53949=CARTESIAN_POINT('Ctrl Pts',(-29.646,-1.38275268314532,-0.862895840586046));
#53950=CARTESIAN_POINT('Ctrl Pts',(-29.646,-1.41241940958756,-0.82515685993998));
#53951=CARTESIAN_POINT('Ctrl Pts',(-29.646,-1.44049103671116,-0.78609530729656));
#53952=CARTESIAN_POINT('Ctrl Pts',(-29.646,-1.46691729796725,-0.74585166902644));
#53953=CARTESIAN_POINT('Ctrl Pts',(-29.646,-1.47995477603729,-0.725997345090078));
#53954=CARTESIAN_POINT('Ctrl Pts',(-29.646,-1.49259162401709,-0.705855084298863));
#53955=CARTESIAN_POINT('Ctrl Pts',(-29.646,-1.50482081984275,-0.685440594208854));
#53956=CARTESIAN_POINT('Ctrl Pts',(-29.646,-1.51109469121476,-0.674967470155894));
#53957=CARTESIAN_POINT('Ctrl Pts',(-29.646,-1.51725645140333,-0.664430682827637));
#53958=CARTESIAN_POINT('Ctrl Pts',(-29.646,-1.52330452002809,-0.653834544117298));
#53959=CARTESIAN_POINT('Ctrl Pts',(-29.646,-1.55542245224318,-0.597564338543406));
#53960=CARTESIAN_POINT('Ctrl Pts',(-29.646,-1.58434610869271,-0.539607784254353));
#53961=CARTESIAN_POINT('Ctrl Pts',(-29.646,-1.60998192831617,-0.480318248615203));
#53962=CARTESIAN_POINT('Ctrl Pts',(-29.646,-1.63611509124052,-0.419878476557027));
#53963=CARTESIAN_POINT('Ctrl Pts',(-29.646,-1.65883236197299,-0.358052705230473));
#53964=CARTESIAN_POINT('Ctrl Pts',(-29.646,-1.67800021593047,-0.295174352807214));
#53965=CARTESIAN_POINT('Ctrl Pts',(-29.646,-1.69037848125595,-0.254568610961997));
#53966=CARTESIAN_POINT('Ctrl Pts',(-29.646,-1.70127578873751,-0.213523101715277));
#53967=CARTESIAN_POINT('Ctrl Pts',(-29.646,-1.71064650068833,-0.172121311687352));
#53968=CARTESIAN_POINT('Ctrl Pts',(-29.646,-1.71591839185181,-0.148828979989804));
#53969=CARTESIAN_POINT('Ctrl Pts',(-29.646,-1.72070695331894,-0.125423806591512));
#53970=CARTESIAN_POINT('Ctrl Pts',(-29.646,-1.72500283464754,-0.101920209121272));
#53971=CARTESIAN_POINT('Ctrl Pts',(-29.646,-1.7270982621959,-0.090455719798291));
#53972=CARTESIAN_POINT('Ctrl Pts',(-29.646,-1.7290767393725,-0.0789660350709723));
#53973=CARTESIAN_POINT('Ctrl Pts',(-29.646,-1.73093620036666,-0.0674584042143595));
#53974=CARTESIAN_POINT('Ctrl Pts',(-29.646,-1.74175324651588,-0.000515040285197679));
#53975=CARTESIAN_POINT('Ctrl Pts',(-29.646,-1.74850514784089,0.0667726732139331));
#53976=CARTESIAN_POINT('Ctrl Pts',(-29.646,-1.75107273016818,0.134046743031648));
#53977=CARTESIAN_POINT('Ctrl Pts',(-29.646,-1.7519840544883,0.15792465155534));
#53978=CARTESIAN_POINT('Ctrl Pts',(-29.646,-1.7523678650129,0.181801136382496));
#53979=CARTESIAN_POINT('Ctrl Pts',(-29.646,-1.75221749782202,0.205661030890043));
#53980=CARTESIAN_POINT('Ctrl Pts',(-29.646,-1.75180885673372,0.270503189618104));
#53981=CARTESIAN_POINT('Ctrl Pts',(-29.646,-1.74745894739069,0.335222160736237));
#53982=CARTESIAN_POINT('Ctrl Pts',(-29.646,-1.73938470553461,0.399582523654373));
#53983=CARTESIAN_POINT('Ctrl Pts',(-29.646,-1.73502774243432,0.43431219008673));
#53984=CARTESIAN_POINT('Ctrl Pts',(-29.646,-1.72958541924836,0.468937626840657));
#53985=CARTESIAN_POINT('Ctrl Pts',(-29.646,-1.72308572421693,0.503422468839529));
#53986=CARTESIAN_POINT('Ctrl Pts',(-29.646,-1.71847023632418,0.527910444038297));
#53987=CARTESIAN_POINT('Ctrl Pts',(-29.646,-1.71332147606747,0.552327531312746));
#53988=CARTESIAN_POINT('Ctrl Pts',(-29.646,-1.7076482220736,0.576660653491874));
#53989=CARTESIAN_POINT('Ctrl Pts',(-29.646,-1.70507942959174,0.587678447051176));
#53990=CARTESIAN_POINT('Ctrl Pts',(-29.646,-1.70240254021491,0.598681189081229));
#53991=CARTESIAN_POINT('Ctrl Pts',(-29.646,-1.69962009251516,0.609660631171463));
#53992=CARTESIAN_POINT('Ctrl Pts',(-29.646,-1.68299527966229,0.675261565915201));
#53993=CARTESIAN_POINT('Ctrl Pts',(-29.646,-1.66265693563362,0.739837446467255));
#53994=CARTESIAN_POINT('Ctrl Pts',(-29.646,-1.63886568474381,0.803133427680957));
#53995=CARTESIAN_POINT('Ctrl Pts',(-29.646,-1.61455213843445,0.867818961769251));
#53996=CARTESIAN_POINT('Ctrl Pts',(-29.646,-1.58663225844587,0.931168648803791));
#53997=CARTESIAN_POINT('Ctrl Pts',(-29.646,-1.55532888245165,0.992914874479613));
#53998=CARTESIAN_POINT('Ctrl Pts',(-29.646,-1.52373954286451,1.05522516623404));
#53999=CARTESIAN_POINT('Ctrl Pts',(-29.646,-1.48870429933303,1.11590354521734));
#54000=CARTESIAN_POINT('Ctrl Pts',(-29.646,-1.45040012878564,1.17466536929942));
#54001=CARTESIAN_POINT('Ctrl Pts',(-29.646,-1.43549335870293,1.19753361024327));
#54002=CARTESIAN_POINT('Ctrl Pts',(-29.646,-1.42009097480235,1.2201114031708));
#54003=CARTESIAN_POINT('Ctrl Pts',(-29.646,-1.40420146593038,1.24238107953945));
#54004=CARTESIAN_POINT('Ctrl Pts',(-29.646,-1.3981387582144,1.25087816650674));
#54005=CARTESIAN_POINT('Ctrl Pts',(-29.646,-1.39200638190649,1.25932854263738));
#54006=CARTESIAN_POINT('Ctrl Pts',(-29.646,-1.38581027364365,1.26772416536366));
#54007=CARTESIAN_POINT('Ctrl Pts',(-29.646,-1.34294092093917,1.32581141893628));
#54008=CARTESIAN_POINT('Ctrl Pts',(-29.646,-1.29695511274685,1.38137692796401));
#54009=CARTESIAN_POINT('Ctrl Pts',(-29.646,-1.24809388707593,1.43414001244329));
#54010=CARTESIAN_POINT('Ctrl Pts',(-29.646,-1.19912143132231,1.48702320938739));
#54011=CARTESIAN_POINT('Ctrl Pts',(-29.646,-1.14726001944392,1.53709221743024));
#54012=CARTESIAN_POINT('Ctrl Pts',(-29.646,-1.09270275532193,1.58404817835453));
#54013=CARTESIAN_POINT('Ctrl Pts',(-29.646,-1.03931253040024,1.62999970021889));
#54014=CARTESIAN_POINT('Ctrl Pts',(-29.646,-0.983339984605486,1.67297078948674));
#54015=CARTESIAN_POINT('Ctrl Pts',(-29.646,-0.924926350941029,1.71265217222693));
#54016=CARTESIAN_POINT('Ctrl Pts',(-29.646,-0.904101655375222,1.72679874492503));
#54017=CARTESIAN_POINT('Ctrl Pts',(-29.646,-0.882966376139423,1.74052687656736));
#54018=CARTESIAN_POINT('Ctrl Pts',(-29.646,-0.861525859670494,1.75382131162756));
#54019=CARTESIAN_POINT('Ctrl Pts',(-29.646,-0.90554702707136,-1.26790990717739));
#54020=CARTESIAN_POINT('Ctrl Pts',(-29.6115450158799,-0.514141345293391,
-1.54438147758941));
#54021=CARTESIAN_POINT('Ctrl Pts',(-29.5400412501341,0.585902364535579,
-1.72181409200425));
#54022=CARTESIAN_POINT('Ctrl Pts',(-29.4314887027624,1.77417745764817,-0.482217988040945));
#54023=CARTESIAN_POINT('Ctrl Pts',(-29.320342357885,1.36710299288539,1.22961697865478));
#54024=CARTESIAN_POINT('Ctrl Pts',(-29.2091960130075,-0.291685088526501,
1.81519477428025));
#54025=CARTESIAN_POINT('Ctrl Pts',(-29.1197298185113,-1.41188498103577,
0.949241954866662));
#54026=CARTESIAN_POINT('Ctrl Pts',(-29.0673124056409,-1.554112608544,0.216012872988254));
#54027=CARTESIAN_POINT('Ctrl Pts',(-29.0519437743963,-1.55324480116087,
0.00070803006655188));
#54028=CARTESIAN_POINT('Origin',(-29.646,-2.59090492670967E-16,0.));
#54029=CARTESIAN_POINT('',(-29.646,-1.954,-2.39295984553393E-16));
#54030=CARTESIAN_POINT('Origin',(-29.646,0.,0.));
#54031=CARTESIAN_POINT('Origin',(-29.646,0.,0.));
#54032=CARTESIAN_POINT('',(-29.646,0.903606778650208,-1.26612599672284));
#54033=CARTESIAN_POINT('Ctrl Pts',(-29.646,0.863566668009735,1.75642846275435));
#54034=CARTESIAN_POINT('Ctrl Pts',(-29.646,0.902259155469474,1.73266520248623));
#54035=CARTESIAN_POINT('Ctrl Pts',(-29.646,0.940006532226865,1.70749215717109));
#54036=CARTESIAN_POINT('Ctrl Pts',(-29.646,0.976720689600575,1.68090467162269));
#54037=CARTESIAN_POINT('Ctrl Pts',(-29.646,1.0349027939429,1.63877062936124));
#54038=CARTESIAN_POINT('Ctrl Pts',(-29.646,1.09049234196888,1.59308558101157));
#54039=CARTESIAN_POINT('Ctrl Pts',(-29.646,1.14332803524928,1.54419031207811));
#54040=CARTESIAN_POINT('Ctrl Pts',(-29.646,1.16845341136095,1.52093875719617));
#54041=CARTESIAN_POINT('Ctrl Pts',(-29.646,1.19295541948053,1.49696080557489));
#54042=CARTESIAN_POINT('Ctrl Pts',(-29.646,1.21681313452585,1.47229119208527));
#54043=CARTESIAN_POINT('Ctrl Pts',(-29.646,1.2292556555639,1.45942524141639));
#54044=CARTESIAN_POINT('Ctrl Pts',(-29.646,1.24152289307511,1.44637114719752));
#54045=CARTESIAN_POINT('Ctrl Pts',(-29.646,1.25361161098408,1.43313375371991));
#54046=CARTESIAN_POINT('Ctrl Pts',(-29.646,1.26358724145162,1.42221023423005));
#54047=CARTESIAN_POINT('Ctrl Pts',(-29.646,1.27343483093232,1.41116895221076));
#54048=CARTESIAN_POINT('Ctrl Pts',(-29.646,1.28315121238943,1.40001516631078));
#54049=CARTESIAN_POINT('Ctrl Pts',(-29.646,1.3300441200689,1.34618510058174));
#54050=CARTESIAN_POINT('Ctrl Pts',(-29.646,1.37389955022329,1.28972022694498));
#54051=CARTESIAN_POINT('Ctrl Pts',(-29.646,1.41455393311167,1.23095477641172));
#54052=CARTESIAN_POINT('Ctrl Pts',(-29.646,1.44358986833681,1.18898366053364));
#54053=CARTESIAN_POINT('Ctrl Pts',(-29.646,1.47099202754879,1.1458383448938));
#54054=CARTESIAN_POINT('Ctrl Pts',(-29.646,1.49668525991621,1.10163578501629));
#54055=CARTESIAN_POINT('Ctrl Pts',(-29.646,1.51149551265388,1.07615627064161));
#54056=CARTESIAN_POINT('Ctrl Pts',(-29.646,1.52573769742341,1.05032541750307));
#54057=CARTESIAN_POINT('Ctrl Pts',(-29.646,1.53939530583147,1.02416547210538));
#54058=CARTESIAN_POINT('Ctrl Pts',(-29.646,1.54521957948012,1.01300958916617));
#54059=CARTESIAN_POINT('Ctrl Pts',(-29.646,1.55093325590683,1.0018019983193));
#54060=CARTESIAN_POINT('Ctrl Pts',(-29.646,1.55653443638647,0.990546796296277));
#54061=CARTESIAN_POINT('Ctrl Pts',(-29.646,1.58755327688888,0.928216486169085));
#54062=CARTESIAN_POINT('Ctrl Pts',(-29.646,1.6151376920719,0.864404941366738));
#54063=CARTESIAN_POINT('Ctrl Pts',(-29.646,1.6391334354648,0.799420358132647));
#54064=CARTESIAN_POINT('Ctrl Pts',(-29.646,1.66253760074651,0.736037869752487));
#54065=CARTESIAN_POINT('Ctrl Pts',(-29.646,1.68252795024664,0.671538496957767));
#54066=CARTESIAN_POINT('Ctrl Pts',(-29.646,1.69891301949968,0.606203195144271));
#54067=CARTESIAN_POINT('Ctrl Pts',(-29.646,1.70967608762625,0.563285567294857));
#54068=CARTESIAN_POINT('Ctrl Pts',(-29.646,1.71888251024604,0.520007171308568));
#54069=CARTESIAN_POINT('Ctrl Pts',(-29.646,1.72646591175805,0.47644935798757));
#54070=CARTESIAN_POINT('Ctrl Pts',(-29.646,1.73282394033038,0.439929885663143));
#54071=CARTESIAN_POINT('Ctrl Pts',(-29.646,1.73804092762139,0.403213996643961));
#54072=CARTESIAN_POINT('Ctrl Pts',(-29.646,1.74207225008614,0.366351346889232));
#54073=CARTESIAN_POINT('Ctrl Pts',(-29.646,1.74334867076358,0.354679681130935));
#54074=CARTESIAN_POINT('Ctrl Pts',(-29.646,1.74450615115825,0.342992647905779));
#54075=CARTESIAN_POINT('Ctrl Pts',(-29.646,1.74554204935843,0.331307707853706));
#54076=CARTESIAN_POINT('Ctrl Pts',(-29.646,1.7512962238706,0.266400572951581));
#54077=CARTESIAN_POINT('Ctrl Pts',(-29.646,1.75331678834241,0.20144064594388));
#54078=CARTESIAN_POINT('Ctrl Pts',(-29.646,1.7514364731807,0.136688241949958));
#54079=CARTESIAN_POINT('Ctrl Pts',(-29.646,1.75089895462669,0.1181777181439));
#54080=CARTESIAN_POINT('Ctrl Pts',(-29.646,1.7500423376016,0.0996841942035913));
#54081=CARTESIAN_POINT('Ctrl Pts',(-29.646,1.74886193315568,0.0812138946393991));
#54082=CARTESIAN_POINT('Ctrl Pts',(-29.646,1.7444812283952,0.0126671100964298));
#54083=CARTESIAN_POINT('Ctrl Pts',(-29.646,1.73564516145986,-0.0555619386623527));
#54084=CARTESIAN_POINT('Ctrl Pts',(-29.646,1.72254696331046,-0.123135794734825));
#54085=CARTESIAN_POINT('Ctrl Pts',(-29.646,1.7107923019786,-0.183778318535385));
#54086=CARTESIAN_POINT('Ctrl Pts',(-29.646,1.69560382797953,-0.243893450349329));
#54087=CARTESIAN_POINT('Ctrl Pts',(-29.646,1.67708883824234,-0.303212355847263));
#54088=CARTESIAN_POINT('Ctrl Pts',(-29.646,1.67396734919769,-0.313213080464503));
#54089=CARTESIAN_POINT('Ctrl Pts',(-29.646,1.67075231970824,-0.32318750802379));
#54090=CARTESIAN_POINT('Ctrl Pts',(-29.646,1.66744711192406,-0.333126627485946));
#54091=CARTESIAN_POINT('Ctrl Pts',(-29.646,1.64699549224018,-0.394626873311822));
#54092=CARTESIAN_POINT('Ctrl Pts',(-29.646,1.62306700922488,-0.454867564271816));
#54093=CARTESIAN_POINT('Ctrl Pts',(-29.646,1.59584883350397,-0.513575166957551));
#54094=CARTESIAN_POINT('Ctrl Pts',(-29.646,1.56873097546522,-0.572066391782911));
#54095=CARTESIAN_POINT('Ctrl Pts',(-29.646,1.53834687411596,-0.629036647008692));
#54096=CARTESIAN_POINT('Ctrl Pts',(-29.646,1.50484185692085,-0.684183082745647));
#54097=CARTESIAN_POINT('Ctrl Pts',(-29.646,1.47201694913541,-0.738210115688802));
#54098=CARTESIAN_POINT('Ctrl Pts',(-29.646,1.43619579268168,-0.790487244163948));
#54099=CARTESIAN_POINT('Ctrl Pts',(-29.646,1.39748800398724,-0.840688000782997));
#54100=CARTESIAN_POINT('Ctrl Pts',(-29.646,1.39006351372884,-0.850316942168009));
#54101=CARTESIAN_POINT('Ctrl Pts',(-29.646,1.38253276005615,-0.859869351508118));
#54102=CARTESIAN_POINT('Ctrl Pts',(-29.646,1.37489643439059,-0.869342715932));
#54103=CARTESIAN_POINT('Ctrl Pts',(-29.646,1.36836089236766,-0.877450485820595));
#54104=CARTESIAN_POINT('Ctrl Pts',(-29.646,1.36175071282073,-0.885496939562918));
#54105=CARTESIAN_POINT('Ctrl Pts',(-29.646,1.35507157412216,-0.893474782751297));
#54106=CARTESIAN_POINT('Ctrl Pts',(-29.646,1.31523219178395,-0.941060610709032));
#54107=CARTESIAN_POINT('Ctrl Pts',(-29.646,1.27288888818335,-0.986274661689286));
#54108=CARTESIAN_POINT('Ctrl Pts',(-29.646,1.22818063142926,-1.02884993242326));
#54109=CARTESIAN_POINT('Ctrl Pts',(-29.646,1.18427440391157,-1.07066143793007));
#54110=CARTESIAN_POINT('Ctrl Pts',(-29.646,1.13808660486174,-1.10992852640867));
#54111=CARTESIAN_POINT('Ctrl Pts',(-29.646,1.08972540441639,-1.14635444573824));
#54112=CARTESIAN_POINT('Ctrl Pts',(-29.646,1.04290945083493,-1.18161647672157));
#54113=CARTESIAN_POINT('Ctrl Pts',(-29.646,0.994056159108196,-1.21421629893641));
#54114=CARTESIAN_POINT('Ctrl Pts',(-29.646,0.94325105145388,-1.24383738917956));
#54115=CARTESIAN_POINT('Ctrl Pts',(-29.646,0.930165355350817,-1.25146679108538));
#54116=CARTESIAN_POINT('Ctrl Pts',(-29.646,0.916950133464095,-1.2588983186305));
#54117=CARTESIAN_POINT('Ctrl Pts',(-29.646,0.903606778650087,-1.26612599672292));
#54118=CARTESIAN_POINT('Origin',(-29.646,0.,0.));
#54119=CARTESIAN_POINT('Origin',(-30.9400562256037,0.,0.));
#54120=CARTESIAN_POINT('Ctrl Pts',(-29.646,0.903606778650087,-1.26612599672292));
#54121=CARTESIAN_POINT('Ctrl Pts',(-29.6089512183742,1.32465582191086,-0.965632388172658));
#54122=CARTESIAN_POINT('Ctrl Pts',(-29.5348536551225,1.83614857151059,0.0831884196457774));
#54123=CARTESIAN_POINT('Ctrl Pts',(-29.4237073102452,0.924038956922092,
1.59090722470862));
#54124=CARTESIAN_POINT('Ctrl Pts',(-29.3125609653677,-0.83473688776688,
1.63754421834404));
#54125=CARTESIAN_POINT('Ctrl Pts',(-29.2346772704873,-1.53141980147719,
0.621433224781769));
#54126=CARTESIAN_POINT('Ctrl Pts',(-29.1938423572326,-1.55773945610431,
0.0536831291795148));
#54127=CARTESIAN_POINT('Ctrl Pts',(-29.1900562256037,-1.55737653422887,
0.00100621910560853));
#54128=CARTESIAN_POINT('Ctrl Pts',(-29.8760740822721,1.13509973994375,-1.59049193030949));
#54129=CARTESIAN_POINT('Ctrl Pts',(-29.8390253006463,1.6640163780225,-1.21301554901262));
#54130=CARTESIAN_POINT('Ctrl Pts',(-29.7649277373946,2.30654728944499,0.104500271287817));
#54131=CARTESIAN_POINT('Ctrl Pts',(-29.6537813925172,1.16076639140178,1.99847812091342));
#54132=CARTESIAN_POINT('Ctrl Pts',(-29.5426350476398,-1.04858622867039,
2.05706293966191));
#54133=CARTESIAN_POINT('Ctrl Pts',(-29.4314887027624,-2.29751693097514,
0.235499367719248));
#54134=CARTESIAN_POINT('Ctrl Pts',(-29.320342357885,-1.44347707856157,-1.80319291664826));
#54135=CARTESIAN_POINT('Ctrl Pts',(-29.2091960130075,0.732117470005603,
-2.19036286313464));
#54136=CARTESIAN_POINT('Ctrl Pts',(-29.0980496681301,2.23742980466302,-0.572814850018687));
#54137=CARTESIAN_POINT('Ctrl Pts',(-28.9869033232526,1.69455056349597,1.56933369051493));
#54138=CARTESIAN_POINT('Ctrl Pts',(-28.8757569783753,-0.399606399986678,
2.27473567517142));
#54139=CARTESIAN_POINT('Ctrl Pts',(-28.7646106334978,-2.12793746980263,
0.897818014163103));
#54140=CARTESIAN_POINT('Ctrl Pts',(-28.6534642886204,-1.90827750560971,
-1.30102961800398));
#54141=CARTESIAN_POINT('Ctrl Pts',(-28.542317943743,0.0582967826181247,
-2.30884711344785));
#54142=CARTESIAN_POINT('Ctrl Pts',(-28.4311715988656,1.97150238108163,-1.20306522421591));
#54143=CARTESIAN_POINT('Ctrl Pts',(-28.3200252539881,2.07991891070671,1.00405403493572));
#54144=CARTESIAN_POINT('Ctrl Pts',(-28.2088789091107,0.284296424689126,
2.29202073726512));
#54145=CARTESIAN_POINT('Ctrl Pts',(-28.0977325642333,-1.7715818298528,1.48178390263166));
#54146=CARTESIAN_POINT('Ctrl Pts',(-27.9865862193559,-2.20568535982826,
-0.684936177450616));
#54147=CARTESIAN_POINT('Ctrl Pts',(-27.8754398744784,-0.620618745970624,
-2.22463870679357));
#54148=CARTESIAN_POINT('Ctrl Pts',(-27.764293529601,1.53258634975486,-1.72782071366884));
#54149=CARTESIAN_POINT('Ctrl Pts',(-27.6531471847236,2.28280236854648,0.350711595825784));
#54150=CARTESIAN_POINT('Ctrl Pts',(-27.5420008398461,0.94325239047631,2.10818883105081));
#54151=CARTESIAN_POINT('Ctrl Pts',(-27.4308544949688,-1.25978747172194,
1.93574812290515));
#54152=CARTESIAN_POINT('Ctrl Pts',(-27.3197081500913,-2.30956893500566,
-0.00875164606705387));
#54153=CARTESIAN_POINT('Ctrl Pts',(-27.2085618052139,-1.24508125418542,
-1.94523981057524));
#54154=CARTESIAN_POINT('Ctrl Pts',(-27.0974154603365,0.959202184405071,
-2.1009798730201));
#54155=CARTESIAN_POINT('Ctrl Pts',(-26.986269115459,2.28539467337763,-0.333401322767505));
#54156=CARTESIAN_POINT('Ctrl Pts',(-26.8751227705816,1.51944807776828,1.73938575175027));
#54157=CARTESIAN_POINT('Ctrl Pts',(-26.7639764257042,-0.637460327196598,
2.21987152481952));
#54158=CARTESIAN_POINT('Ctrl Pts',(-26.6528300808268,-2.21081277979495,
0.668200649323706));
#54159=CARTESIAN_POINT('Ctrl Pts',(-26.5416837359493,-1.76030131128423,
-1.4951670637397));
#54160=CARTESIAN_POINT('Ctrl Pts',(-26.430537391072,0.301658375125117,-2.28980075112679));
#54161=CARTESIAN_POINT('Ctrl Pts',(-26.3193910461945,2.08746826383544,-0.988261859306003));
#54162=CARTESIAN_POINT('Ctrl Pts',(-26.2082447013171,1.9623285939949,1.21797033800769));
#54163=CARTESIAN_POINT('Ctrl Pts',(-26.0970983564397,0.0407970817586391,
2.30922516295313));
#54164=CARTESIAN_POINT('Ctrl Pts',(-25.9859520115622,-1.91808166431569,
1.2865255473956));
#54165=CARTESIAN_POINT('Ctrl Pts',(-25.8748056666848,-2.12107392666094,
-0.913909542966534));
#54166=CARTESIAN_POINT('Ctrl Pts',(-25.7636593218074,-0.382352700941006,
-2.27771632719524));
#54167=CARTESIAN_POINT('Ctrl Pts',(-25.65251297693,1.70638904376409,-1.55641308347398));
#54168=CARTESIAN_POINT('Ctrl Pts',(-25.5413666320525,2.23303595503733,0.589691172223087));
#54169=CARTESIAN_POINT('Ctrl Pts',(-25.4302202871751,0.715474987117585,
2.19596921606308));
#54170=CARTESIAN_POINT('Ctrl Pts',(-25.3190739422977,-1.45705958421952,
1.79197171381733));
#54171=CARTESIAN_POINT('Ctrl Pts',(-25.2079275974203,-2.29574519723769,
-0.252466323392859));
#54172=CARTESIAN_POINT('Ctrl Pts',(-25.0967812525429,-1.0328164541474,-2.06578687843878));
#54173=CARTESIAN_POINT('Ctrl Pts',(-24.9856349076654,1.17559260177244,-1.9880058575732));
#54174=CARTESIAN_POINT('Ctrl Pts',(-24.874488562788,2.30781851167389,-0.0903270295247155));
#54175=CARTESIAN_POINT('Ctrl Pts',(-24.7633422179106,1.3273776843161,1.89004067106162));
#54176=CARTESIAN_POINT('Ctrl Pts',(-24.6521958730331,-0.868196251320992,
2.14019170269385));
#54177=CARTESIAN_POINT('Ctrl Pts',(-24.5410495281557,-2.26898960421259,
0.431128091247411));
#54178=CARTESIAN_POINT('Ctrl Pts',(-24.4299031832783,-1.59266171045552,
-1.67260692666757));
#54179=CARTESIAN_POINT('Ctrl Pts',(-24.3187568384009,0.541650596878888,
-2.24517257376536));
#54180=CARTESIAN_POINT('Ctrl Pts',(-24.2076104935235,2.18011490167143,-0.762420009310885));
#54181=CARTESIAN_POINT('Ctrl Pts',(-24.096464148646,1.82281731580137,1.41828145595369));
#54182=CARTESIAN_POINT('Ctrl Pts',(-23.9853178037686,-0.203158067613754,
2.30063296826132));
#54183=CARTESIAN_POINT('Ctrl Pts',(-23.8741714588912,-2.04315466210664,
1.07689566894818));
#54184=CARTESIAN_POINT('Ctrl Pts',(-23.7630251140138,-2.01276809090682,
-1.13267376914748));
#54185=CARTESIAN_POINT('Ctrl Pts',(-23.6518787691364,-0.139815401979066,
-2.30534962824663));
#54186=CARTESIAN_POINT('Ctrl Pts',(-23.5407324242589,1.86112973853166,-1.3676188619058));
#54187=CARTESIAN_POINT('Ctrl Pts',(-23.4295860793815,2.15832440107783,0.822083350275042));
#54188=CARTESIAN_POINT('Ctrl Pts',(-23.3184397345041,0.479705043887776,
2.25921852107228));
#54189=CARTESIAN_POINT('Ctrl Pts',(-23.2072933896267,-1.63805494970446,
1.62817727438881));
#54190=CARTESIAN_POINT('Ctrl Pts',(-23.0961470447492,-2.25627579472933,
-0.493360713075091));
#54191=CARTESIAN_POINT('Ctrl Pts',(-22.9850006998718,-0.809014108309205,
-2.16325713396352));
#54192=CARTESIAN_POINT('Ctrl Pts',(-22.8738543549944,1.37885052758575,-1.85282391976786));
#54193=CARTESIAN_POINT('Ctrl Pts',(-22.762708010117,2.30446181446416,0.153756303168402));
#54194=CARTESIAN_POINT('Ctrl Pts',(-22.6515616652395,1.12047921513559,2.01958203189089));
#54195=CARTESIAN_POINT('Ctrl Pts',(-22.5404153203621,-1.08923359462026,
2.03660389654887));
#54196=CARTESIAN_POINT('Ctrl Pts',(-22.4292689754847,-2.30181964903589,
0.189239420839657));
#54197=CARTESIAN_POINT('Ctrl Pts',(-22.3181226306073,-1.4072305581405,-1.83136217371742));
#54198=CARTESIAN_POINT('Ctrl Pts',(-22.2069762857299,0.775592064464368,
-2.17546367577749));
#54199=CARTESIAN_POINT('Ctrl Pts',(-22.0958299408524,2.24840757516354,-0.528061200084454));
#54200=CARTESIAN_POINT('Ctrl Pts',(-21.984683595975,1.66294342833263,1.60274901630066));
#54201=CARTESIAN_POINT('Ctrl Pts',(-21.8735372510976,-0.444843747458639,
2.26634050738947));
#54202=CARTESIAN_POINT('Ctrl Pts',(-21.7623909062202,-2.14540367215556,
0.855235837993748));
#54203=CARTESIAN_POINT('Ctrl Pts',(-21.6512445613427,-1.88197771441436,
-1.33878494820309));
#54204=CARTESIAN_POINT('Ctrl Pts',(-21.5400982164654,0.104283768475023,
-2.30722997352238));
#54205=CARTESIAN_POINT('Ctrl Pts',(-21.4289518715878,1.99507983769398,-1.16354703227434));
#54206=CARTESIAN_POINT('Ctrl Pts',(-21.3178055267105,2.05950230346372,1.04529207263571));
#54207=CARTESIAN_POINT('Ctrl Pts',(-21.206659181833,0.238576337445077,2.29723019880436));
#54208=CARTESIAN_POINT('Ctrl Pts',(-21.0955128369556,-1.80075167789753,
1.4461945407298));
#54209=CARTESIAN_POINT('Ctrl Pts',(-20.9843664920782,-2.19160163800585,
-0.728743792685421));
#54210=CARTESIAN_POINT('Ctrl Pts',(-20.8732201472008,-0.576174302687003,
-2.23656174249909));
#54211=CARTESIAN_POINT('Ctrl Pts',(-20.7620738023233,1.56670537690975,-1.69694417028066));
#54212=CARTESIAN_POINT('Ctrl Pts',(-20.6509274574459,2.27536207920589,0.396122031196596));
#54213=CARTESIAN_POINT('Ctrl Pts',(-20.5397811125685,0.901063923638144,
2.12656273375728));
#54214=CARTESIAN_POINT('Ctrl Pts',(-20.4286347676911,-1.29810315900734,
1.91026528096561));
#54215=CARTESIAN_POINT('Ctrl Pts',(-20.3174884228136,-2.3089361713204,-0.0547632345256441));
#54216=CARTESIAN_POINT('Ctrl Pts',(-20.2063420779362,-1.20607929730647,
-1.96965935727377));
#54217=CARTESIAN_POINT('Ctrl Pts',(-20.0951957330588,1.00086942839655,-2.08145277207738));
#54218=CARTESIAN_POINT('Ctrl Pts',(-19.9840493881814,2.2915833899632,-0.287803443225016));
#54219=CARTESIAN_POINT('Ctrl Pts',(-19.872903043304,1.48449287550998,1.76931234033099));
#54220=CARTESIAN_POINT('Ctrl Pts',(-19.7617566984265,-0.681560098046438,
2.20673085985544));
#54221=CARTESIAN_POINT('Ctrl Pts',(-19.6506103535491,-2.22368647542462,
0.624022206416638));
#54222=CARTESIAN_POINT('Ctrl Pts',(-19.5394640086717,-1.73016385052689,
-1.52994062153321));
#54223=CARTESIAN_POINT('Ctrl Pts',(-19.4283176637943,0.347217989697661,
-2.28333635777074));
#54224=CARTESIAN_POINT('Ctrl Pts',(-19.3171713189168,2.10674299078965,-0.946477271700759));
#54225=CARTESIAN_POINT('Ctrl Pts',(-19.2060249740394,1.93767359934984,1.25682388482638));
#54226=CARTESIAN_POINT('Ctrl Pts',(-19.094878629162,-0.00521749440511517,
2.3095796225373));
#54227=CARTESIAN_POINT('Ctrl Pts',(-18.9837322842846,-1.94333229105276,
1.24805643367561));
#54228=CARTESIAN_POINT('Ctrl Pts',(-18.8725859394071,-2.10244519912854,
-0.955986108554305));
#54229=CARTESIAN_POINT('Ctrl Pts',(-18.7614395945297,-0.336898080152378,
-2.28488182159977));
#54230=CARTESIAN_POINT('Ctrl Pts',(-18.6502932496523,1.73705863177231,-1.5221079346987));
#54231=CARTESIAN_POINT('Ctrl Pts',(-18.5391469047749,2.22084437771726,0.634062698042624));
#54232=CARTESIAN_POINT('Ctrl Pts',(-18.4280005598974,0.671582888059023,
2.20978770010916));
#54233=CARTESIAN_POINT('Ctrl Pts',(-18.31685421502,-1.4924716720845,1.76258717886881));
#54234=CARTESIAN_POINT('Ctrl Pts',(-18.2057078701426,-2.29025967271958,
-0.298154132290432));
#54235=CARTESIAN_POINT('Ctrl Pts',(-18.0945615252652,-0.991454979533412,
-2.08595356579331));
#54236=CARTESIAN_POINT('Ctrl Pts',(-17.9834151803877,1.21496612549574,-1.96419005419163));
#54237=CARTESIAN_POINT('Ctrl Pts',(-17.8722688355103,2.3091600310083,-0.0443306471998567));
#54238=CARTESIAN_POINT('Ctrl Pts',(-17.7611224906329,1.28945912033737,1.91611075673255));
#54239=CARTESIAN_POINT('Ctrl Pts',(-17.6499761457555,-0.910662771798187,
2.12246992231887));
#54240=CARTESIAN_POINT('Ctrl Pts',(-17.5388298008781,-2.27712857828129,
0.385837651172181));
#54241=CARTESIAN_POINT('Ctrl Pts',(-17.4276834560006,-1.55902240500851,
-1.70400539781096));
#54242=CARTESIAN_POINT('Ctrl Pts',(-17.3165371111232,0.586273454560011,
-2.23393569548582));
#54243=CARTESIAN_POINT('Ctrl Pts',(-17.2053907662458,2.19487181381747,-0.718834456601151));
#54244=CARTESIAN_POINT('Ctrl Pts',(-17.0942444213684,1.79419923164516,1.45431577460032));
#54245=CARTESIAN_POINT('Ctrl Pts',(-16.983098076491,-0.24895304186277,2.29612883742065));
#54246=CARTESIAN_POINT('Ctrl Pts',(-16.8719517316135,-2.06420402762972,
1.03597634500247));
#54247=CARTESIAN_POINT('Ctrl Pts',(-16.7608053867361,-1.98980244061841,
-1.17254914711346));
#54248=CARTESIAN_POINT('Ctrl Pts',(-16.6496590418587,-0.0938583844972828,
-2.30767758986106));
#54249=CARTESIAN_POINT('Ctrl Pts',(-16.5385126969813,1.88800728371649,-1.33026830065251));
#54250=CARTESIAN_POINT('Ctrl Pts',(-16.4273663521038,2.14151772476039,0.864920279346345));
#54251=CARTESIAN_POINT('Ctrl Pts',(-16.3162200072264,0.434599630602511,
2.26832722863514));
#54252=CARTESIAN_POINT('Ctrl Pts',(-16.205073662349,-1.67016785203829,1.59521929561588));
#54253=CARTESIAN_POINT('Ctrl Pts',(-16.0939273174715,-2.24599878754927,
-0.538214363813031));
#54254=CARTESIAN_POINT('Ctrl Pts',(-15.9827809725941,-0.765755163307141,
-2.17894568196545));
#54255=CARTESIAN_POINT('Ctrl Pts',(-15.8716346277167,1.41549049130265,-1.82498545860486));
#54256=CARTESIAN_POINT('Ctrl Pts',(-15.7604882828393,2.30094115044168,0.199637364467602));
#54257=CARTESIAN_POINT('Ctrl Pts',(-15.6493419379619,1.08002087601742,2.04150438707684));
#54258=CARTESIAN_POINT('Ctrl Pts',(-15.5381955930844,-1.12959247317232,
2.01449896987808));
#54259=CARTESIAN_POINT('Ctrl Pts',(-15.427049248207,-2.30513298142682,0.143342921086773));
#54260=CARTESIAN_POINT('Ctrl Pts',(-15.3159029033296,-1.37046519115816,
-1.85903480734257));
#54261=CARTESIAN_POINT('Ctrl Pts',(-15.2047565584522,0.818779685343973,
-2.15957983921769));
#54262=CARTESIAN_POINT('Ctrl Pts',(-15.0936102135747,2.25848182370628,-0.483161574502515));
#54263=CARTESIAN_POINT('Ctrl Pts',(-14.9824638686973,1.63068194598152,1.63556156904512));
#54264=CARTESIAN_POINT('Ctrl Pts',(-14.8713175238199,-0.489907546220147,
2.25702810156277));
#54265=CARTESIAN_POINT('Ctrl Pts',(-14.7601711789425,-2.16201663496024,
0.81232341172874));
#54266=CARTESIAN_POINT('Ctrl Pts',(-14.649024834065,-1.85493168960417,-1.37601369251531));
#54267=CARTESIAN_POINT('Ctrl Pts',(-14.5378784891876,0.15022979889931,-2.30469439679324));
#54268=CARTESIAN_POINT('Ctrl Pts',(-14.4267321443102,2.01786509222139,-1.12356829996301));
#54269=CARTESIAN_POINT('Ctrl Pts',(-14.3155857994328,2.03826827476513,1.08611587557377));
#54270=CARTESIAN_POINT('Ctrl Pts',(-14.2044394545554,0.1927614804521,2.30152737692633));
#54271=CARTESIAN_POINT('Ctrl Pts',(-14.0932931096779,-1.82920666292977,
1.41003129021336));
#54272=CARTESIAN_POINT('Ctrl Pts',(-13.9821467648005,-2.17664795214331,
-0.772262227172698));
#54273=CARTESIAN_POINT('Ctrl Pts',(-13.8710004199231,-0.531501131002706,
-2.24759689509269));
#54274=CARTESIAN_POINT('Ctrl Pts',(-13.7598540750456,1.60020247725313,-1.66539403351891));
#54275=CARTESIAN_POINT('Ctrl Pts',(-13.6487077301682,2.26701856100407,0.441375236222479));
#54276=CARTESIAN_POINT('Ctrl Pts',(-13.5375613852908,0.858517767645496,
2.14409246482619));
#54277=CARTESIAN_POINT('Ctrl Pts',(-13.4264150404134,-1.33590354843874,
1.88402414112882));
#54278=CARTESIAN_POINT('Ctrl Pts',(-13.315268695536,-2.30738684894824,-0.100753086246275));
#54279=CARTESIAN_POINT('Ctrl Pts',(-13.2041223506585,-1.16659857303008,
-1.99329702364993));
#54280=CARTESIAN_POINT('Ctrl Pts',(-13.0929760057811,1.04213936552734,-2.06109941485259));
#54281=CARTESIAN_POINT('Ctrl Pts',(-12.9818296609037,2.29686243593069,-0.242091316444785));
#54282=CARTESIAN_POINT('Ctrl Pts',(-12.8706833160263,1.44894838651503,1.79853657963994));
#54283=CARTESIAN_POINT('Ctrl Pts',(-12.7595369711489,-0.725389315675418,
2.19271420750434));
#54284=CARTESIAN_POINT('Ctrl Pts',(-12.6483906262714,-2.23567745285949,
0.579596050593111));
#54285=CARTESIAN_POINT('Ctrl Pts',(-12.537244281394,-1.69933958110716,-1.56410685158336));
#54286=CARTESIAN_POINT('Ctrl Pts',(-12.4260979365166,0.3926397720497,-2.27596556751023));
#54287=CARTESIAN_POINT('Ctrl Pts',(-12.3149515916392,2.12518142161832,-0.904316968930544));
#54288=CARTESIAN_POINT('Ctrl Pts',(-12.2038052467617,1.9122494226383,1.29517852078659));
#54289=CARTESIAN_POINT('Ctrl Pts',(-12.0926589018843,-0.0512299994234969,
2.30901726763714));
#54290=CARTESIAN_POINT('Ctrl Pts',(-11.9815125570069,-1.96781148944065,
1.20909188944132));
#54291=CARTESIAN_POINT('Ctrl Pts',(-11.8703662121295,-2.08298188152774,
-0.997683184339907));
#54292=CARTESIAN_POINT('Ctrl Pts',(-11.759219867252,-0.291309723753528,
-2.29114030559764));
#54293=CARTESIAN_POINT('Ctrl Pts',(-11.6480735223746,1.76703867415875,-1.48719856748004));
#54294=CARTESIAN_POINT('Ctrl Pts',(-11.5369271774972,2.20777121039822,0.678182525301448));
#54295=CARTESIAN_POINT('Ctrl Pts',(-11.4257808326198,0.627424196364101,
2.22272898323306));
#54296=CARTESIAN_POINT('Ctrl Pts',(-11.3146344877423,-1.5272913059653,1.73250296444486));
#54297=CARTESIAN_POINT('Ctrl Pts',(-11.2034881428649,-2.28386500299402,
-0.343723585438356));
#54298=CARTESIAN_POINT('Ctrl Pts',(-11.0923417979875,-0.949699935336984,
-2.10529220962515));
#54299=CARTESIAN_POINT('Ctrl Pts',(-10.9811954531101,1.25385735428831,-1.9395945427291));
#54300=CARTESIAN_POINT('Ctrl Pts',(-10.8700491082326,2.30958490241829,0.00168333269087447));
#54301=CARTESIAN_POINT('Ctrl Pts',(-10.7589027633552,1.25102869056742,1.94142021995873));
#54302=CARTESIAN_POINT('Ctrl Pts',(-10.6477564184778,-0.952767794099242,
2.10390560282886));
#54303=CARTESIAN_POINT('Ctrl Pts',(-10.5366100736004,-2.28436361968318,
0.340394048354919));
#54304=CARTESIAN_POINT('Ctrl Pts',(-10.4254637287229,-1.52476422749005,
-1.7347274441981));
#54305=CARTESIAN_POINT('Ctrl Pts',(-10.3143173838455,0.630663584176363,
-2.2218120304565));
#54306=CARTESIAN_POINT('Ctrl Pts',(-10.2031710389681,2.20875744607579,-0.674963554195493));
#54307=CARTESIAN_POINT('Ctrl Pts',(-10.0920246940907,1.7648689192416,1.48977278568995));
#54308=CARTESIAN_POINT('Ctrl Pts',(-9.98087834921324,-0.294649191307109,
2.29071323153936));
#54309=CARTESIAN_POINT('Ctrl Pts',(-9.86973200433586,-2.08443398336217,
0.99464577820062));
#54310=CARTESIAN_POINT('Ctrl Pts',(-9.75858565945839,-1.96604691511444,
-1.21195906806146));
#54311=CARTESIAN_POINT('Ctrl Pts',(-9.647439314581,-0.047864108838437,-2.30908949202333));
#54312=CARTESIAN_POINT('Ctrl Pts',(-9.53629296970356,1.91413536245694,-1.29238967392936));
#54313=CARTESIAN_POINT('Ctrl Pts',(-9.42514662482614,2.12386094808125,0.907413868255737));
#54314=CARTESIAN_POINT('Ctrl Pts',(-9.31400027994872,0.389321697940529,
2.27653549732926));
#54315=CARTESIAN_POINT('Ctrl Pts',(-9.2028539350713,-1.70161776182311,1.56162807599489));
#54316=CARTESIAN_POINT('Ctrl Pts',(-9.09170759019387,-2.23483020503478,
-0.58285436410105));
#54317=CARTESIAN_POINT('Ctrl Pts',(-8.98056124531646,-0.722192242889091,
-2.19376927214288));
#54318=CARTESIAN_POINT('Ctrl Pts',(-8.86941490043901,1.45156855961018,-1.79642254824377));
#54319=CARTESIAN_POINT('Ctrl Pts',(-8.75826855556161,2.29650710107497,0.245439177393632));
#54320=CARTESIAN_POINT('Ctrl Pts',(-8.64712221068417,1.03913381005442,2.06261634335842));
#54321=CARTESIAN_POINT('Ctrl Pts',(-8.53597586580677,-1.16950294685762,
1.9915943644173));
#54322=CARTESIAN_POINT('Ctrl Pts',(-8.42482952092932,-2.30753126447749,
0.0973895196946199));
#54323=CARTESIAN_POINT('Ctrl Pts',(-8.31368317605192,-1.33315580208287,
-1.88596947548475));
#54324=CARTESIAN_POINT('Ctrl Pts',(-8.20253683117448,0.86164228210699,-2.14283873232982));
#54325=CARTESIAN_POINT('Ctrl Pts',(-8.09139048629707,2.26765954162825,-0.438070152315537));
#54326=CARTESIAN_POINT('Ctrl Pts',(-7.98024414141964,1.59777314547094,1.66772486660701));
#54327=CARTESIAN_POINT('Ctrl Pts',(-7.86909779654221,-0.534776870484712,
2.24681974218716));
#54328=CARTESIAN_POINT('Ctrl Pts',(-7.75795145166479,-2.17777136012248,
0.769088524240027));
#54329=CARTESIAN_POINT('Ctrl Pts',(-7.64680510678736,-1.82714932809128,
-1.4126962121925));
#54330=CARTESIAN_POINT('Ctrl Pts',(-7.53565876190995,0.196116193858117,
-2.30124394482506));
#54331=CARTESIAN_POINT('Ctrl Pts',(-7.42451241703251,2.0398493317374,-1.08314355415055));
#54332=CARTESIAN_POINT('Ctrl Pts',(-7.31336607215511,2.01622513177459,1.12650853218607));
#54333=CARTESIAN_POINT('Ctrl Pts',(-7.20221972727766,0.146870104548076,
2.30491093699463));
#54334=CARTESIAN_POINT('Ctrl Pts',(-7.09107338240025,-1.85693552310777,
1.37330831138092));
#54335=CARTESIAN_POINT('Ctrl Pts',(-6.97992703752283,-2.16083022056687,
-0.815474103189318));
#54336=CARTESIAN_POINT('Ctrl Pts',(-6.8687806926454,-0.486616973764323,
-2.25773983796448));
#54337=CARTESIAN_POINT('Ctrl Pts',(-6.75763434776797,1.63306435861655,-1.63318279923092));
#54338=CARTESIAN_POINT('Ctrl Pts',(-6.64648800289056,2.25777512342436,0.486453232216203));
#54339=CARTESIAN_POINT('Ctrl Pts',(-6.53534165801313,0.815630813042409,
2.16077107346039));
#54340=CARTESIAN_POINT('Ctrl Pts',(-6.42419531313571,-1.37317363542316,
1.85703511600243));
#54341=CARTESIAN_POINT('Ctrl Pts',(-6.31304896825829,-2.30492158253688,
-0.146702942857817));
#54342=CARTESIAN_POINT('Ctrl Pts',(-6.20190262338086,-1.12665475388528,
-2.01614342759515));
#54343=CARTESIAN_POINT('Ctrl Pts',(-6.09075627850344,1.08299561331934,-2.03992788024932));
#54344=CARTESIAN_POINT('Ctrl Pts',(-5.97960993362602,2.30122971564711,-0.196283088701521));
#54345=CARTESIAN_POINT('Ctrl Pts',(-5.86846358874859,1.41282872061015,1.82704686894083));
#54346=CARTESIAN_POINT('Ctrl Pts',(-5.75731724387116,-0.76893058158095,
2.17782713175243));
#54347=CARTESIAN_POINT('Ctrl Pts',(-5.64617089899375,-2.24678095213377,
0.534939817377955));
#54348=CARTESIAN_POINT('Ctrl Pts',(-5.53502455411632,-1.66784073908135,
-1.59765219123186));
#54349=CARTESIAN_POINT('Ctrl Pts',(-5.4238782092389,0.43790569147873,-2.26769130625355));
#54350=CARTESIAN_POINT('Ctrl Pts',(-5.31273186436147,2.14277623697082,-0.861797687024427));
#54351=CARTESIAN_POINT('Ctrl Pts',(-5.20158551948405,1.88606615628344,1.33301902057307));
#54352=CARTESIAN_POINT('Ctrl Pts',(-5.09043917460662,-0.0972221680979084,
2.30753832148412));
#54353=CARTESIAN_POINT('Ctrl Pts',(-4.97929282972921,-1.99150954217679,
1.16964738212262));
#54354=CARTESIAN_POINT('Ctrl Pts',(-4.86814648485178,-2.06269170004884,
-1.03898421818477));
#54355=CARTESIAN_POINT('Ctrl Pts',(-4.75700013997435,-0.245605728572608,
-2.2964892948106));
#54356=CARTESIAN_POINT('Ctrl Pts',(-4.64585379509694,1.796317269997,-1.45169883949742));
#54357=CARTESIAN_POINT('Ctrl Pts',(-4.5347074502195,2.19382164262593,0.722033140121231));
#54358=CARTESIAN_POINT('Ctrl Pts',(-4.42356110534209,0.58301644133906,2.23478792824183));
#54359=CARTESIAN_POINT('Ctrl Pts',(-4.31241476046466,-1.56150466380355,
1.70173101282442));
#54360=CARTESIAN_POINT('Ctrl Pts',(-4.20126841558724,-2.27656372649916,
-0.389156593512695));
#54361=CARTESIAN_POINT('Ctrl Pts',(-4.09012207070982,-0.907567896709133,
-2.12379513323403));
#54362=CARTESIAN_POINT('Ctrl Pts',(-3.97897572583239,1.29225084982594,-1.91422908666128));
#54363=CARTESIAN_POINT('Ctrl Pts',(-3.86782938095497,2.30909295724377,0.0476966443656992));
#54364=CARTESIAN_POINT('Ctrl Pts',(-3.75668303607755,1.21210165041682,1.96595901384947));
#54365=CARTESIAN_POINT('Ctrl Pts',(-3.64553669120012,-0.994494604154669,
2.08450611355572));
#54366=CARTESIAN_POINT('Ctrl Pts',(-3.5343903463227,-2.29069185636784,0.29481532214432));
#54367=CARTESIAN_POINT('Ctrl Pts',(-3.42324400144527,-1.48990077711358,
-1.76476087032143));
#54368=CARTESIAN_POINT('Ctrl Pts',(-3.31209765656785,0.674803364609756,
-2.20880639137193));
#54369=CARTESIAN_POINT('Ctrl Pts',(-3.20095131169043,2.22176628626919,-0.630824717035695));
#54370=CARTESIAN_POINT('Ctrl Pts',(-3.08980496681301,1.73483802181615,1.52463841391558));
#54371=CARTESIAN_POINT('Ctrl Pts',(-2.97865862193558,-0.34022837674139,
2.28438830085055));
#54372=CARTESIAN_POINT('Ctrl Pts',(-2.86751227705816,-2.10383649800309,
0.952920374344482));
#54373=CARTESIAN_POINT('Ctrl Pts',(-2.75636593218073,-1.94151094591982,
-1.25088788615355));
#54374=CARTESIAN_POINT('Ctrl Pts',(-2.64521958730332,-0.00185083012522597,
-2.30958477732822));
#54375=CARTESIAN_POINT('Ctrl Pts',(-2.53407324242588,1.93950359750643,-1.25399801226566));
#54376=CARTESIAN_POINT('Ctrl Pts',(-2.42292689754847,2.10536109037917,0.949547237585121));
#54377=CARTESIAN_POINT('Ctrl Pts',(-2.31178055267104,0.343889199955978,
2.28384008989064));
#54378=CARTESIAN_POINT('Ctrl Pts',(-2.20063420779362,-1.73239215746682,
1.52741690980612));
#54379=CARTESIAN_POINT('Ctrl Pts',(-2.08948786291619,-2.2227745514199,-0.627262917205774));
#54380=CARTESIAN_POINT('Ctrl Pts',(-1.97834151803877,-0.678342505305206,
-2.20772216536846));
#54381=CARTESIAN_POINT('Ctrl Pts',(-1.86719517316134,1.48707015493526,-1.76714625072322));
#54382=CARTESIAN_POINT('Ctrl Pts',(-1.75604882828392,2.2911619134242,0.291143034710522));
#54383=CARTESIAN_POINT('Ctrl Pts',(-1.6449024834065,0.997833321604641,2.0829105200713));
#54384=CARTESIAN_POINT('Ctrl Pts',(-1.53375613852908,-1.20894741079716,
1.96789727020159));
#54385=CARTESIAN_POINT('Ctrl Pts',(-1.42260979365165,-2.30901689786607,
0.0514010769203556));
#54386=CARTESIAN_POINT('Ctrl Pts',(-1.31146344877423,-1.29531082547211,
-1.91216236950752));
#54387=CARTESIAN_POINT('Ctrl Pts',(-1.2003171038968,0.904150711394524,-2.12523390663066));
#54388=CARTESIAN_POINT('Ctrl Pts',(-1.08917075901938,2.2759601575129,-0.392829741546613));
#54389=CARTESIAN_POINT('Ctrl Pts',(-0.978024414141959,1.56418620131702,
1.69927352442324));
#54390=CARTESIAN_POINT('Ctrl Pts',(-0.866878069264531,-0.57935041752618,
2.23562934222088));
#54391=CARTESIAN_POINT('Ctrl Pts',(-0.755731724387112,-2.19282043956138,
0.725719843207388));
#54392=CARTESIAN_POINT('Ctrl Pts',(-0.644585379509683,-1.79833929219668,
-1.44914450295862));
#54393=CARTESIAN_POINT('Ctrl Pts',(-0.533439034632267,0.241347848115584,
-2.29625613399237));
#54394=CARTESIAN_POINT('Ctrl Pts',(-0.422292689754837,2.06213591769256,
-1.04349838147448));
#54395=CARTESIAN_POINT('Ctrl Pts',(-0.311146344877418,1.99113983194757,
1.16894947486069));
#54396=CARTESIAN_POINT('Ctrl Pts',(-0.237048781625798,0.734562905288542,
1.92373973464384));
#54397=CARTESIAN_POINT('Ctrl Pts',(-0.199999999999991,0.0853826423429707,
1.9521336543348));
#54398=CARTESIAN_POINT('Ctrl Pts',(-29.7993827215147,1.05793541951253,-1.4823699524473));
#54399=CARTESIAN_POINT('Ctrl Pts',(-29.7623339398889,1.55089619265196,-1.1305544953993));
#54400=CARTESIAN_POINT('Ctrl Pts',(-29.6882363766373,2.14974771680019,0.0973963207404695));
#54401=CARTESIAN_POINT('Ctrl Pts',(-29.5770900317599,1.08185724657521,1.86262115551182));
#54402=CARTESIAN_POINT('Ctrl Pts',(-29.4659436868824,-0.977303115035886,
1.91722336588929));
#54403=CARTESIAN_POINT('Ctrl Pts',(-29.354797342005,-2.14133124400932,0.219490070886125));
#54404=CARTESIAN_POINT('Ctrl Pts',(-29.2436509971276,-1.34534920141955,
-1.68061148074165));
#54405=CARTESIAN_POINT('Ctrl Pts',(-29.1325046522502,0.682347969528367,
-2.04146153236715));
#54406=CARTESIAN_POINT('Ctrl Pts',(-29.0213583073728,2.08532885325423,-0.533874775345859));
#54407=CARTESIAN_POINT('Ctrl Pts',(-28.9102119624953,1.57935465773805,1.46265005426954));
#54408=CARTESIAN_POINT('Ctrl Pts',(-28.7990656176179,-0.372441072386024,
2.12009866279412));
#54409=CARTESIAN_POINT('Ctrl Pts',(-28.6879192727404,-1.98327983047877,
0.836784155643198));
#54410=CARTESIAN_POINT('Ctrl Pts',(-28.5767729278631,-1.77855239711682,
-1.21258534936276));
#54411=CARTESIAN_POINT('Ctrl Pts',(-28.4656265829856,0.0543337550040538,
-2.15189119828085));
#54412=CARTESIAN_POINT('Ctrl Pts',(-28.3544802381082,1.83747923218003,-1.12128059578709));
#54413=CARTESIAN_POINT('Ctrl Pts',(-28.2433338932307,1.93852558318769,0.93579822925128));
#54414=CARTESIAN_POINT('Ctrl Pts',(-28.1321875483534,0.264969893601056,
2.13620868271033));
#54415=CARTESIAN_POINT('Ctrl Pts',(-28.0210412034759,-1.6511493223133,1.38105191948624));
#54416=CARTESIAN_POINT('Ctrl Pts',(-27.9098948585985,-2.05574240249434,
-0.638374071221615));
#54417=CARTESIAN_POINT('Ctrl Pts',(-27.7987485137211,-0.578428952338934,
-2.07340729692367));
#54418=CARTESIAN_POINT('Ctrl Pts',(-27.6876021688437,1.42840080550757,-1.61036309606447));
#54419=CARTESIAN_POINT('Ctrl Pts',(-27.5764558239662,2.12761698064718,0.326870147354796));
#54420=CARTESIAN_POINT('Ctrl Pts',(-27.4653094790888,0.879129893443812,
1.96487370836676));
#54421=CARTESIAN_POINT('Ctrl Pts',(-27.3541631342114,-1.174146852909,1.80415555603761));
#54422=CARTESIAN_POINT('Ctrl Pts',(-27.243016789334,-2.15256395025648,-0.00815670731610067));
#54423=CARTESIAN_POINT('Ctrl Pts',(-27.1318704444565,-1.16044036715154,
-1.81300199677203));
#54424=CARTESIAN_POINT('Ctrl Pts',(-27.0207240995791,0.893995417007299,
-1.95815481682795));
#54425=CARTESIAN_POINT('Ctrl Pts',(-26.9095777547017,2.13003306004753,-0.310736630320814));
#54426=CARTESIAN_POINT('Ctrl Pts',(-26.7984314098243,1.4161556760299,1.62114194041067));
#54427=CARTESIAN_POINT('Ctrl Pts',(-26.6872850649468,-0.594125639310525,
2.06896418898866));
#54428=CARTESIAN_POINT('Ctrl Pts',(-26.5761387200694,-2.06052125936704,
0.622776227836984));
#54429=CARTESIAN_POINT('Ctrl Pts',(-26.464992375192,-1.64063565578329,-1.3935252904711));
#54430=CARTESIAN_POINT('Ctrl Pts',(-26.3538460303146,0.281151574973685,
-2.13413961169929));
#54431=CARTESIAN_POINT('Ctrl Pts',(-26.2426996854371,1.94556172969375,-0.921079609061524));
#54432=CARTESIAN_POINT('Ctrl Pts',(-26.1315533405598,1.82892908108006,1.13517245679029));
#54433=CARTESIAN_POINT('Ctrl Pts',(-26.0204069956823,0.03802368751086,2.15224354790078));
#54434=CARTESIAN_POINT('Ctrl Pts',(-25.9092606508049,-1.78769006704002,
1.19906726854251));
#54435=CARTESIAN_POINT('Ctrl Pts',(-25.7981143059274,-1.97688287245175,
-0.851781778914594));
#54436=CARTESIAN_POINT('Ctrl Pts',(-25.6869679610501,-0.356360283451301,
-2.12287668946283));
#54437=CARTESIAN_POINT('Ctrl Pts',(-25.5758216161726,1.59038835561325,-1.45060779282844));
#54438=CARTESIAN_POINT('Ctrl Pts',(-25.4646752712952,2.08123369845556,0.549603841596811));
#54439=CARTESIAN_POINT('Ctrl Pts',(-25.3535289264178,0.666836846147605,
2.04668676423755));
#54440=CARTESIAN_POINT('Ctrl Pts',(-25.2423825815403,-1.35800836546965,
1.67015309765288));
#54441=CARTESIAN_POINT('Ctrl Pts',(-25.1312362366629,-2.13967995310613,
-0.235303609323872));
#54442=CARTESIAN_POINT('Ctrl Pts',(-25.0200898917855,-0.962605373120884,
-1.92535424946266));
#54443=CARTESIAN_POINT('Ctrl Pts',(-24.9089435469081,1.09567556802856,-1.85286079884874));
#54444=CARTESIAN_POINT('Ctrl Pts',(-24.7977972020306,2.15093252107306,-0.084186578950635));
#54445=CARTESIAN_POINT('Ctrl Pts',(-24.6866508571532,1.23714226855362,1.76155530643892));
#54446=CARTESIAN_POINT('Ctrl Pts',(-24.5755045122758,-0.809176086504933,
1.99470101802593));
#54447=CARTESIAN_POINT('Ctrl Pts',(-24.4643581673984,-2.11474321095452,
0.401819912407123));
#54448=CARTESIAN_POINT('Ctrl Pts',(-24.3532118225209,-1.48439223048003,
-1.55890275398294));
#54449=CARTESIAN_POINT('Ctrl Pts',(-24.2420654776435,0.504829074726625,
-2.09254526727519));
#54450=CARTESIAN_POINT('Ctrl Pts',(-24.1309191327661,2.03191022949194,-0.710590535801833));
#54451=CARTESIAN_POINT('Ctrl Pts',(-24.0197727878887,1.69890180908922,1.32186638256614));
#54452=CARTESIAN_POINT('Ctrl Pts',(-23.9086264430113,-0.189347339202901,
2.14423545242165));
#54453=CARTESIAN_POINT('Ctrl Pts',(-23.7974800981338,-1.90426057598421,
1.00368807357534));
#54454=CARTESIAN_POINT('Ctrl Pts',(-23.6863337532564,-1.87593969032234,
-1.05567436672414));
#54455=CARTESIAN_POINT('Ctrl Pts',(-23.575187408379,-0.13031072137717,-2.14863147286343));
#54456=CARTESIAN_POINT('Ctrl Pts',(-23.4640410635016,1.73460974521793,-1.27464784237848));
#54457=CARTESIAN_POINT('Ctrl Pts',(-23.3528947186241,2.01160105173812,0.766197950226435));
#54458=CARTESIAN_POINT('Ctrl Pts',(-23.2417483737467,0.447094593531423,
2.10563636811299));
#54459=CARTESIAN_POINT('Ctrl Pts',(-23.1306020288693,-1.52669962772263,
1.51749343886447));
#54460=CARTESIAN_POINT('Ctrl Pts',(-23.0194556839919,-2.10289368892934,
-0.459821947438659));
#54461=CARTESIAN_POINT('Ctrl Pts',(-22.9083093391144,-0.75401715809411,
-2.01619845639877));
#54462=CARTESIAN_POINT('Ctrl Pts',(-22.797162994237,1.28511597704955,-1.72686855777071));
#54463=CARTESIAN_POINT('Ctrl Pts',(-22.6860166493596,2.1478040128497,0.143303917154594));
#54464=CARTESIAN_POINT('Ctrl Pts',(-22.5748703044822,1.04430880107363,1.88229041815689));
#54465=CARTESIAN_POINT('Ctrl Pts',(-22.4637239596048,-1.01518726445027,
1.89815513285481));
#54466=CARTESIAN_POINT('Ctrl Pts',(-22.3525776147273,-2.14534146238614,
0.176374884980863));
#54467=CARTESIAN_POINT('Ctrl Pts',(-22.2414312698499,-1.31156672712401,
-1.70686578575655));
#54468=CARTESIAN_POINT('Ctrl Pts',(-22.1302849249725,0.72286715185956,-2.02757519491819));
#54469=CARTESIAN_POINT('Ctrl Pts',(-22.0191385800951,2.09556035259399,-0.492163488000983));
#54470=CARTESIAN_POINT('Ctrl Pts',(-21.9079922352176,1.54989618230904,1.49379379913996));
#54471=CARTESIAN_POINT('Ctrl Pts',(-21.7968458903402,-0.414603175407699,
2.11227420029383));
#54472=CARTESIAN_POINT('Ctrl Pts',(-21.6856995454628,-1.99955867670109,
0.797096724817328));
#54473=CARTESIAN_POINT('Ctrl Pts',(-21.5745532005854,-1.75404047129018,
-1.24777406422847));
#54474=CARTESIAN_POINT('Ctrl Pts',(-21.4634068557079,0.0971945358346896,
-2.15038399186959));
#54475=CARTESIAN_POINT('Ctrl Pts',(-21.3522605108305,1.85945388830448,-1.08444885889306));
#54476=CARTESIAN_POINT('Ctrl Pts',(-21.2411141659531,1.91949690122385,0.974232896425261));
#54477=CARTESIAN_POINT('Ctrl Pts',(-21.1299678210757,0.222357867559114,
2.14106400395216));
#54478=CARTESIAN_POINT('Ctrl Pts',(-21.0188214761983,-1.67833619791759,
1.34788192993475));
#54479=CARTESIAN_POINT('Ctrl Pts',(-20.9076751313208,-2.04261609506057,
-0.679203635506052));
#54480=CARTESIAN_POINT('Ctrl Pts',(-20.7965287864434,-0.537005851711156,
-2.08451980213983));
#54481=CARTESIAN_POINT('Ctrl Pts',(-20.685382441566,1.46020041397922,-1.5815855466272));
#54482=CARTESIAN_POINT('Ctrl Pts',(-20.5742360966886,2.12068248374981,0.369193571723346));
#54483=CARTESIAN_POINT('Ctrl Pts',(-20.4630897518111,0.839809407505516,
1.98199854928058));
#54484=CARTESIAN_POINT('Ctrl Pts',(-20.3519434069337,-1.20985783166774,
1.78040504308355));
#54485=CARTESIAN_POINT('Ctrl Pts',(-20.2407970620563,-2.15197420198039,
-0.0510404182583582));
#54486=CARTESIAN_POINT('Ctrl Pts',(-20.1296507171789,-1.12408977155138,
-1.83576149752049));
#54487=CARTESIAN_POINT('Ctrl Pts',(-20.0185043723015,0.932830112938281,
-1.93995517233793));
#54488=CARTESIAN_POINT('Ctrl Pts',(-19.907358027424,2.13580106637051,-0.268238504275029));
#54489=CARTESIAN_POINT('Ctrl Pts',(-19.7962116825466,1.38357673581526,1.64903411316925));
#54490=CARTESIAN_POINT('Ctrl Pts',(-19.6850653376692,-0.635227498409481,
2.05671682920852));
#54491=CARTESIAN_POINT('Ctrl Pts',(-19.5739189927917,-2.07251979844461,
0.581601044823888));
#54492=CARTESIAN_POINT('Ctrl Pts',(-19.4627726479143,-1.61254694598326,
-1.42593493445009));
#54493=CARTESIAN_POINT('Ctrl Pts',(-19.3516263030369,0.323614037310276,
-2.12811466917101));
#54494=CARTESIAN_POINT('Ctrl Pts',(-19.2404799581594,1.9635261566324,-0.88213554656046));
#54495=CARTESIAN_POINT('Ctrl Pts',(-19.1293336132821,1.8059501381863,1.17138473127749));
#54496=CARTESIAN_POINT('Ctrl Pts',(-19.0181872684046,-0.00486280803173237,
2.15257391124745));
#54497=CARTESIAN_POINT('Ctrl Pts',(-18.9070409235272,-1.81122415083018,
1.16321329331064));
#54498=CARTESIAN_POINT('Ctrl Pts',(-18.7958945786497,-1.95952052975758,
-0.89099797067317));
#54499=CARTESIAN_POINT('Ctrl Pts',(-18.6847482337724,-0.313995677398985,
-2.12955507204201));
#54500=CARTESIAN_POINT('Ctrl Pts',(-18.5736018888949,1.61897301854108,-1.41863471532354));
#54501=CARTESIAN_POINT('Ctrl Pts',(-18.4624555440175,2.06987090714062,0.590958981705142));
#54502=CARTESIAN_POINT('Ctrl Pts',(-18.3513091991401,0.625928541267625,
2.05956586481513));
#54503=CARTESIAN_POINT('Ctrl Pts',(-18.2401628542627,-1.39101313211078,
1.64276612960593));
#54504=CARTESIAN_POINT('Ctrl Pts',(-18.1290165093852,-2.13456733570513,
-0.277885551308158));
#54505=CARTESIAN_POINT('Ctrl Pts',(-18.0178701645078,-0.924055660300427,
-1.94415000114493));
#54506=CARTESIAN_POINT('Ctrl Pts',(-17.9067238196304,1.13237247128039,-1.83066399881886));
#54507=CARTESIAN_POINT('Ctrl Pts',(-17.795577474753,2.15218284363935,-0.0413170404259255));
#54508=CARTESIAN_POINT('Ctrl Pts',(-17.6844311298755,1.20180141657515,1.78585314217129));
#54509=CARTESIAN_POINT('Ctrl Pts',(-17.5732847849981,-0.848755723937063,
1.97818396802956));
#54510=CARTESIAN_POINT('Ctrl Pts',(-17.4621384401207,-2.12232889584438,
0.359608326028584));
#54511=CARTESIAN_POINT('Ctrl Pts',(-17.3509920952433,-1.45303973213311,
-1.58816675041623));
#54512=CARTESIAN_POINT('Ctrl Pts',(-17.2398457503659,0.546418461103423,
-2.08207227435804));
#54513=CARTESIAN_POINT('Ctrl Pts',(-17.1286994054884,2.04566396362873,-0.66996793818504));
#54514=CARTESIAN_POINT('Ctrl Pts',(-17.017553060611,1.67222918834758,1.35545108060876));
#54515=CARTESIAN_POINT('Ctrl Pts',(-16.9064067157336,-0.232029161415369,
2.1400375133483));
#54516=CARTESIAN_POINT('Ctrl Pts',(-16.7952603708562,-1.92387900118643,
0.965550453927213));
#54517=CARTESIAN_POINT('Ctrl Pts',(-16.6841140259787,-1.85453524979851,
-1.09283900806108));
#54518=CARTESIAN_POINT('Ctrl Pts',(-16.5729676811013,-0.0874778716651755,
-2.15080117915488));
#54519=CARTESIAN_POINT('Ctrl Pts',(-16.4618213362239,1.75966014919564,-1.23983638018002));
#54520=CARTESIAN_POINT('Ctrl Pts',(-16.3506749913465,1.99593689683189,0.806122815798095));
#54521=CARTESIAN_POINT('Ctrl Pts',(-16.239528646469,0.405055455782525,2.11412586380894));
#54522=CARTESIAN_POINT('Ctrl Pts',(-16.1283823015916,-1.55662948816291,
1.48677595046018));
#54523=CARTESIAN_POINT('Ctrl Pts',(-16.0172359567142,-2.09331531487129,
-0.501626437511458));
#54524=CARTESIAN_POINT('Ctrl Pts',(-15.9060896118368,-0.713698965323934,
-2.03082049358889));
#54525=CARTESIAN_POINT('Ctrl Pts',(-15.7949432669594,1.31926514828246,-1.7009225610863));
#54526=CARTESIAN_POINT('Ctrl Pts',(-15.6837969220819,2.14452268431221,0.186065974201366));
#54527=CARTESIAN_POINT('Ctrl Pts',(-15.5726505772045,1.00660082840694,1.90272248700002));
#54528=CARTESIAN_POINT('Ctrl Pts',(-15.4615042323271,-1.05280253790118,
1.877552903775));
#54529=CARTESIAN_POINT('Ctrl Pts',(-15.3503578874497,-2.14842955374026,
0.133598438989754));
#54530=CARTESIAN_POINT('Ctrl Pts',(-15.2392115425722,-1.27730067756617,
-1.73265722789423));
#54531=CARTESIAN_POINT('Ctrl Pts',(-15.1280651976948,0.763118869136211,
-2.01277114492766));
#54532=CARTESIAN_POINT('Ctrl Pts',(-15.0169188528174,2.10494975158977,-0.450316148463807));
#54533=CARTESIAN_POINT('Ctrl Pts',(-14.90577250794,1.51982784235249,1.52437574760794));
#54534=CARTESIAN_POINT('Ctrl Pts',(-14.7946261630625,-0.456603527596969,
2.10359485378509));
#54535=CARTESIAN_POINT('Ctrl Pts',(-14.6834798181851,-2.01504228678013,
0.757101494367162));
#54536=CARTESIAN_POINT('Ctrl Pts',(-14.5723334733077,-1.72883304096769,
-1.28247199062728));
#54537=CARTESIAN_POINT('Ctrl Pts',(-14.4611871284303,0.140017145391684,
-2.14802078418285));
#54538=CARTESIAN_POINT('Ctrl Pts',(-14.3500407835528,1.88069019640931,-1.04718788926104));
#54539=CARTESIAN_POINT('Ctrl Pts',(-14.2388944386754,1.89970636628787,1.01228148860406));
#54540=CARTESIAN_POINT('Ctrl Pts',(-14.127748093798,0.179657514235822,2.14506905899641));
#54541=CARTESIAN_POINT('Ctrl Pts',(-14.0166017489206,-1.7048568070482,1.3141770648381));
#54542=CARTESIAN_POINT('Ctrl Pts',(-13.9054554040431,-2.02867896392615,
-0.719763677611344));
#54543=CARTESIAN_POINT('Ctrl Pts',(-13.7943090591657,-0.495369571687756,
-2.09480478272584));
#54544=CARTESIAN_POINT('Ctrl Pts',(-13.6831627142883,1.49142037435554,-1.55218019483637));
#54545=CARTESIAN_POINT('Ctrl Pts',(-13.5720163694109,2.11290615968028,0.411370454299073));
#54546=CARTESIAN_POINT('Ctrl Pts',(-13.4608700245335,0.800155548197115,
1.99833660552333));
#54547=CARTESIAN_POINT('Ctrl Pts',(-13.349723679656,-1.24508854262961,1.75594778148371));
#54548=CARTESIAN_POINT('Ctrl Pts',(-13.2385773347786,-2.15053020287081,
-0.0939038701307013));
#54549=CARTESIAN_POINT('Ctrl Pts',(-13.1274309899012,-1.08729295526273,
-1.85779227033627));
#54550=CARTESIAN_POINT('Ctrl Pts',(-13.0162846450238,0.971294511013014,
-1.92098544064266));
#54551=CARTESIAN_POINT('Ctrl Pts',(-12.9051383001463,2.14072124167643,-0.225633897542892));
#54552=CARTESIAN_POINT('Ctrl Pts',(-12.7939919552689,1.35044856870098,1.67627168250812));
#54553=CARTESIAN_POINT('Ctrl Pts',(-12.6828456103915,-0.676077196552766,
2.04365303184921));
#54554=CARTESIAN_POINT('Ctrl Pts',(-12.5716992655141,-2.08369562669698,
0.540194988470795));
#54555=CARTESIAN_POINT('Ctrl Pts',(-12.4605529206366,-1.583818116919,-1.45777853695418));
#54556=CARTESIAN_POINT('Ctrl Pts',(-12.3494065757592,0.365948037289866,
-2.12124494679158));
#54557=CARTESIAN_POINT('Ctrl Pts',(-12.2382602308818,1.98071113903302,-0.842841310090813));
#54558=CARTESIAN_POINT('Ctrl Pts',(-12.1271138860044,1.78225430238563,1.20713201097189));
#54559=CARTESIAN_POINT('Ctrl Pts',(-12.0159675411269,-0.0477473732258512,
2.15204978535236));
#54560=CARTESIAN_POINT('Ctrl Pts',(-11.9048211962495,-1.83403924813354,
1.12689756703564));
#54561=CARTESIAN_POINT('Ctrl Pts',(-11.7936748513721,-1.94138033260439,
-0.929860470426608));
#54562=CARTESIAN_POINT('Ctrl Pts',(-11.6825285064947,-0.271506427111522,
-2.13538810297384));
#54563=CARTESIAN_POINT('Ctrl Pts',(-11.5713821616172,1.64691501130435,-1.38609849427286));
#54564=CARTESIAN_POINT('Ctrl Pts',(-11.4602358167399,2.05768645650133,0.63207953377416));
#54565=CARTESIAN_POINT('Ctrl Pts',(-11.3490894718624,0.584771766775093,
2.07162739677478));
#54566=CARTESIAN_POINT('Ctrl Pts',(-11.237943126985,-1.42346571991491,1.61472704644229));
#54567=CARTESIAN_POINT('Ctrl Pts',(-11.1267967821076,-2.12860737698019,
-0.320357183391695));
#54568=CARTESIAN_POINT('Ctrl Pts',(-11.0156504372302,-0.885139132841,-1.96217399987834));
#54569=CARTESIAN_POINT('Ctrl Pts',(-10.9045040923527,1.16861986611292,-1.80774049542829));
#54570=CARTESIAN_POINT('Ctrl Pts',(-10.7933577474753,2.15257883220101,0.00156889937841303));
#54571=CARTESIAN_POINT('Ctrl Pts',(-10.6822114025979,1.16598349555022,1.80944206273359));
#54572=CARTESIAN_POINT('Ctrl Pts',(-10.5710650577204,-0.887998437915542,
1.96088165490543));
#54573=CARTESIAN_POINT('Ctrl Pts',(-10.459918712843,-2.12907209760132,0.317253988943611));
#54574=CARTESIAN_POINT('Ctrl Pts',(-10.3487723679656,-1.42111043276905,
-1.61680030559128));
#54575=CARTESIAN_POINT('Ctrl Pts',(-10.2376260230881,0.587790940318532,
-2.07077277864196));
#54576=CARTESIAN_POINT('Ctrl Pts',(-10.1264796782108,2.05860564766888,-0.629079389005017));
#54577=CARTESIAN_POINT('Ctrl Pts',(-10.0153333333333,1.64489275678552,1.38849771658423));
#54578=CARTESIAN_POINT('Ctrl Pts',(-9.90418698845591,-0.27461887695429,
2.1349900615004));
#54579=CARTESIAN_POINT('Ctrl Pts',(-9.79304064357848,-1.94273372024891,
0.927029547799284));
#54580=CARTESIAN_POINT('Ctrl Pts',(-9.68189429870106,-1.83239462994335,
-1.12956983424659));
#54581=CARTESIAN_POINT('Ctrl Pts',(-9.57074795382363,-0.0446102965948741,
-2.1521170999095));
#54582=CARTESIAN_POINT('Ctrl Pts',(-9.45960160894622,1.78401203561639,-1.20453275051405));
#54583=CARTESIAN_POINT('Ctrl Pts',(-9.34845526406878,1.97948043156636,0.845727681544679));
#54584=CARTESIAN_POINT('Ctrl Pts',(-9.23730891919137,0.362855526560633,
2.12177613266092));
#54585=CARTESIAN_POINT('Ctrl Pts',(-9.12616257431394,-1.5859414264279,1.45546826905465));
#54586=CARTESIAN_POINT('Ctrl Pts',(-9.01501622943652,-2.08290597495865,
-0.543231801137112));
#54587=CARTESIAN_POINT('Ctrl Pts',(-8.90386988455909,-0.673097461450849,
-2.0446363729704));
#54588=CARTESIAN_POINT('Ctrl Pts',(-8.79272353968167,1.35289062187478,-1.67430136341352));
#54589=CARTESIAN_POINT('Ctrl Pts',(-8.68157719480423,2.14039006255939,0.228754170196138));
#54590=CARTESIAN_POINT('Ctrl Pts',(-8.57043084992684,0.968493273837022,
1.92239924802773));
#54591=CARTESIAN_POINT('Ctrl Pts',(-8.45928450504939,-1.089999889143,1.8562053582385));
#54592=CARTESIAN_POINT('Ctrl Pts',(-8.34813816017197,-2.15066480100183,
0.0907689595448498));
#54593=CARTESIAN_POINT('Ctrl Pts',(-8.23699181529456,-1.24252758865235,
-1.75776087159856));
#54594=CARTESIAN_POINT('Ctrl Pts',(-8.12584547041711,0.803067657504474,
-1.99716810202731));
#54595=CARTESIAN_POINT('Ctrl Pts',(-8.01469912553972,2.11350356630602,-0.408290050695375));
#54596=CARTESIAN_POINT('Ctrl Pts',(-7.90355278066228,1.48915618906188,1.55435257739802));
#54597=CARTESIAN_POINT('Ctrl Pts',(-7.79240643578487,-0.498422625706736,
2.09408046083924));
#54598=CARTESIAN_POINT('Ctrl Pts',(-7.68126009090743,-2.02972600239322,
0.71680572367549));
#54599=CARTESIAN_POINT('Ctrl Pts',(-7.57011374603002,-1.7029393302673,-1.3166608248573));
#54600=CARTESIAN_POINT('Ctrl Pts',(-7.45896740115258,0.182784173514752,
-2.14480489466936));
#54601=CARTESIAN_POINT('Ctrl Pts',(-7.34782105627517,1.90117994267266,-1.00951122622003));
#54602=CARTESIAN_POINT('Ctrl Pts',(-7.23667471139775,1.87916172082065,1.04992824387551));
#54603=CARTESIAN_POINT('Ctrl Pts',(-7.12552836652031,0.136885843773243,
2.14822260393554));
#54604=CARTESIAN_POINT('Ctrl Pts',(-7.0143820216429,-1.73070065344576,1.27995052187477));
#54605=CARTESIAN_POINT('Ctrl Pts',(-6.90323567676547,-2.01393652508823,
-0.760038001155664));
#54606=CARTESIAN_POINT('Ctrl Pts',(-6.79208933188806,-0.453536648952868,
-2.10425820619564));
#54607=CARTESIAN_POINT('Ctrl Pts',(-6.68094298701061,1.52204829807255,-1.52215868706898));
#54608=CARTESIAN_POINT('Ctrl Pts',(-6.56979664213322,2.10429109294252,0.45338403858971));
#54609=CARTESIAN_POINT('Ctrl Pts',(-6.45865029725577,0.760184057839905,
2.01388139881452));
#54610=CARTESIAN_POINT('Ctrl Pts',(-6.34750395237836,-1.27982500121702,
1.73079347599445));
#54611=CARTESIAN_POINT('Ctrl Pts',(-6.23635760750093,-2.14823252579159,
-0.136730045769932));
#54612=CARTESIAN_POINT('Ctrl Pts',(-6.12521126262351,-1.05006452539279,
-1.87908557090855));
#54613=CARTESIAN_POINT('Ctrl Pts',(-6.01406491774608,1.00937334243772,-1.90125315144018));
#54614=CARTESIAN_POINT('Ctrl Pts',(-5.90291857286866,2.14479163279392,-0.182939722811514));
#54615=CARTESIAN_POINT('Ctrl Pts',(-5.79177222799124,1.31678432532478,1.7028438363115));
#54616=CARTESIAN_POINT('Ctrl Pts',(-5.6806258831138,-0.716658517991673,
2.02977798265601));
#54617=CARTESIAN_POINT('Ctrl Pts',(-5.5694795382364,-2.09404430774185,0.498574495435823));
#54618=CARTESIAN_POINT('Ctrl Pts',(-5.45833319335896,-1.55446057283712,
-1.48904345731747));
#54619=CARTESIAN_POINT('Ctrl Pts',(-5.34718684848155,0.408136769940926,
-2.1135331715654));
#54620=CARTESIAN_POINT('Ctrl Pts',(-5.23604050360411,1.99710985511599,-0.803212497962859));
#54621=CARTESIAN_POINT('Ctrl Pts',(-5.1248941587267,1.75785098001617,1.24240010557842));
#54622=CARTESIAN_POINT('Ctrl Pts',(-5.01374781384926,-0.0906129845449661,
2.15067137827167));
#54623=CARTESIAN_POINT('Ctrl Pts',(-4.90260146897186,-1.85612630223178,
1.09013450566824));
#54624=CARTESIAN_POINT('Ctrl Pts',(-4.79145512409441,-1.92246948195445,
-0.968353851254212));
#54625=CARTESIAN_POINT('Ctrl Pts',(-4.68030877921701,-0.228909399190852,
-2.14037346676862));
#54626=CARTESIAN_POINT('Ctrl Pts',(-4.56916243433958,1.67420324200416,-1.35301204530782));
#54627=CARTESIAN_POINT('Ctrl Pts',(-4.45801608946216,2.04468518329698,0.672949174522688));
#54628=CARTESIAN_POINT('Ctrl Pts',(-4.34686974458473,0.543382860330313,
2.082866572151));
#54629=CARTESIAN_POINT('Ctrl Pts',(-4.23572339970731,-1.4553532464501,1.58604697860226));
#54630=CARTESIAN_POINT('Ctrl Pts',(-4.12457705482988,-2.1218024428059,-0.362701645966607));
#54631=CARTESIAN_POINT('Ctrl Pts',(-4.01343070995247,-0.845871239111339,
-1.97941909082634));
#54632=CARTESIAN_POINT('Ctrl Pts',(-3.90228436507503,1.20440336370244,-1.78409938842956));
#54633=CARTESIAN_POINT('Ctrl Pts',(-3.79113802019762,2.15212032956352,0.0444542163922969));
#54634=CARTESIAN_POINT('Ctrl Pts',(-3.67999167532019,1.12970272382336,1.8323127042249));
#54635=CARTESIAN_POINT('Ctrl Pts',(-3.56884533044277,-0.926888650596847,
1.94280094701669));
#54636=CARTESIAN_POINT('Ctrl Pts',(-3.45769898556534,-2.13497013941755,
0.274773714182162));
#54637=CARTESIAN_POINT('Ctrl Pts',(-3.34655264068793,-1.3886170071239,-1.64479205305372));
#54638=CARTESIAN_POINT('Ctrl Pts',(-3.23540629581049,0.628930089141089,
-2.05865126565347));
#54639=CARTESIAN_POINT('Ctrl Pts',(-3.12425995093308,2.07073014415415,-0.587941119332112));
#54640=CARTESIAN_POINT('Ctrl Pts',(-3.01311360605564,1.61690336611955,1.42099317202789));
#54641=CARTESIAN_POINT('Ctrl Pts',(-2.90196726117823,-0.317099579721297,
2.12909510093774));
#54642=CARTESIAN_POINT('Ctrl Pts',(-2.7908209163008,-1.96081724784028,0.888140645723541));
#54643=CARTESIAN_POINT('Ctrl Pts',(-2.67967457142338,-1.80952662112472,
-1.16585226305009));
#54644=CARTESIAN_POINT('Ctrl Pts',(-2.56852822654596,-0.00172501030186185,
-2.15257871561459));
#54645=CARTESIAN_POINT('Ctrl Pts',(-2.45738188166853,1.80765573268103,-1.16875096213131));
#54646=CARTESIAN_POINT('Ctrl Pts',(-2.34623553679111,1.96223819810419,0.8849968155145));
#54647=CARTESIAN_POINT('Ctrl Pts',(-2.23508919191368,0.320511539399493,
2.12858415747483));
#54648=CARTESIAN_POINT('Ctrl Pts',(-2.12394284703626,-1.61462377214598,
1.42358278518015));
#54649=CARTESIAN_POINT('Ctrl Pts',(-2.01279650215883,-2.07166986722666,
-0.584621451407953));
#54650=CARTESIAN_POINT('Ctrl Pts',(-1.90165015728142,-0.632228638303536,
-2.05764074556303));
#54651=CARTESIAN_POINT('Ctrl Pts',(-1.79050381240399,1.38597881123994,-1.64701527479129));
#54652=CARTESIAN_POINT('Ctrl Pts',(-1.67935746752657,2.1354082418958,0.271351069624803));
#54653=CARTESIAN_POINT('Ctrl Pts',(-1.56821112264915,0.930000401328434,
1.94131382231481));
#54654=CARTESIAN_POINT('Ctrl Pts',(-1.45706477777172,-1.12676291008018,
1.83411919750027));
#54655=CARTESIAN_POINT('Ctrl Pts',(-1.3459184328943,-2.1520494407184,0.0479068208384009));
#54656=CARTESIAN_POINT('Ctrl Pts',(-1.23477208801687,-1.207255321557,-1.78217316714502));
#54657=CARTESIAN_POINT('Ctrl Pts',(-1.12362574313945,0.842686354777153,
-1.98076005610316));
#54658=CARTESIAN_POINT('Ctrl Pts',(-1.01247939826203,2.12123990456699,-0.36612509262031));
#54659=CARTESIAN_POINT('Ctrl Pts',(-0.901333053384604,1.45785249247625,
1.58375655078235));
#54660=CARTESIAN_POINT('Ctrl Pts',(-0.790186708507176,-0.539966053591598,
2.0836507866298));
#54661=CARTESIAN_POINT('Ctrl Pts',(-0.679040363629756,-2.04375204222851,
0.67638525475331));
#54662=CARTESIAN_POINT('Ctrl Pts',(-0.567894018752329,-1.67608780670706,
-1.35063135310715));
#54663=CARTESIAN_POINT('Ctrl Pts',(-0.456747673874911,0.224940970347859,
-2.14015615627215));
#54664=CARTESIAN_POINT('Ctrl Pts',(-0.345601328997483,1.92195148180026,
-0.9725611407687));
#54665=CARTESIAN_POINT('Ctrl Pts',(-0.234454984120063,1.85578172498221,
1.08948404228951));
#54666=CARTESIAN_POINT('Ctrl Pts',(-0.160357420868444,0.684627163603588,
1.79296350055041));
#54667=CARTESIAN_POINT('Ctrl Pts',(-0.123308639242636,0.0795783122553931,
1.81942719557457));
#54668=CARTESIAN_POINT('Ctrl Pts',(-29.7226913607573,0.98077109908131,-1.37424797458511));
#54669=CARTESIAN_POINT('Ctrl Pts',(-29.6856425791315,1.43777600728141,-1.04809344178598));
#54670=CARTESIAN_POINT('Ctrl Pts',(-29.6115450158799,1.99294814415539,0.0902923701931233));
#54671=CARTESIAN_POINT('Ctrl Pts',(-29.5003986710025,1.00294810174865,1.72676419011022));
#54672=CARTESIAN_POINT('Ctrl Pts',(-29.389252326125,-0.906020001401381,
1.77738379211666));
#54673=CARTESIAN_POINT('Ctrl Pts',(-29.2781059812477,-1.98514555704351,
0.203480774053002));
#54674=CARTESIAN_POINT('Ctrl Pts',(-29.1669596363702,-1.24722132427754,
-1.55803004483504));
#54675=CARTESIAN_POINT('Ctrl Pts',(-29.0558132914928,0.632578469051131,
-1.89256020159966));
#54676=CARTESIAN_POINT('Ctrl Pts',(-28.9446669466154,1.93322790184544,-0.494934700673032));
#54677=CARTESIAN_POINT('Ctrl Pts',(-28.8335206017379,1.46415875198014,1.35596641802415));
#54678=CARTESIAN_POINT('Ctrl Pts',(-28.7223742568606,-0.345275744785372,
1.96546165041682));
#54679=CARTESIAN_POINT('Ctrl Pts',(-28.6112279119831,-1.83862219115491,
0.775750297123293));
#54680=CARTESIAN_POINT('Ctrl Pts',(-28.5000815671057,-1.64882728862394,
-1.12414108072153));
#54681=CARTESIAN_POINT('Ctrl Pts',(-28.3889352222282,0.0503707273899882,
-1.99493528311385));
#54682=CARTESIAN_POINT('Ctrl Pts',(-28.2777888773509,1.70345608327842,-1.03949596735827));
#54683=CARTESIAN_POINT('Ctrl Pts',(-28.1666425324734,1.79713225566867,0.867542423566838));
#54684=CARTESIAN_POINT('Ctrl Pts',(-28.055496187596,0.245643362512984,1.98039662815554));
#54685=CARTESIAN_POINT('Ctrl Pts',(-27.9443498427186,-1.5307168147738,1.28031993634082));
#54686=CARTESIAN_POINT('Ctrl Pts',(-27.8332034978412,-1.90579944516041,
-0.591811964992614));
#54687=CARTESIAN_POINT('Ctrl Pts',(-27.7220571529637,-0.536239158707246,
-1.92217588705377));
#54688=CARTESIAN_POINT('Ctrl Pts',(-27.6109108080863,1.32421526126029,-1.4929054784601));
#54689=CARTESIAN_POINT('Ctrl Pts',(-27.4997644632089,1.97243159274787,0.30302869888381));
#54690=CARTESIAN_POINT('Ctrl Pts',(-27.3886181183314,0.815007396411317,
1.82155858568272));
#54691=CARTESIAN_POINT('Ctrl Pts',(-27.277471773454,-1.08850623409605,1.67256298917007));
#54692=CARTESIAN_POINT('Ctrl Pts',(-27.1663254285766,-1.99555896550728,
-0.00756176856515067));
#54693=CARTESIAN_POINT('Ctrl Pts',(-27.0551790836992,-1.07579948011766,
-1.68076418296882));
#54694=CARTESIAN_POINT('Ctrl Pts',(-26.9440327388218,0.828788649609528,
-1.8153297606358));
#54695=CARTESIAN_POINT('Ctrl Pts',(-26.8328863939443,1.97467144671743,-0.288071937874124));
#54696=CARTESIAN_POINT('Ctrl Pts',(-26.721740049067,1.31286327429152,1.50289812907108));
#54697=CARTESIAN_POINT('Ctrl Pts',(-26.6105937041895,-0.550790951424447,
1.9180568531578));
#54698=CARTESIAN_POINT('Ctrl Pts',(-26.4994473593121,-1.91022973893913,
0.577351806350263));
#54699=CARTESIAN_POINT('Ctrl Pts',(-26.3883010144347,-1.52097000028234,
-1.2918835172025));
#54700=CARTESIAN_POINT('Ctrl Pts',(-26.2771546695572,0.260644774822252,
-1.9784784722718));
#54701=CARTESIAN_POINT('Ctrl Pts',(-26.1660083246798,1.80365519555206,-0.853897358817045));
#54702=CARTESIAN_POINT('Ctrl Pts',(-26.0548619798023,1.69552956816522,1.0523745755729));
#54703=CARTESIAN_POINT('Ctrl Pts',(-25.943715634925,0.0352502932630832,
1.99526193284844));
#54704=CARTESIAN_POINT('Ctrl Pts',(-25.8325692900475,-1.65729846976434,
1.1116089896894));
#54705=CARTESIAN_POINT('Ctrl Pts',(-25.7214229451701,-1.83269181824256,
-0.789654014862648));
#54706=CARTESIAN_POINT('Ctrl Pts',(-25.6102766002927,-0.330367865961598,
-1.96803705173043));
#54707=CARTESIAN_POINT('Ctrl Pts',(-25.4991302554152,1.47438766746241,-1.3448025021829));
#54708=CARTESIAN_POINT('Ctrl Pts',(-25.3879839105379,1.9294314418738,0.509516510970531));
#54709=CARTESIAN_POINT('Ctrl Pts',(-25.2768375656604,0.618198705177624,
1.89740431241202));
#54710=CARTESIAN_POINT('Ctrl Pts',(-25.165691220783,-1.25895714671978,1.54833448148843));
#54711=CARTESIAN_POINT('Ctrl Pts',(-25.0545448759056,-1.98361470897458,
-0.218140895254885));
#54712=CARTESIAN_POINT('Ctrl Pts',(-24.9433985310281,-0.892394292094368,
-1.78492162048654));
#54713=CARTESIAN_POINT('Ctrl Pts',(-24.8322521861507,1.01575853428468,-1.71771574012429));
#54714=CARTESIAN_POINT('Ctrl Pts',(-24.7211058412733,1.99404653047223,-0.0780461283765578));
#54715=CARTESIAN_POINT('Ctrl Pts',(-24.6099594963959,1.14690685279113,1.63306994181622));
#54716=CARTESIAN_POINT('Ctrl Pts',(-24.4988131515184,-0.750155921688874,
1.84921033335801));
#54717=CARTESIAN_POINT('Ctrl Pts',(-24.387666806641,-1.96049681769646,0.372511733566841));
#54718=CARTESIAN_POINT('Ctrl Pts',(-24.2765204617636,-1.37612275050455,
-1.44519858129832));
#54719=CARTESIAN_POINT('Ctrl Pts',(-24.1653741168862,0.468007552574359,
-1.93991796078501));
#54720=CARTESIAN_POINT('Ctrl Pts',(-24.0542277720088,1.88370555731245,-0.658761062292782));
#54721=CARTESIAN_POINT('Ctrl Pts',(-23.9430814271313,1.57498630237707,1.22545130917859));
#54722=CARTESIAN_POINT('Ctrl Pts',(-23.8319350822539,-0.175536610792046,
1.98783793658199));
#54723=CARTESIAN_POINT('Ctrl Pts',(-23.7207887373765,-1.76536648986179,
0.930480478202514));
#54724=CARTESIAN_POINT('Ctrl Pts',(-23.609642392499,-1.73911128973787,-0.978674964300812));
#54725=CARTESIAN_POINT('Ctrl Pts',(-23.4984960476217,-0.120806040775277,
-1.99191331748023));
#54726=CARTESIAN_POINT('Ctrl Pts',(-23.3873497027442,1.6080897519042,-1.18167682285115));
#54727=CARTESIAN_POINT('Ctrl Pts',(-23.2762033578668,1.86487770239841,0.710312550177829));
#54728=CARTESIAN_POINT('Ctrl Pts',(-23.1650570129894,0.414484143175073,
1.9520542151537));
#54729=CARTESIAN_POINT('Ctrl Pts',(-23.053910668112,-1.4153443057408,1.40680960334012));
#54730=CARTESIAN_POINT('Ctrl Pts',(-22.9427643232345,-1.94951158312934,
-0.426283181802225));
#54731=CARTESIAN_POINT('Ctrl Pts',(-22.8316179783571,-0.699020207879015,
-1.86913977883402));
#54732=CARTESIAN_POINT('Ctrl Pts',(-22.7204716334796,1.19138142651335,-1.60091319577356));
#54733=CARTESIAN_POINT('Ctrl Pts',(-22.6093252886023,1.99114621123524,0.132851531140779));
#54734=CARTESIAN_POINT('Ctrl Pts',(-22.4981789437248,0.968138387011664,
1.7449988044229));
#54735=CARTESIAN_POINT('Ctrl Pts',(-22.3870325988474,-0.941140934280283,
1.75970636916075));
#54736=CARTESIAN_POINT('Ctrl Pts',(-22.27588625397,-1.98886327573639,0.163510349122069));
#54737=CARTESIAN_POINT('Ctrl Pts',(-22.1647399090925,-1.21590289610751,
-1.58236939779569));
#54738=CARTESIAN_POINT('Ctrl Pts',(-22.0535935642152,0.670142239254753,
-1.87968671405889));
#54739=CARTESIAN_POINT('Ctrl Pts',(-21.9424472193377,1.94271313002443,-0.456265775917509));
#54740=CARTESIAN_POINT('Ctrl Pts',(-21.8313008744603,1.43684893628544,1.38483858197925));
#54741=CARTESIAN_POINT('Ctrl Pts',(-21.7201545295828,-0.384362603356758,
1.95820789319819));
#54742=CARTESIAN_POINT('Ctrl Pts',(-21.6090081847055,-1.85371368124662,
0.738957611640905));
#54743=CARTESIAN_POINT('Ctrl Pts',(-21.497861839828,-1.62610322816601,-1.15676318025385));
#54744=CARTESIAN_POINT('Ctrl Pts',(-21.3867154949506,0.0901053031943518,
-1.9935380102168));
#54745=CARTESIAN_POINT('Ctrl Pts',(-21.2755691500732,1.72382793891499,-1.00535068551179));
#54746=CARTESIAN_POINT('Ctrl Pts',(-21.1644228051957,1.77949149898398,0.903173720214814));
#54747=CARTESIAN_POINT('Ctrl Pts',(-21.0532764603183,0.206139397673152,
1.98489780909996));
#54748=CARTESIAN_POINT('Ctrl Pts',(-20.9421301154409,-1.55592071793766,
1.24956931913971));
#54749=CARTESIAN_POINT('Ctrl Pts',(-20.8309837705635,-1.89363055211529,
-0.62966347832668));
#54750=CARTESIAN_POINT('Ctrl Pts',(-20.719837425686,-0.497837400735304,
-1.93247786178057));
#54751=CARTESIAN_POINT('Ctrl Pts',(-20.6086910808086,1.35369545104868,-1.46622692297373));
#54752=CARTESIAN_POINT('Ctrl Pts',(-20.4975447359312,1.96600288829374,0.342265112250096));
#54753=CARTESIAN_POINT('Ctrl Pts',(-20.3863983910538,0.778554891372885,
1.83743436480388));
#54754=CARTESIAN_POINT('Ctrl Pts',(-20.2752520461764,-1.12161250432815,
1.6505448052015));
#54755=CARTESIAN_POINT('Ctrl Pts',(-20.1641057012989,-1.99501223264037,
-0.0473176019910748));
#54756=CARTESIAN_POINT('Ctrl Pts',(-20.0529593564215,-1.04210024579629,
-1.7018636377672));
#54757=CARTESIAN_POINT('Ctrl Pts',(-19.9418130115441,0.86479079748002,-1.79845757259847));
#54758=CARTESIAN_POINT('Ctrl Pts',(-19.8306666666667,1.98001874277781,-0.248673565325042));
#54759=CARTESIAN_POINT('Ctrl Pts',(-19.7195203217893,1.28266059612054,1.52875588600751));
#54760=CARTESIAN_POINT('Ctrl Pts',(-19.6083739769118,-0.588894898772527,
1.90670279856159));
#54761=CARTESIAN_POINT('Ctrl Pts',(-19.4972276320344,-1.9213531214646,0.539179883231139));
#54762=CARTESIAN_POINT('Ctrl Pts',(-19.386081287157,-1.49493004143963,-1.32192924736697));
#54763=CARTESIAN_POINT('Ctrl Pts',(-19.2749349422796,0.300010084922888,
-1.97289298057129));
#54764=CARTESIAN_POINT('Ctrl Pts',(-19.1637885974021,1.82030932247515,-0.81779382142016));
#54765=CARTESIAN_POINT('Ctrl Pts',(-19.0526422525247,1.67422667702274,1.08594557772859));
#54766=CARTESIAN_POINT('Ctrl Pts',(-18.9414959076473,-0.00450812165834452,
1.9955681999576));
#54767=CARTESIAN_POINT('Ctrl Pts',(-18.8303495627698,-1.67911601060762,
1.07837015294568));
#54768=CARTESIAN_POINT('Ctrl Pts',(-18.7192032178924,-1.81659586038661,
-0.826009832792037));
#54769=CARTESIAN_POINT('Ctrl Pts',(-18.608056873015,-0.291093274645596,
-1.97422832248426));
#54770=CARTESIAN_POINT('Ctrl Pts',(-18.4969105281376,1.50088740530984,-1.31516149594839));
#54771=CARTESIAN_POINT('Ctrl Pts',(-18.3857641832602,1.91889743656399,0.547855265367661));
#54772=CARTESIAN_POINT('Ctrl Pts',(-18.2746178383827,0.580274194476223,
1.9093440295211));
#54773=CARTESIAN_POINT('Ctrl Pts',(-18.1634714935053,-1.28955459213706,
1.52294508034306));
#54774=CARTESIAN_POINT('Ctrl Pts',(-18.0523251486279,-1.97887499869068,
-0.257616970325887));
#54775=CARTESIAN_POINT('Ctrl Pts',(-17.9411788037505,-0.856656341067444,
-1.80234643649655));
#54776=CARTESIAN_POINT('Ctrl Pts',(-17.830032458873,1.04977881706505,-1.69713794344609));
#54777=CARTESIAN_POINT('Ctrl Pts',(-17.7188861139956,1.9952056562704,-0.0383034336519918));
#54778=CARTESIAN_POINT('Ctrl Pts',(-17.6077397691182,1.11414371281292,1.65559552761003));
#54779=CARTESIAN_POINT('Ctrl Pts',(-17.4965934242408,-0.786848676075942,
1.83389801374025));
#54780=CARTESIAN_POINT('Ctrl Pts',(-17.3854470793633,-1.96752921340748,
0.333379000884986));
#54781=CARTESIAN_POINT('Ctrl Pts',(-17.2743007344859,-1.3470570592577,-1.4723281030215));
#54782=CARTESIAN_POINT('Ctrl Pts',(-17.1631543896085,0.506563467646839,
-1.93020885323027));
#54783=CARTESIAN_POINT('Ctrl Pts',(-17.0520080447311,1.89645611344,-0.621101419768934));
#54784=CARTESIAN_POINT('Ctrl Pts',(-16.9408616998537,1.55025914505001,1.25658638661721));
#54785=CARTESIAN_POINT('Ctrl Pts',(-16.8297153549762,-0.215105280967968,
1.98394618927596));
#54786=CARTESIAN_POINT('Ctrl Pts',(-16.7185690100988,-1.78355397474313,
0.895124562851952));
#54787=CARTESIAN_POINT('Ctrl Pts',(-16.6074226652214,-1.71926805897861,
-1.01312886900871));
#54788=CARTESIAN_POINT('Ctrl Pts',(-16.496276320344,-0.0810973588330665,
-1.9939247684487));
#54789=CARTESIAN_POINT('Ctrl Pts',(-16.3851299754665,1.63131301467479,-1.14940445970753));
#54790=CARTESIAN_POINT('Ctrl Pts',(-16.2739836305891,1.85035606890338,0.747325352249846));
#54791=CARTESIAN_POINT('Ctrl Pts',(-16.1628372857117,0.375511280962539,
1.95992449898274));
#54792=CARTESIAN_POINT('Ctrl Pts',(-16.0516909408343,-1.44309112428753,
1.37833260530449));
#54793=CARTESIAN_POINT('Ctrl Pts',(-15.9405445959568,-1.94063184219332,
-0.465038511209882));
#54794=CARTESIAN_POINT('Ctrl Pts',(-15.8293982510794,-0.661642767340725,
-1.88269530521234));
#54795=CARTESIAN_POINT('Ctrl Pts',(-15.718251906202,1.22303980526226,-1.57685966356773));
#54796=CARTESIAN_POINT('Ctrl Pts',(-15.6071055613246,1.98810421818273,0.172494583935125));
#54797=CARTESIAN_POINT('Ctrl Pts',(-15.4959592164471,0.933180780796459,
1.76394058692321));
#54798=CARTESIAN_POINT('Ctrl Pts',(-15.3848128715697,-0.976012602630028,
1.74060683767192));
#54799=CARTESIAN_POINT('Ctrl Pts',(-15.2736665266923,-1.9917261260537,0.123853956892735));
#54800=CARTESIAN_POINT('Ctrl Pts',(-15.1625201818149,-1.18413616397418,
-1.60627964844588));
#54801=CARTESIAN_POINT('Ctrl Pts',(-15.0513738369374,0.707458052928451,
-1.86596245063764));
#54802=CARTESIAN_POINT('Ctrl Pts',(-14.94022749206,1.95141767947325,-0.417470722425096));
#54803=CARTESIAN_POINT('Ctrl Pts',(-14.8290811471826,1.40897373872346,1.41318992617077));
#54804=CARTESIAN_POINT('Ctrl Pts',(-14.7179348023052,-0.423299508973792,
1.95016160600743));
#54805=CARTESIAN_POINT('Ctrl Pts',(-14.6067884574277,-1.86806793860003,
0.70187957700558));
#54806=CARTESIAN_POINT('Ctrl Pts',(-14.4956421125503,-1.60273439233121,
-1.18893028873925));
#54807=CARTESIAN_POINT('Ctrl Pts',(-14.3844957676729,0.129804491884053,
-1.99134717157247));
#54808=CARTESIAN_POINT('Ctrl Pts',(-14.2733494227955,1.74351530059724,-0.970807478559067));
#54809=CARTESIAN_POINT('Ctrl Pts',(-14.1622030779181,1.7611444578106,0.938447101634346));
#54810=CARTESIAN_POINT('Ctrl Pts',(-14.0510567330406,0.166553548019546,
1.98861074106649));
#54811=CARTESIAN_POINT('Ctrl Pts',(-13.9399103881632,-1.58050695116664,
1.21832283946285));
#54812=CARTESIAN_POINT('Ctrl Pts',(-13.8287640432858,-1.88070997570899,
-0.667265128049994));
#54813=CARTESIAN_POINT('Ctrl Pts',(-13.7176176984084,-0.459238012372806,
-1.94201267035898));
#54814=CARTESIAN_POINT('Ctrl Pts',(-13.606471353531,1.38263827145797,-1.43896635615383));
#54815=CARTESIAN_POINT('Ctrl Pts',(-13.4953250086535,1.95879375835649,0.381365672375669));
#54816=CARTESIAN_POINT('Ctrl Pts',(-13.3841786637761,0.741793328748737,
1.85258074622047));
#54817=CARTESIAN_POINT('Ctrl Pts',(-13.2730323188987,-1.15427353682048,
1.6278714218386));
#54818=CARTESIAN_POINT('Ctrl Pts',(-13.1618859740213,-1.99367355679339,
-0.0870546540151287));
#54819=CARTESIAN_POINT('Ctrl Pts',(-13.0507396291438,-1.00798733749538,
-1.72228751702261));
#54820=CARTESIAN_POINT('Ctrl Pts',(-12.9395932842664,0.900449656498692,
-1.78087146643273));
#54821=CARTESIAN_POINT('Ctrl Pts',(-12.828446939389,1.98458004742218,-0.209176478640999));
#54822=CARTESIAN_POINT('Ctrl Pts',(-12.7173005945116,1.25194875088693,1.5540067853763));
#54823=CARTESIAN_POINT('Ctrl Pts',(-12.6061542496341,-0.626765077430113,
1.89459185619408));
#54824=CARTESIAN_POINT('Ctrl Pts',(-12.4950079047567,-1.93171380053448,
0.500793926348479));
#54825=CARTESIAN_POINT('Ctrl Pts',(-12.3838615598793,-1.46829665273085,
-1.35145022232501));
#54826=CARTESIAN_POINT('Ctrl Pts',(-12.2727152150019,0.33925630253003,-1.96652432607292));
#54827=CARTESIAN_POINT('Ctrl Pts',(-12.1615688701244,1.83624085644772,-0.781365651251085));
#54828=CARTESIAN_POINT('Ctrl Pts',(-12.050422525247,1.65225918213296,1.1190855011572));
#54829=CARTESIAN_POINT('Ctrl Pts',(-11.9392761803696,-0.0442647470282004,
1.99508230306758));
#54830=CARTESIAN_POINT('Ctrl Pts',(-11.8281298354922,-1.70026700682643,
1.04470324462997));
#54831=CARTESIAN_POINT('Ctrl Pts',(-11.7169834906148,-1.79977878368105,
-0.862037756513309));
#54832=CARTESIAN_POINT('Ctrl Pts',(-11.6058371457373,-0.251703130469517,
-1.97963590035004));
#54833=CARTESIAN_POINT('Ctrl Pts',(-11.4946908008599,1.52679134844995,-1.28499842106567));
#54834=CARTESIAN_POINT('Ctrl Pts',(-11.3835444559825,1.90760170260443,0.585976542246873));
#54835=CARTESIAN_POINT('Ctrl Pts',(-11.272398111105,0.542119337186086,1.92052581031649));
#54836=CARTESIAN_POINT('Ctrl Pts',(-11.1612517662276,-1.31964013386451,
1.49695112843972));
#54837=CARTESIAN_POINT('Ctrl Pts',(-11.0501054213502,-1.97334975096636,
-0.296990781345034));
#54838=CARTESIAN_POINT('Ctrl Pts',(-10.9389590764728,-0.820578330345012,
-1.81905579013154));
#54839=CARTESIAN_POINT('Ctrl Pts',(-10.8278127315954,1.08338237793752,-1.67588644812748));
#54840=CARTESIAN_POINT('Ctrl Pts',(-10.7166663867179,1.99557276198374,0.00145446606594789));
#54841=CARTESIAN_POINT('Ctrl Pts',(-10.6055200418405,1.08093830053302,1.67746390550846));
#54842=CARTESIAN_POINT('Ctrl Pts',(-10.4943736969631,-0.823229081731838,
1.817857706982));
#54843=CARTESIAN_POINT('Ctrl Pts',(-10.3832273520857,-1.97378057551948,
0.294113929532303));
#54844=CARTESIAN_POINT('Ctrl Pts',(-10.2720810072083,-1.31745663804804,
-1.49887316698446));
#54845=CARTESIAN_POINT('Ctrl Pts',(-10.1609346623308,0.544918296460699,
-1.91973352682743));
#54846=CARTESIAN_POINT('Ctrl Pts',(-10.0497883174534,1.90845384926197,-0.583195223814541));
#54847=CARTESIAN_POINT('Ctrl Pts',(-9.93864197257597,1.52491659432944,1.28722264747851));
#54848=CARTESIAN_POINT('Ctrl Pts',(-9.82749562769855,-0.254588562601471,
1.97926689146143));
#54849=CARTESIAN_POINT('Ctrl Pts',(-9.71634928282112,-1.80103345713564,
0.859413317397949));
#54850=CARTESIAN_POINT('Ctrl Pts',(-9.60520293794371,-1.69874234477226,
-1.04718060043171));
#54851=CARTESIAN_POINT('Ctrl Pts',(-9.49405659306628,-0.0413564843513104,
-1.99514470779566));
#54852=CARTESIAN_POINT('Ctrl Pts',(-9.38291024818885,1.65388870877585,-1.11667582709874));
#54853=CARTESIAN_POINT('Ctrl Pts',(-9.27176390331144,1.83509991505148,0.784041494833618));
#54854=CARTESIAN_POINT('Ctrl Pts',(-9.16061755843401,0.336389355180736,
1.96701676799259));
#54855=CARTESIAN_POINT('Ctrl Pts',(-9.04947121355659,-1.47026509103269,
1.3493084621144));
#54856=CARTESIAN_POINT('Ctrl Pts',(-8.93832486867916,-1.93098174488252,
-0.503609238173173));
#54857=CARTESIAN_POINT('Ctrl Pts',(-8.82717852380175,-0.62400268001261,
-1.89550347379793));
#54858=CARTESIAN_POINT('Ctrl Pts',(-8.71603217892431,1.25421268413938,-1.55218017858327));
#54859=CARTESIAN_POINT('Ctrl Pts',(-8.60488583404689,1.9842730240438,0.212069162998644));
#54860=CARTESIAN_POINT('Ctrl Pts',(-8.49373948916947,0.897852737619631,
1.78218215269705));
#54861=CARTESIAN_POINT('Ctrl Pts',(-8.38259314429204,-1.01049683142839,
1.7208163520597));
#54862=CARTESIAN_POINT('Ctrl Pts',(-8.27144679941463,-1.99379833752617,
0.084148399395079));
#54863=CARTESIAN_POINT('Ctrl Pts',(-8.16030045453719,-1.15189937522182,
-1.62955226771236));
#54864=CARTESIAN_POINT('Ctrl Pts',(-8.04915410965978,0.744493032901956,
-1.8514974717248));
#54865=CARTESIAN_POINT('Ctrl Pts',(-7.93800776478235,1.95934759098379,-0.378509949075211));
#54866=CARTESIAN_POINT('Ctrl Pts',(-7.82686141990493,1.38053923265282,1.44098028818902));
#54867=CARTESIAN_POINT('Ctrl Pts',(-7.71571507502751,-0.46206838092876,
1.94134117949132));
#54868=CARTESIAN_POINT('Ctrl Pts',(-7.60456873015007,-1.88168064466396,
0.664522923110952));
#54869=CARTESIAN_POINT('Ctrl Pts',(-7.49342238527267,-1.57872933244332,
-1.22062543752209));
#54870=CARTESIAN_POINT('Ctrl Pts',(-7.38227604039523,0.169452153171387,
-1.98836584451364));
#54871=CARTESIAN_POINT('Ctrl Pts',(-7.27112969551781,1.76251055360792,-0.93587889828952));
#54872=CARTESIAN_POINT('Ctrl Pts',(-7.1599833506404,1.74209830986671,0.973347955564964));
#54873=CARTESIAN_POINT('Ctrl Pts',(-7.04883700576295,0.126901582998413,
1.99153427087645));
#54874=CARTESIAN_POINT('Ctrl Pts',(-6.93769066088555,-1.60446578378376,
1.18659273236863));
#54875=CARTESIAN_POINT('Ctrl Pts',(-6.82654431600812,-1.86704282960959,
-0.704601899122013));
#54876=CARTESIAN_POINT('Ctrl Pts',(-6.71539797113069,-0.420456324141416,
-1.9507765744268));
#54877=CARTESIAN_POINT('Ctrl Pts',(-6.60425162625326,1.41103223752855,-1.41113457490704));
#54878=CARTESIAN_POINT('Ctrl Pts',(-6.49310528137585,1.95080706246068,0.420314844963218));
#54879=CARTESIAN_POINT('Ctrl Pts',(-6.38195893649842,0.704737302637404,
1.86699172416866));
#54880=CARTESIAN_POINT('Ctrl Pts',(-6.27081259162099,-1.18647636701088,
1.60455183598647));
#54881=CARTESIAN_POINT('Ctrl Pts',(-6.15966624674359,-1.99154346904629,
-0.126757148682046));
#54882=CARTESIAN_POINT('Ctrl Pts',(-6.04851990186614,-0.9734742969003,-1.74202771422195));
#54883=CARTESIAN_POINT('Ctrl Pts',(-5.93737355698873,0.935751071556099,
-1.76257842263103));
#54884=CARTESIAN_POINT('Ctrl Pts',(-5.82622721211131,1.98835354994073,-0.169596356921512));
#54885=CARTESIAN_POINT('Ctrl Pts',(-5.71508086723387,1.2207399300394,1.57864080368217));
#54886=CARTESIAN_POINT('Ctrl Pts',(-5.60393452235647,-0.664386454402397,
1.88172883355958));
#54887=CARTESIAN_POINT('Ctrl Pts',(-5.49278817747902,-1.94130766334994,
0.462209173493692));
#54888=CARTESIAN_POINT('Ctrl Pts',(-5.38164183260162,-1.44108040659289,
-1.38043472340309));
#54889=CARTESIAN_POINT('Ctrl Pts',(-5.27049548772418,0.37836784840312,-1.95937503687724));
#54890=CARTESIAN_POINT('Ctrl Pts',(-5.15934914284677,1.85144347326116,-0.744627308901291));
#54891=CARTESIAN_POINT('Ctrl Pts',(-5.04820279796934,1.6296358037489,1.15178119058377));
#54892=CARTESIAN_POINT('Ctrl Pts',(-4.93705645309192,-0.0840038009920192,
1.99380443505921));
#54893=CARTESIAN_POINT('Ctrl Pts',(-4.8259101082145,-1.72074306228678,1.01062162921386));
#54894=CARTESIAN_POINT('Ctrl Pts',(-4.71476376333707,-1.78224726386006,
-0.89772348432365));
#54895=CARTESIAN_POINT('Ctrl Pts',(-4.60361741845965,-0.2122130698091,-1.98425763872665));
#54896=CARTESIAN_POINT('Ctrl Pts',(-4.49247107358223,1.55208921401132,-1.25432525111822));
#54897=CARTESIAN_POINT('Ctrl Pts',(-4.3813247287048,1.89554872396803,0.623865208924149));
#54898=CARTESIAN_POINT('Ctrl Pts',(-4.27017838382738,0.503749279321564,
1.93094521606016));
#54899=CARTESIAN_POINT('Ctrl Pts',(-4.15903203894995,-1.34920182909664,
1.4703629443801));
#54900=CARTESIAN_POINT('Ctrl Pts',(-4.04788569407253,-1.96704115911265,
-0.336246698420522));
#54901=CARTESIAN_POINT('Ctrl Pts',(-3.93673934919511,-0.784174581513545,
-1.83504304841865));
#54902=CARTESIAN_POINT('Ctrl Pts',(-3.82559300431769,1.11655587757895,-1.65396969019784));
#54903=CARTESIAN_POINT('Ctrl Pts',(-3.71444665944026,1.99514770188327,0.041211788418896));
#54904=CARTESIAN_POINT('Ctrl Pts',(-3.60330031456284,1.04730379722992,1.69866639460034));
#54905=CARTESIAN_POINT('Ctrl Pts',(-3.49215396968541,-0.859282697039027,
1.80109578047766));
#54906=CARTESIAN_POINT('Ctrl Pts',(-3.38100762480799,-1.97924842246725,
0.254732106220004));
#54907=CARTESIAN_POINT('Ctrl Pts',(-3.26986127993057,-1.28733323713422,
-1.52482323578601));
#54908=CARTESIAN_POINT('Ctrl Pts',(-3.15871493505314,0.583056813672423,
-1.90849613993501));
#54909=CARTESIAN_POINT('Ctrl Pts',(-3.04756859017572,1.91969400203911,-0.545057521628532));
#54910=CARTESIAN_POINT('Ctrl Pts',(-2.9364222452983,1.49896871042294,1.31734793014021));
#54911=CARTESIAN_POINT('Ctrl Pts',(-2.82527590042087,-0.293970782701203,
1.97380190102493));
#54912=CARTESIAN_POINT('Ctrl Pts',(-2.71412955554345,-1.81779799767748,
0.8233609171026));
#54913=CARTESIAN_POINT('Ctrl Pts',(-2.60298321066602,-1.67754229632962,
-1.08081663994663));
#54914=CARTESIAN_POINT('Ctrl Pts',(-2.49183686578861,-0.00159919047849908,
-1.99557265390096));
#54915=CARTESIAN_POINT('Ctrl Pts',(-2.38069052091117,1.67580786785562,-1.08350391199696));
#54916=CARTESIAN_POINT('Ctrl Pts',(-2.26954417603376,1.8191153058292,0.82044639344388));
#54917=CARTESIAN_POINT('Ctrl Pts',(-2.15839783115632,0.297133878843009,
1.97332822505901));
#54918=CARTESIAN_POINT('Ctrl Pts',(-2.04725148627891,-1.49685538682514,
1.31974866055417));
#54919=CARTESIAN_POINT('Ctrl Pts',(-1.93610514140148,-1.92056518303343,
-0.54197998561013));
#54920=CARTESIAN_POINT('Ctrl Pts',(-1.82495879652407,-0.586114771301867,
-1.9075593257576));
#54921=CARTESIAN_POINT('Ctrl Pts',(-1.71381245164663,1.28488746754462,-1.52688429885936));
#54922=CARTESIAN_POINT('Ctrl Pts',(-1.60266610676922,1.9796545703674,0.251559104539083));
#54923=CARTESIAN_POINT('Ctrl Pts',(-1.49151976189179,0.862167481052224,
1.79971712455831));
#54924=CARTESIAN_POINT('Ctrl Pts',(-1.38037341701437,-1.04457840936319,
1.70034112479895));
#54925=CARTESIAN_POINT('Ctrl Pts',(-1.26922707213694,-1.99508198357073,
0.0444125647564481));
#54926=CARTESIAN_POINT('Ctrl Pts',(-1.15808072725952,-1.1191998176419,-1.65218396478253));
#54927=CARTESIAN_POINT('Ctrl Pts',(-1.04693438238209,0.78122199815978,-1.83628620557567));
#54928=CARTESIAN_POINT('Ctrl Pts',(-0.935788037504671,1.96651965162107,
-0.339420443694009));
#54929=CARTESIAN_POINT('Ctrl Pts',(-0.82464169262725,1.35151878363549,1.46823957714146));
#54930=CARTESIAN_POINT('Ctrl Pts',(-0.713495347749821,-0.500581689657017,
1.93167223103872));
#54931=CARTESIAN_POINT('Ctrl Pts',(-0.602349002872402,-1.89468364489563,
0.627050666299228));
#54932=CARTESIAN_POINT('Ctrl Pts',(-0.491202657994974,-1.55383632121744,
-1.25211820325569));
#54933=CARTESIAN_POINT('Ctrl Pts',(-0.380056313117557,0.208534092580134,
-1.98405617855194));
#54934=CARTESIAN_POINT('Ctrl Pts',(-0.268909968240128,1.78176704590796,
-0.90162390006292));
#54935=CARTESIAN_POINT('Ctrl Pts',(-0.157763623362708,1.72042361801685,
1.01001860971832));
#54936=CARTESIAN_POINT('Ctrl Pts',(-0.0836660601110885,0.634691421918637,
1.66218726645698));
#54937=CARTESIAN_POINT('Ctrl Pts',(-0.0466172784852814,0.0737739821678156,
1.68672073681435));
#54938=CARTESIAN_POINT('Ctrl Pts',(-29.646,0.903606778650087,-1.26612599672292));
#54939=CARTESIAN_POINT('Ctrl Pts',(-29.6089512183742,1.32465582191086,-0.965632388172658));
#54940=CARTESIAN_POINT('Ctrl Pts',(-29.5348536551225,1.83614857151059,0.0831884196457774));
#54941=CARTESIAN_POINT('Ctrl Pts',(-29.4237073102452,0.924038956922092,
1.59090722470862));
#54942=CARTESIAN_POINT('Ctrl Pts',(-29.3125609653677,-0.83473688776688,
1.63754421834404));
#54943=CARTESIAN_POINT('Ctrl Pts',(-29.2014146204903,-1.82895987007768,
0.187471477219877));
#54944=CARTESIAN_POINT('Ctrl Pts',(-29.0902682756128,-1.14909344713552,
-1.43544860892843));
#54945=CARTESIAN_POINT('Ctrl Pts',(-28.9791219307355,0.582808968573894,
-1.74365887083216));
#54946=CARTESIAN_POINT('Ctrl Pts',(-28.867975585858,1.78112695043666,-0.455994626000207));
#54947=CARTESIAN_POINT('Ctrl Pts',(-28.7568292409806,1.34896284622222,1.24928278177877));
#54948=CARTESIAN_POINT('Ctrl Pts',(-28.6456828961032,-0.318110417184717,
1.81082463803951));
#54949=CARTESIAN_POINT('Ctrl Pts',(-28.5345365512258,-1.69396455183104,
0.714716438603391));
#54950=CARTESIAN_POINT('Ctrl Pts',(-28.4233902063484,-1.51910218013106,
-1.0356968120803));
#54951=CARTESIAN_POINT('Ctrl Pts',(-28.3122438614709,0.046407699775919,
-1.83797936794685));
#54952=CARTESIAN_POINT('Ctrl Pts',(-28.2010975165935,1.56943293437681,-0.95771133892945));
#54953=CARTESIAN_POINT('Ctrl Pts',(-28.089951171716,1.65573892814966,0.799286617882397));
#54954=CARTESIAN_POINT('Ctrl Pts',(-27.9788048268387,0.226316831424914,
1.82458457360074));
#54955=CARTESIAN_POINT('Ctrl Pts',(-27.8676584819612,-1.41028430723429,
1.1795879531954));
#54956=CARTESIAN_POINT('Ctrl Pts',(-27.7565121370838,-1.75585648782649,
-0.545249858763614));
#54957=CARTESIAN_POINT('Ctrl Pts',(-27.6453657922064,-0.494049365075557,
-1.77094447718388));
#54958=CARTESIAN_POINT('Ctrl Pts',(-27.534219447329,1.22002971701301,-1.37544786085574));
#54959=CARTESIAN_POINT('Ctrl Pts',(-27.4230731024515,1.81724620484857,0.279187250412826));
#54960=CARTESIAN_POINT('Ctrl Pts',(-27.3119267575741,0.750884899378822,
1.67824346299867));
#54961=CARTESIAN_POINT('Ctrl Pts',(-27.2007804126967,-1.00286561528311,
1.54097042230253));
#54962=CARTESIAN_POINT('Ctrl Pts',(-27.0896340678193,-1.83855398075809,
-0.00696682981420152));
#54963=CARTESIAN_POINT('Ctrl Pts',(-26.9784877229418,-0.991158593083783,
-1.54852636916561));
#54964=CARTESIAN_POINT('Ctrl Pts',(-26.8673413780644,0.763581882211757,
-1.67250470444365));
#54965=CARTESIAN_POINT('Ctrl Pts',(-26.756195033187,1.81930983338734,-0.265407245427431));
#54966=CARTESIAN_POINT('Ctrl Pts',(-26.6450486883096,1.20957087255313,1.38465431773148));
#54967=CARTESIAN_POINT('Ctrl Pts',(-26.5339023434321,-0.507456263538371,
1.76714951732695));
#54968=CARTESIAN_POINT('Ctrl Pts',(-26.4227559985548,-1.75993821851123,
0.531927384863541));
#54969=CARTESIAN_POINT('Ctrl Pts',(-26.3116096536772,-1.4013043447814,-1.1902417439339));
#54970=CARTESIAN_POINT('Ctrl Pts',(-26.2004633087999,0.240137974670818,
-1.8228173328443));
#54971=CARTESIAN_POINT('Ctrl Pts',(-26.0893169639224,1.66174866141038,-0.786715108572567));
#54972=CARTESIAN_POINT('Ctrl Pts',(-25.978170619045,1.56213005525038,0.969576694355506));
#54973=CARTESIAN_POINT('Ctrl Pts',(-25.8670242741676,0.032476899015307,
1.8382803177961));
#54974=CARTESIAN_POINT('Ctrl Pts',(-25.7558779292902,-1.52690687248867,
1.02415071083631));
#54975=CARTESIAN_POINT('Ctrl Pts',(-25.6447315844127,-1.68850076403338,
-0.727526250810708));
#54976=CARTESIAN_POINT('Ctrl Pts',(-25.5335852395354,-0.304375448471892,
-1.81319741399803));
#54977=CARTESIAN_POINT('Ctrl Pts',(-25.4224388946579,1.35838697931157,-1.23899721153737));
#54978=CARTESIAN_POINT('Ctrl Pts',(-25.3112925497805,1.77762918529204,0.469429180344255));
#54979=CARTESIAN_POINT('Ctrl Pts',(-25.200146204903,0.569560564207642,1.74812186058649));
#54980=CARTESIAN_POINT('Ctrl Pts',(-25.0889998600256,-1.1599059279699,1.42651586532399));
#54981=CARTESIAN_POINT('Ctrl Pts',(-24.9778535151482,-1.82754946484302,
-0.200978181185898));
#54982=CARTESIAN_POINT('Ctrl Pts',(-24.8667071702708,-0.822183211067854,
-1.64448899151042));
#54983=CARTESIAN_POINT('Ctrl Pts',(-24.7555608253933,0.935841500540801,
-1.58257068139984));
#54984=CARTESIAN_POINT('Ctrl Pts',(-24.644414480516,1.8371605398714,-0.071905677802479));
#54985=CARTESIAN_POINT('Ctrl Pts',(-24.5332681356385,1.05667143702865,1.50458457719352));
#54986=CARTESIAN_POINT('Ctrl Pts',(-24.4221217907611,-0.691135756872815,
1.70371964869008));
#54987=CARTESIAN_POINT('Ctrl Pts',(-24.3109754458837,-1.80625042443839,
0.343203554726555));
#54988=CARTESIAN_POINT('Ctrl Pts',(-24.1998291010062,-1.26785327052907,
-1.3314944086137));
#54989=CARTESIAN_POINT('Ctrl Pts',(-24.0886827561288,0.431186030422094,
-1.78729065429483));
#54990=CARTESIAN_POINT('Ctrl Pts',(-23.9775364112514,1.73550088513296,-0.606931588783731));
#54991=CARTESIAN_POINT('Ctrl Pts',(-23.866390066374,1.45107079566491,1.12903623579104));
#54992=CARTESIAN_POINT('Ctrl Pts',(-23.7552437214966,-0.161725882381191,
1.83144042074233));
#54993=CARTESIAN_POINT('Ctrl Pts',(-23.6440973766191,-1.62647240373936,
0.857272882829682));
#54994=CARTESIAN_POINT('Ctrl Pts',(-23.5329510317417,-1.60228288915339,
-0.901675561877481));
#54995=CARTESIAN_POINT('Ctrl Pts',(-23.4218046868643,-0.111301360173381,
-1.83519516209704));
#54996=CARTESIAN_POINT('Ctrl Pts',(-23.3106583419868,1.48156975859047,-1.08870580332383));
#54997=CARTESIAN_POINT('Ctrl Pts',(-23.1995119971095,1.7181543530587,0.654427150129224));
#54998=CARTESIAN_POINT('Ctrl Pts',(-23.088365652232,0.381873692818719,1.79847206219441));
#54999=CARTESIAN_POINT('Ctrl Pts',(-22.9772193073546,-1.30398898375897,
1.29612576781578));
#55000=CARTESIAN_POINT('Ctrl Pts',(-22.8660729624772,-1.79612947732935,
-0.392744416165795));
#55001=CARTESIAN_POINT('Ctrl Pts',(-22.7549266175997,-0.644023257663918,
-1.72208110126926));
#55002=CARTESIAN_POINT('Ctrl Pts',(-22.6437802727223,1.09764687597715,-1.47495783377641));
#55003=CARTESIAN_POINT('Ctrl Pts',(-22.5326339278449,1.83448840962079,0.122399145126971));
#55004=CARTESIAN_POINT('Ctrl Pts',(-22.4214875829675,0.891967972949703,
1.6077071906889));
#55005=CARTESIAN_POINT('Ctrl Pts',(-22.3103412380901,-0.867094604110294,
1.6212576054667));
#55006=CARTESIAN_POINT('Ctrl Pts',(-22.1991948932126,-1.83238508908664,
0.150645813263272));
#55007=CARTESIAN_POINT('Ctrl Pts',(-22.0880485483352,-1.12023906509101,
-1.45787300983482));
#55008=CARTESIAN_POINT('Ctrl Pts',(-21.9769022034578,0.617417326649948,
-1.73179823319959));
#55009=CARTESIAN_POINT('Ctrl Pts',(-21.8657558585803,1.78986590745487,-0.420368063834038));
#55010=CARTESIAN_POINT('Ctrl Pts',(-21.7546095137029,1.32380169026185,1.27588336481854));
#55011=CARTESIAN_POINT('Ctrl Pts',(-21.6434631688255,-0.35412203130582,
1.80414158610255));
#55012=CARTESIAN_POINT('Ctrl Pts',(-21.532316823948,-1.70786868579214,0.680818498464482));
#55013=CARTESIAN_POINT('Ctrl Pts',(-21.4211704790707,-1.49816598504183,
-1.06575229627923));
#55014=CARTESIAN_POINT('Ctrl Pts',(-21.3100241341932,0.0830160705540191,
-1.83669202856401));
#55015=CARTESIAN_POINT('Ctrl Pts',(-21.1988777893158,1.58820198952549,-0.926252512130515));
#55016=CARTESIAN_POINT('Ctrl Pts',(-21.0877314444384,1.6394860967441,0.832114544004366));
#55017=CARTESIAN_POINT('Ctrl Pts',(-20.976585099561,0.189920927787188,1.82873161424777));
#55018=CARTESIAN_POINT('Ctrl Pts',(-20.8654387546835,-1.43350523795772,
1.15125670834466));
#55019=CARTESIAN_POINT('Ctrl Pts',(-20.7542924098061,-1.74464500917001,
-0.580123321147311));
#55020=CARTESIAN_POINT('Ctrl Pts',(-20.6431460649287,-0.458668949759455,
-1.78043592142131));
#55021=CARTESIAN_POINT('Ctrl Pts',(-20.5319997200512,1.24719048811815,-1.35086829932027));
#55022=CARTESIAN_POINT('Ctrl Pts',(-20.4208533751738,1.81132329283767,0.315336652776849));
#55023=CARTESIAN_POINT('Ctrl Pts',(-20.3097070302964,0.717300375240254,
1.69287018032718));
#55024=CARTESIAN_POINT('Ctrl Pts',(-20.198560685419,-1.03336717698855,1.52068456731945));
#55025=CARTESIAN_POINT('Ctrl Pts',(-20.0874143405416,-1.83805026330036,
-0.0435947857237916));
#55026=CARTESIAN_POINT('Ctrl Pts',(-19.9762679956642,-0.960110720041205,
-1.56796577801391));
#55027=CARTESIAN_POINT('Ctrl Pts',(-19.8651216507867,0.796751482021758,
-1.65695997285902));
#55028=CARTESIAN_POINT('Ctrl Pts',(-19.7539753059093,1.82423641918512,-0.229108626375055));
#55029=CARTESIAN_POINT('Ctrl Pts',(-19.6428289610319,1.18174445642581,1.40847765884577));
#55030=CARTESIAN_POINT('Ctrl Pts',(-19.5316826161545,-0.542562299135568,
1.75668876791466));
#55031=CARTESIAN_POINT('Ctrl Pts',(-19.420536271277,-1.77018644448459,0.49675872163839));
#55032=CARTESIAN_POINT('Ctrl Pts',(-19.3093899263996,-1.37731313689601,
-1.21792356028385));
#55033=CARTESIAN_POINT('Ctrl Pts',(-19.1982435815222,0.276406132535501,
-1.81767129197156));
#55034=CARTESIAN_POINT('Ctrl Pts',(-19.0870972366448,1.67709248831789,-0.75345209627986));
#55035=CARTESIAN_POINT('Ctrl Pts',(-18.9759508917673,1.5425032158592,1.0005064241797));
#55036=CARTESIAN_POINT('Ctrl Pts',(-18.8648045468899,-0.00415343528496038,
1.83856248866775));
#55037=CARTESIAN_POINT('Ctrl Pts',(-18.7536582020125,-1.54700787038504,
0.993527012580707));
#55038=CARTESIAN_POINT('Ctrl Pts',(-18.6425118571351,-1.67367119101565,
-0.761021694910901));
#55039=CARTESIAN_POINT('Ctrl Pts',(-18.5313655122577,-0.268190871892204,
-1.8189015729265));
#55040=CARTESIAN_POINT('Ctrl Pts',(-18.4202191673802,1.38280179207861,-1.21168827657323));
#55041=CARTESIAN_POINT('Ctrl Pts',(-18.3090728225028,1.76792396598735,0.504751549030178));
#55042=CARTESIAN_POINT('Ctrl Pts',(-18.1979264776254,0.534619847684823,
1.75912219422707));
#55043=CARTESIAN_POINT('Ctrl Pts',(-18.0867801327479,-1.18809605216334,
1.40312403108018));
#55044=CARTESIAN_POINT('Ctrl Pts',(-17.9756337878705,-1.82318266167623,
-0.237348389343613));
#55045=CARTESIAN_POINT('Ctrl Pts',(-17.8644874429931,-0.789257021834459,
-1.66054287184818));
#55046=CARTESIAN_POINT('Ctrl Pts',(-17.7533410981157,0.967185162849705,
-1.56361188807332));
#55047=CARTESIAN_POINT('Ctrl Pts',(-17.6421947532383,1.83822846890144,-0.0352898268780593));
#55048=CARTESIAN_POINT('Ctrl Pts',(-17.5310484083608,1.0264860090507,1.52533791304877));
#55049=CARTESIAN_POINT('Ctrl Pts',(-17.4199020634834,-0.724941628214821,
1.68961205945094));
#55050=CARTESIAN_POINT('Ctrl Pts',(-17.308755718606,-1.81272953097057,0.307149675741386));
#55051=CARTESIAN_POINT('Ctrl Pts',(-17.1976093737286,-1.24107438638229,
-1.35648945562677));
#55052=CARTESIAN_POINT('Ctrl Pts',(-17.0864630288511,0.466708474190256,
-1.7783454321025));
#55053=CARTESIAN_POINT('Ctrl Pts',(-16.9753166839737,1.74724826325126,-0.572234901352823));
#55054=CARTESIAN_POINT('Ctrl Pts',(-16.8641703390963,1.42828910175244,1.15772169262565));
#55055=CARTESIAN_POINT('Ctrl Pts',(-16.7530239942189,-0.19818140052057,
1.82785486520361));
#55056=CARTESIAN_POINT('Ctrl Pts',(-16.6418776493414,-1.64322894829983,
0.824698671776694));
#55057=CARTESIAN_POINT('Ctrl Pts',(-16.530731304464,-1.58400086815871,-0.933418729956337));
#55058=CARTESIAN_POINT('Ctrl Pts',(-16.4195849595866,-0.0747168460009575,
-1.83704835774251));
#55059=CARTESIAN_POINT('Ctrl Pts',(-16.3084386147092,1.50296588015394,-1.05897253923504));
#55060=CARTESIAN_POINT('Ctrl Pts',(-16.1972922698318,1.70477524097488,0.688527888701595));
#55061=CARTESIAN_POINT('Ctrl Pts',(-16.0861459249543,0.345967106142554,
1.80572313415655));
#55062=CARTESIAN_POINT('Ctrl Pts',(-15.9749995800769,-1.32955276041214,
1.26988926014879));
#55063=CARTESIAN_POINT('Ctrl Pts',(-15.8638532351995,-1.78794836951534,
-0.428450584908307));
#55064=CARTESIAN_POINT('Ctrl Pts',(-15.7527068903221,-0.609586569357517,
-1.73457011683579));
#55065=CARTESIAN_POINT('Ctrl Pts',(-15.6415605454446,1.12681446224207,-1.45279676604917));
#55066=CARTESIAN_POINT('Ctrl Pts',(-15.5304142005672,1.83168575205326,0.158923193668888));
#55067=CARTESIAN_POINT('Ctrl Pts',(-15.4192678556898,0.859760733185979,
1.6251586868464));
#55068=CARTESIAN_POINT('Ctrl Pts',(-15.3081215108124,-0.899222667358879,
1.60366077156884));
#55069=CARTESIAN_POINT('Ctrl Pts',(-15.1969751659349,-1.83502269836715,
0.114109474795715));
#55070=CARTESIAN_POINT('Ctrl Pts',(-15.0858288210575,-1.09097165038219,
-1.47990206899753));
#55071=CARTESIAN_POINT('Ctrl Pts',(-14.9746824761801,0.651797236720689,
-1.71915375634761));
#55072=CARTESIAN_POINT('Ctrl Pts',(-14.8635361313027,1.79788560735673,-0.384625296386388));
#55073=CARTESIAN_POINT('Ctrl Pts',(-14.7523897864252,1.29811963509442,1.30200410473359));
#55074=CARTESIAN_POINT('Ctrl Pts',(-14.6412434415478,-0.389995490350614,
1.79672835822976));
#55075=CARTESIAN_POINT('Ctrl Pts',(-14.5300970966704,-1.72109359041992,
0.646657659644004));
#55076=CARTESIAN_POINT('Ctrl Pts',(-14.418950751793,-1.47663574369473,-1.09538858685122));
#55077=CARTESIAN_POINT('Ctrl Pts',(-14.3078044069155,0.119591838376424,
-1.83467355896208));
#55078=CARTESIAN_POINT('Ctrl Pts',(-14.1966580620381,1.60634040478516,-0.894427067857099));
#55079=CARTESIAN_POINT('Ctrl Pts',(-14.0855117171607,1.62258254933333,0.864612714664634));
#55080=CARTESIAN_POINT('Ctrl Pts',(-13.9743653722833,0.153449581803269,
1.83215242313658));
#55081=CARTESIAN_POINT('Ctrl Pts',(-13.8632190274059,-1.45615709528508,
1.1224686140876));
#55082=CARTESIAN_POINT('Ctrl Pts',(-13.7520726825284,-1.73274098749183,
-0.614766578488641));
#55083=CARTESIAN_POINT('Ctrl Pts',(-13.640926337651,-0.423106453057855,
-1.78922055799212));
#55084=CARTESIAN_POINT('Ctrl Pts',(-13.5297799927736,1.27385616856038,-1.32575251747129));
#55085=CARTESIAN_POINT('Ctrl Pts',(-13.4186336478962,1.8046813570327,0.351360890452264));
#55086=CARTESIAN_POINT('Ctrl Pts',(-13.3074873030187,0.683431109300355,
1.70682488691761));
#55087=CARTESIAN_POINT('Ctrl Pts',(-13.1963409581413,-1.06345853101135,
1.49979506219349));
#55088=CARTESIAN_POINT('Ctrl Pts',(-13.0851946132639,-1.83681691071596,
-0.0802054378995563));
#55089=CARTESIAN_POINT('Ctrl Pts',(-12.9740482683865,-0.928681719728038,
-1.58678276370895));
#55090=CARTESIAN_POINT('Ctrl Pts',(-12.8629019235091,0.829604801984373,
-1.64075749222281));
#55091=CARTESIAN_POINT('Ctrl Pts',(-12.7517555786316,1.82843885316793,-0.192719059739105));
#55092=CARTESIAN_POINT('Ctrl Pts',(-12.6406092337542,1.15344893307288,1.43174188824448));
#55093=CARTESIAN_POINT('Ctrl Pts',(-12.5294628888768,-0.577452958307463,
1.74553068053895));
#55094=CARTESIAN_POINT('Ctrl Pts',(-12.4183165439994,-1.77973197437198,
0.461392864226164));
#55095=CARTESIAN_POINT('Ctrl Pts',(-12.3071701991219,-1.35277518854269,
-1.24512190769584));
#55096=CARTESIAN_POINT('Ctrl Pts',(-12.1960238542445,0.312564567770197,
-1.81180370535426));
#55097=CARTESIAN_POINT('Ctrl Pts',(-12.0848775093671,1.69177057386242,-0.719889992411354));
#55098=CARTESIAN_POINT('Ctrl Pts',(-11.9737311644897,1.52226406188029,1.0310389913425));
#55099=CARTESIAN_POINT('Ctrl Pts',(-11.8625848196122,-0.0407821208305537,
1.83811482078279));
#55100=CARTESIAN_POINT('Ctrl Pts',(-11.7514384747348,-1.56649476551932,
0.962508922224293));
#55101=CARTESIAN_POINT('Ctrl Pts',(-11.6402921298574,-1.6581772347577,-0.794215042600007));
#55102=CARTESIAN_POINT('Ctrl Pts',(-11.52914578498,-0.231899833827511,-1.82388369772625));
#55103=CARTESIAN_POINT('Ctrl Pts',(-11.4179994401025,1.40666768559556,-1.18389834785848));
#55104=CARTESIAN_POINT('Ctrl Pts',(-11.3068530952251,1.75751694870754,0.539873550719585));
#55105=CARTESIAN_POINT('Ctrl Pts',(-11.1957067503477,0.499466907597081,
1.7694242238582));
#55106=CARTESIAN_POINT('Ctrl Pts',(-11.0845604054703,-1.21581454781411,
1.37917521043716));
#55107=CARTESIAN_POINT('Ctrl Pts',(-10.9734140605928,-1.81809212495253,
-0.273624379298372));
#55108=CARTESIAN_POINT('Ctrl Pts',(-10.8622677157155,-0.756017527849028,
-1.67593758038474));
#55109=CARTESIAN_POINT('Ctrl Pts',(-10.751121370838,0.998144889762121,-1.54403240082667));
#55110=CARTESIAN_POINT('Ctrl Pts',(-10.6399750259606,1.83856669176645,0.00134003275348477));
#55111=CARTESIAN_POINT('Ctrl Pts',(-10.5288286810832,0.99589310551582,1.54548574828332));
#55112=CARTESIAN_POINT('Ctrl Pts',(-10.4176823362057,-0.758459725548137,
1.67483375905857));
#55113=CARTESIAN_POINT('Ctrl Pts',(-10.3065359913283,-1.81848905343763,
0.270973870120994));
#55114=CARTESIAN_POINT('Ctrl Pts',(-10.1953896464509,-1.21380284332704,
-1.38094602837764));
#55115=CARTESIAN_POINT('Ctrl Pts',(-10.0842433015735,0.502045652602867,
-1.76869427501289));
#55116=CARTESIAN_POINT('Ctrl Pts',(-9.97309695669603,1.75830205085506,-0.537311058624067));
#55117=CARTESIAN_POINT('Ctrl Pts',(-9.86195061181863,1.40494043187336,1.1859475783728));
#55118=CARTESIAN_POINT('Ctrl Pts',(-9.75080426694118,-0.234558248248651,
1.82354372142247));
#55119=CARTESIAN_POINT('Ctrl Pts',(-9.63965792206378,-1.65933319402237,
0.791797086996613));
#55120=CARTESIAN_POINT('Ctrl Pts',(-9.52851157718634,-1.56509005960118,
-0.964791366616839));
#55121=CARTESIAN_POINT('Ctrl Pts',(-9.41736523230892,-0.0381026721077461,
-1.83817231568183));
#55122=CARTESIAN_POINT('Ctrl Pts',(-9.30621888743151,1.5237653819353,-1.02881890368343));
#55123=CARTESIAN_POINT('Ctrl Pts',(-9.19507254255407,1.6907193985366,0.722355308122558));
#55124=CARTESIAN_POINT('Ctrl Pts',(-9.08392619767666,0.309923183800838,
1.81225740332426));
#55125=CARTESIAN_POINT('Ctrl Pts',(-8.97277985279922,-1.35458875563747,
1.24314865517416));
#55126=CARTESIAN_POINT('Ctrl Pts',(-8.86163350792181,-1.77905751480639,
-0.463986675209236));
#55127=CARTESIAN_POINT('Ctrl Pts',(-8.75048716304438,-0.574907898574367,
-1.74637057462545));
#55128=CARTESIAN_POINT('Ctrl Pts',(-8.63934081816696,1.15553474640397,-1.43005899375302));
#55129=CARTESIAN_POINT('Ctrl Pts',(-8.52819447328953,1.82815598552823,0.195384155801151));
#55130=CARTESIAN_POINT('Ctrl Pts',(-8.41704812841212,0.827212201402232,
1.64196505736636));
#55131=CARTESIAN_POINT('Ctrl Pts',(-8.30590178353469,-0.930993773713778,
1.58542734588091));
#55132=CARTESIAN_POINT('Ctrl Pts',(-8.19475543865727,-1.83693187405052,
0.0775278392453074));
#55133=CARTESIAN_POINT('Ctrl Pts',(-8.08360909377984,-1.0612711617913,-1.50134366382617));
#55134=CARTESIAN_POINT('Ctrl Pts',(-7.97246274890243,0.685918408299438,
-1.70582684142229));
#55135=CARTESIAN_POINT('Ctrl Pts',(-7.86131640402499,1.80519161566156,-0.348729847455048));
#55136=CARTESIAN_POINT('Ctrl Pts',(-7.75017005914758,1.27192227624375,1.32760799898003));
#55137=CARTESIAN_POINT('Ctrl Pts',(-7.63902371427015,-0.425714136150784,
1.7886018981434));
#55138=CARTESIAN_POINT('Ctrl Pts',(-7.52787736939272,-1.7336352869347,0.612240122546414));
#55139=CARTESIAN_POINT('Ctrl Pts',(-7.4167310245153,-1.45451933461935,-1.12459005018688));
#55140=CARTESIAN_POINT('Ctrl Pts',(-7.30558467963788,0.156120132828023,
-1.83192679435794));
#55141=CARTESIAN_POINT('Ctrl Pts',(-7.19443833476045,1.62384116454318,-0.862246570359003));
#55142=CARTESIAN_POINT('Ctrl Pts',(-7.08329198988304,1.60503489891277,0.896767667254413));
#55143=CARTESIAN_POINT('Ctrl Pts',(-6.97214564500561,0.116917322223582,
1.83484593781736));
#55144=CARTESIAN_POINT('Ctrl Pts',(-6.86099930012818,-1.47823091412176,
1.09323494286248));
#55145=CARTESIAN_POINT('Ctrl Pts',(-6.74985295525077,-1.72014913413095,
-0.649165797088362));
#55146=CARTESIAN_POINT('Ctrl Pts',(-6.63870661037334,-0.387375999329962,
-1.79729494265797));
#55147=CARTESIAN_POINT('Ctrl Pts',(-6.5275602654959,1.30001617698454,-1.30011046274511));
#55148=CARTESIAN_POINT('Ctrl Pts',(-6.4164139206185,1.79732303197884,0.387245651336726));
#55149=CARTESIAN_POINT('Ctrl Pts',(-6.30526757574106,0.649290547434899,
1.72010204952278));
#55150=CARTESIAN_POINT('Ctrl Pts',(-6.19412123086365,-1.09312773280473,
1.4783101959785));
#55151=CARTESIAN_POINT('Ctrl Pts',(-6.08297488598622,-1.83485441230099,
-0.11678425159416));
#55152=CARTESIAN_POINT('Ctrl Pts',(-5.9718285411088,-0.896884068407809,
-1.60496985753535));
#55153=CARTESIAN_POINT('Ctrl Pts',(-5.86068219623137,0.862128800674478,
-1.62390369382189));
#55154=CARTESIAN_POINT('Ctrl Pts',(-5.74953585135396,1.83191546708753,-0.156252991031506));
#55155=CARTESIAN_POINT('Ctrl Pts',(-5.63838950647652,1.12469553475403,1.45443777105284));
#55156=CARTESIAN_POINT('Ctrl Pts',(-5.5272431615991,-0.612114390813121,
1.73367968446316));
#55157=CARTESIAN_POINT('Ctrl Pts',(-5.41609681672168,-1.78857101895803,
0.42584385155156));
#55158=CARTESIAN_POINT('Ctrl Pts',(-5.30495047184425,-1.32770024034866,
-1.2718259894887));
#55159=CARTESIAN_POINT('Ctrl Pts',(-5.19380412696683,0.348598926865315,
-1.80521690218908));
#55160=CARTESIAN_POINT('Ctrl Pts',(-5.08265778208941,1.70577709140633,-0.686042119839725));
#55161=CARTESIAN_POINT('Ctrl Pts',(-4.97151143721198,1.50142062748163,1.06116227558912));
#55162=CARTESIAN_POINT('Ctrl Pts',(-4.86036509233456,-0.0773946174390751,
1.83693749184676));
#55163=CARTESIAN_POINT('Ctrl Pts',(-4.74921874745714,-1.58535982234177,
0.931108752759484));
#55164=CARTESIAN_POINT('Ctrl Pts',(-4.63807240257972,-1.64202504576567,
-0.827093117393093));
#55165=CARTESIAN_POINT('Ctrl Pts',(-4.52692605770229,-0.195516740427347,
-1.82814181068467));
#55166=CARTESIAN_POINT('Ctrl Pts',(-4.41577971282487,1.42997518601849,-1.15563845692861));
#55167=CARTESIAN_POINT('Ctrl Pts',(-4.30463336794744,1.74641226463907,0.57478124332561));
#55168=CARTESIAN_POINT('Ctrl Pts',(-4.19348702307002,0.464115698312818,
1.77902385996933));
#55169=CARTESIAN_POINT('Ctrl Pts',(-4.0823406781926,-1.24305041174318,1.35467891015794));
#55170=CARTESIAN_POINT('Ctrl Pts',(-3.97119433331518,-1.81227987541939,
-0.309791750874438));
#55171=CARTESIAN_POINT('Ctrl Pts',(-3.86004798843775,-0.72247792391575,
-1.69066700601096));
#55172=CARTESIAN_POINT('Ctrl Pts',(-3.74890164356033,1.02870839145545,-1.52383999196612));
#55173=CARTESIAN_POINT('Ctrl Pts',(-3.63775529868291,1.83817507420302,0.0379693604454949));
#55174=CARTESIAN_POINT('Ctrl Pts',(-3.52660895380548,0.964904870636465,
1.56502008497577));
#55175=CARTESIAN_POINT('Ctrl Pts',(-3.41546260892806,-0.791676743481206,
1.65939061393862));
#55176=CARTESIAN_POINT('Ctrl Pts',(-3.30431626405063,-1.82352670551695,
0.234690498257847));
#55177=CARTESIAN_POINT('Ctrl Pts',(-3.19316991917321,-1.18604946714455,
-1.4048544185183));
#55178=CARTESIAN_POINT('Ctrl Pts',(-3.08202357429579,0.537183538203758,
-1.75834101421655));
#55179=CARTESIAN_POINT('Ctrl Pts',(-2.97087722941836,1.76865785992407,-0.502173923924951));
#55180=CARTESIAN_POINT('Ctrl Pts',(-2.85973088454094,1.38103405472633,1.21370268825252));
#55181=CARTESIAN_POINT('Ctrl Pts',(-2.74858453966351,-0.27084198568111,
1.81850870111212));
#55182=CARTESIAN_POINT('Ctrl Pts',(-2.6374381947861,-1.67477874751467,0.758581188481656));
#55183=CARTESIAN_POINT('Ctrl Pts',(-2.52629184990866,-1.54555797153453,
-0.995781016843169));
#55184=CARTESIAN_POINT('Ctrl Pts',(-2.41514550503125,-0.00147337065513613,
-1.83856659218734));
#55185=CARTESIAN_POINT('Ctrl Pts',(-2.30399916015382,1.54396000303022,-0.998256861862604));
#55186=CARTESIAN_POINT('Ctrl Pts',(-2.1928528152764,1.67599241355422,0.755895971373255));
#55187=CARTESIAN_POINT('Ctrl Pts',(-2.08170647039897,0.273756218286524,
1.81807229264321));
#55188=CARTESIAN_POINT('Ctrl Pts',(-1.97056012552155,-1.3790870015043,1.21591453592819));
#55189=CARTESIAN_POINT('Ctrl Pts',(-1.85941378064413,-1.7694604988402,-0.499338519812307));
#55190=CARTESIAN_POINT('Ctrl Pts',(-1.74826743576671,-0.540000904300196,
-1.75747790595217));
#55191=CARTESIAN_POINT('Ctrl Pts',(-1.63712109088928,1.1837961238493,-1.40675332292743));
#55192=CARTESIAN_POINT('Ctrl Pts',(-1.52597474601186,1.82390089883899,0.231767139453362));
#55193=CARTESIAN_POINT('Ctrl Pts',(-1.41482840113443,0.794334560776014,
1.65812042680182));
#55194=CARTESIAN_POINT('Ctrl Pts',(-1.30368205625701,-0.962393908646208,
1.56656305209763));
#55195=CARTESIAN_POINT('Ctrl Pts',(-1.19253571137958,-1.83811452642306,
0.040918308674494));
#55196=CARTESIAN_POINT('Ctrl Pts',(-1.08138936650216,-1.03114431372679,
-1.52219476242003));
#55197=CARTESIAN_POINT('Ctrl Pts',(-0.970243021624738,0.719757641542406,
-1.69181235504817));
#55198=CARTESIAN_POINT('Ctrl Pts',(-0.859096676747318,1.81179939867516,
-0.312715794767707));
#55199=CARTESIAN_POINT('Ctrl Pts',(-0.747950331869893,1.24518507479472,
1.35272260350057));
#55200=CARTESIAN_POINT('Ctrl Pts',(-0.636803986992467,-0.461197325722433,
1.77969367544763));
#55201=CARTESIAN_POINT('Ctrl Pts',(-0.525657642115045,-1.74561524756276,
0.57771607784515));
#55202=CARTESIAN_POINT('Ctrl Pts',(-0.41451129723762,-1.43158483572782,
-1.15360505340423));
#55203=CARTESIAN_POINT('Ctrl Pts',(-0.303364952360201,0.192127214812409,
-1.82795620083171));
#55204=CARTESIAN_POINT('Ctrl Pts',(-0.192218607482774,1.64158261001566,
-0.830686659357144));
#55205=CARTESIAN_POINT('Ctrl Pts',(-0.0810722626053533,1.5850655110515,
0.930553177147139));
#55206=CARTESIAN_POINT('Ctrl Pts',(-0.00697469935373359,0.584755680233683,
1.53141103236355));
#55207=CARTESIAN_POINT('Ctrl Pts',(0.0300740822720735,0.067969652080238,
1.55401427805413));
#55208=CARTESIAN_POINT('Ctrl Pts',(-0.199999999999991,0.0853826423429707,
1.9521336543348));
#55209=CARTESIAN_POINT('Ctrl Pts',(-0.237048781625799,0.734562905288549,
1.92373973464384));
#55210=CARTESIAN_POINT('Ctrl Pts',(-0.274097563251607,1.36285136861803,
1.54634460475229));
#55211=CARTESIAN_POINT('Ctrl Pts',(-0.311146344877415,1.68882828124029,
0.988905730417313));
#55212=CARTESIAN_POINT('Ctrl Pts',(-0.348195126503225,2.01480519386257,
0.431466856082309));
#55213=CARTESIAN_POINT('Ctrl Pts',(-0.385243908129031,2.03847055577757,
-0.306015762696088));
#55214=CARTESIAN_POINT('Ctrl Pts',(-0.422292689754841,1.74683855847221,
-0.883550030838296));
#55215=CARTESIAN_POINT('Ctrl Pts',(-0.459341471380647,1.45520656116689,
-1.46108429898044));
#55216=CARTESIAN_POINT('Ctrl Pts',(-0.496390253006459,0.848277204641205,
-1.87867021648642));
#55217=CARTESIAN_POINT('Ctrl Pts',(-0.533439034632265,0.204864669659703,
-1.94627790340044));
#55218=CARTESIAN_POINT('Ctrl Pts',(-0.570487816258072,-0.438547865321837,
-2.01388559031446));
#55219=CARTESIAN_POINT('Ctrl Pts',(-0.607536597883876,-1.11844357875923,
-1.73151504663655));
#55220=CARTESIAN_POINT('Ctrl Pts',(-0.644585379509684,-1.52413829337206,
-1.22785238376993));
#55221=CARTESIAN_POINT('Ctrl Pts',(-0.669767022298391,-1.79988445657465,
-0.885518501095601));
#55222=CARTESIAN_POINT('Ctrl Pts',(-0.694948665087098,-1.94895609331017,
-0.440952771968191));
#55223=CARTESIAN_POINT('Ctrl Pts',(-0.720130307875805,-1.95236950710743,
0.00155959742907545));
#55224=CARTESIAN_POINT('Origin',(-0.2,0.,0.));
#55225=CARTESIAN_POINT('',(-0.2,-2.39295984553393E-16,1.954));
#55226=CARTESIAN_POINT('Origin',(-0.2,0.,0.));
#55227=CARTESIAN_POINT('',(0.,-2.6378892053634E-16,2.154));
#55228=CARTESIAN_POINT('Origin',(-0.2,-2.6378892053634E-16,2.154));
#55229=CARTESIAN_POINT('Origin',(0.,0.,0.));
#55230=CARTESIAN_POINT('Origin',(-0.2,0.,0.));
#55231=CARTESIAN_POINT('Origin',(-14.8,0.,0.));
#55232=CARTESIAN_POINT('Origin',(0.,3.5,0.));
#55233=CARTESIAN_POINT('',(-2.77555756156289E-16,-3.5,-4.28626379701574E-16));
#55234=CARTESIAN_POINT('Origin',(0.,0.,0.));
#55235=CARTESIAN_POINT('Origin',(0.3,3.51777354540171,-0.493350061591077));
#55236=CARTESIAN_POINT('',(3.5,3.46093394308575,-0.521475063255119));
#55237=CARTESIAN_POINT('',(0.3,3.46093394308575,-0.521475063255119));
#55238=CARTESIAN_POINT('',(1.8,3.46093394308575,-0.521475063255119));
#55239=CARTESIAN_POINT('',(3.5,3.32865020518126,-0.586930840514225));
#55240=CARTESIAN_POINT('',(3.5,3.51777354540171,-0.493350061591077));
#55241=CARTESIAN_POINT('',(0.3,3.32865020518126,-0.586930840514225));
#55242=CARTESIAN_POINT('',(0.3,3.32865020518126,-0.586930840514225));
#55243=CARTESIAN_POINT('',(0.3,3.51777354540171,-0.493350061591077));
#55244=CARTESIAN_POINT('Origin',(0.3,3.4123588641873,-0.601690935615914));
#55245=CARTESIAN_POINT('',(0.3,3.43056906322043,-0.69368285439016));
#55246=CARTESIAN_POINT('Origin',(0.3,0.,0.));
#55247=CARTESIAN_POINT('',(0.3,3.32865020518126,-0.586930840514225));
#55248=CARTESIAN_POINT('Origin',(0.3,3.32865020518126,-0.586930840514225));
#55249=CARTESIAN_POINT('',(3.5,3.43056906322043,-0.69368285439016));
#55250=CARTESIAN_POINT('',(1.8,3.43056906322043,-0.69368285439016));
#55251=CARTESIAN_POINT('',(3.5,3.32865020518126,-0.586930840514225));
#55252=CARTESIAN_POINT('Origin',(3.5,3.4123588641873,-0.601690935615914));
#55253=CARTESIAN_POINT('Origin',(3.5,0.,0.));
#55254=CARTESIAN_POINT('Origin',(0.3,3.37866132170568,-1.09670993120789));
#55255=CARTESIAN_POINT('',(3.5,3.31780138538096,-1.11453755753864));
#55256=CARTESIAN_POINT('',(0.3,3.31780138538096,-1.11453755753864));
#55257=CARTESIAN_POINT('',(1.8,3.31780138538096,-1.11453755753864));
#55258=CARTESIAN_POINT('',(3.5,3.17616105825637,-1.15602808444076));
#55259=CARTESIAN_POINT('',(3.5,3.37866132170568,-1.09670993120789));
#55260=CARTESIAN_POINT('',(0.3,3.17616105825637,-1.15602808444076));
#55261=CARTESIAN_POINT('',(0.3,3.17616105825637,-1.15602808444076));
#55262=CARTESIAN_POINT('',(0.3,3.37866132170568,-1.09670993120789));
#55263=CARTESIAN_POINT('Origin',(0.3,3.25603493102317,-1.18509979662344));
#55264=CARTESIAN_POINT('',(0.3,3.25799424715966,-1.27885631932385));
#55265=CARTESIAN_POINT('Origin',(0.3,0.,0.));
#55266=CARTESIAN_POINT('',(0.3,3.17616105825637,-1.15602808444076));
#55267=CARTESIAN_POINT('Origin',(0.3,3.17616105825637,-1.15602808444076));
#55268=CARTESIAN_POINT('',(3.5,3.25799424715966,-1.27885631932385));
#55269=CARTESIAN_POINT('',(1.8,3.25799424715966,-1.27885631932385));
#55270=CARTESIAN_POINT('',(3.5,3.17616105825637,-1.15602808444076));
#55271=CARTESIAN_POINT('Origin',(3.5,3.25603493102317,-1.18509979662344));
#55272=CARTESIAN_POINT('Origin',(3.5,0.,0.));
#55273=CARTESIAN_POINT('Origin',(0.3,3.13689018343476,-1.66674682452695));
#55274=CARTESIAN_POINT('',(3.5,3.07385911146988,-1.67373539211956));
#55275=CARTESIAN_POINT('',(0.3,3.07385911146988,-1.67373539211956));
#55276=CARTESIAN_POINT('',(1.8,3.07385911146988,-1.67373539211956));
#55277=CARTESIAN_POINT('',(3.5,2.9271658647914,-1.69));
#55278=CARTESIAN_POINT('',(3.5,3.13689018343476,-1.66674682452695));
#55279=CARTESIAN_POINT('',(0.3,2.9271658647914,-1.69));
#55280=CARTESIAN_POINT('',(0.3,2.9271658647914,-1.69));
#55281=CARTESIAN_POINT('',(0.3,3.13689018343476,-1.66674682452695));
#55282=CARTESIAN_POINT('Origin',(0.3,3.00077802411308,-1.7325));
#55283=CARTESIAN_POINT('',(0.3,2.98642692452359,-1.8251723821274));
#55284=CARTESIAN_POINT('Origin',(0.3,0.,0.));
#55285=CARTESIAN_POINT('',(0.3,2.9271658647914,-1.69));
#55286=CARTESIAN_POINT('Origin',(0.3,2.9271658647914,-1.69));
#55287=CARTESIAN_POINT('',(3.5,2.98642692452359,-1.8251723821274));
#55288=CARTESIAN_POINT('',(1.8,2.98642692452358,-1.8251723821274));
#55289=CARTESIAN_POINT('',(3.5,2.9271658647914,-1.69));
#55290=CARTESIAN_POINT('Origin',(3.5,3.00077802411308,-1.7325));
#55291=CARTESIAN_POINT('Origin',(3.5,0.,0.));
#55292=CARTESIAN_POINT('Origin',(0.3,2.79980622428319,-2.18614045899734));
#55293=CARTESIAN_POINT('',(3.5,2.73651918390454,-2.18207762376191));
#55294=CARTESIAN_POINT('',(0.3,2.73651918390454,-2.18207762376191));
#55295=CARTESIAN_POINT('',(1.8,2.73651918390454,-2.18207762376191));
#55296=CARTESIAN_POINT('',(3.5,2.58923021774214,-2.1726221207405));
#55297=CARTESIAN_POINT('',(3.5,2.79980622428319,-2.18614045899734));
#55298=CARTESIAN_POINT('',(0.3,2.58923021774214,-2.1726221207405));
#55299=CARTESIAN_POINT('',(0.3,2.58923021774214,-2.1726221207405));
#55300=CARTESIAN_POINT('',(0.3,2.79980622428319,-2.18614045899734));
#55301=CARTESIAN_POINT('Origin',(0.3,2.65434399540726,-2.22725906756386));
#55302=CARTESIAN_POINT('',(0.3,2.6241185309908,-2.3160315056818));
#55303=CARTESIAN_POINT('Origin',(0.3,0.,0.));
#55304=CARTESIAN_POINT('',(0.3,2.58923021774214,-2.1726221207405));
#55305=CARTESIAN_POINT('Origin',(0.3,2.58923021774214,-2.1726221207405));
#55306=CARTESIAN_POINT('',(3.5,2.6241185309908,-2.3160315056818));
#55307=CARTESIAN_POINT('',(1.8,2.6241185309908,-2.3160315056818));
#55308=CARTESIAN_POINT('',(3.5,2.58923021774214,-2.1726221207405));
#55309=CARTESIAN_POINT('Origin',(3.5,2.65434399540726,-2.22725906756386));
#55310=CARTESIAN_POINT('Origin',(3.5,0.,0.));
#55311=CARTESIAN_POINT('Origin',(0.3,2.37765156977709,-2.63910932186155));
#55312=CARTESIAN_POINT('',(3.5,2.3160315056818,-2.6241185309908));
#55313=CARTESIAN_POINT('',(0.3,2.3160315056818,-2.6241185309908));
#55314=CARTESIAN_POINT('',(1.8,2.3160315056818,-2.6241185309908));
#55315=CARTESIAN_POINT('',(3.5,2.1726221207405,-2.58923021774215));
#55316=CARTESIAN_POINT('',(3.5,2.37765156977709,-2.63910932186155));
#55317=CARTESIAN_POINT('',(0.3,2.1726221207405,-2.58923021774215));
#55318=CARTESIAN_POINT('',(0.3,2.1726221207405,-2.58923021774215));
#55319=CARTESIAN_POINT('',(0.3,2.37765156977709,-2.63910932186155));
#55320=CARTESIAN_POINT('Origin',(0.3,2.22725906756386,-2.65434399540726));
#55321=CARTESIAN_POINT('',(0.3,2.1820776237619,-2.73651918390455));
#55322=CARTESIAN_POINT('Origin',(0.3,0.,0.));
#55323=CARTESIAN_POINT('',(0.3,2.1726221207405,-2.58923021774215));
#55324=CARTESIAN_POINT('Origin',(0.3,2.1726221207405,-2.58923021774215));
#55325=CARTESIAN_POINT('',(3.5,2.1820776237619,-2.73651918390455));
#55326=CARTESIAN_POINT('',(1.8,2.1820776237619,-2.73651918390455));
#55327=CARTESIAN_POINT('',(3.5,2.1726221207405,-2.58923021774215));
#55328=CARTESIAN_POINT('Origin',(3.5,2.22725906756386,-2.65434399540726));
#55329=CARTESIAN_POINT('Origin',(3.5,0.,0.));
#55330=CARTESIAN_POINT('Origin',(0.3,1.88325317547306,-3.01189018343476));
#55331=CARTESIAN_POINT('',(3.5,1.8251723821274,-2.98642692452359));
#55332=CARTESIAN_POINT('',(0.3,1.8251723821274,-2.98642692452359));
#55333=CARTESIAN_POINT('',(1.8,1.8251723821274,-2.98642692452359));
#55334=CARTESIAN_POINT('',(3.5,1.69,-2.9271658647914));
#55335=CARTESIAN_POINT('',(3.5,1.88325317547306,-3.01189018343476));
#55336=CARTESIAN_POINT('',(0.3,1.69,-2.9271658647914));
#55337=CARTESIAN_POINT('',(0.3,1.69,-2.9271658647914));
#55338=CARTESIAN_POINT('',(0.3,1.88325317547306,-3.01189018343476));
#55339=CARTESIAN_POINT('Origin',(0.3,1.7325,-3.00077802411308));
#55340=CARTESIAN_POINT('',(0.3,1.67373539211956,-3.07385911146988));
#55341=CARTESIAN_POINT('Origin',(0.3,0.,0.));
#55342=CARTESIAN_POINT('',(0.3,1.69,-2.9271658647914));
#55343=CARTESIAN_POINT('Origin',(0.3,1.69,-2.9271658647914));
#55344=CARTESIAN_POINT('',(3.5,1.67373539211956,-3.07385911146988));
#55345=CARTESIAN_POINT('',(1.8,1.67373539211956,-3.07385911146988));
#55346=CARTESIAN_POINT('',(3.5,1.69,-2.9271658647914));
#55347=CARTESIAN_POINT('Origin',(3.5,1.7325,-3.00077802411308));
#55348=CARTESIAN_POINT('Origin',(3.5,0.,0.));
#55349=CARTESIAN_POINT('Origin',(0.3,1.33163308640436,-3.29315628587427));
#55350=CARTESIAN_POINT('',(3.5,1.27885631932384,-3.25799424715967));
#55351=CARTESIAN_POINT('',(0.3,1.27885631932384,-3.25799424715967));
#55352=CARTESIAN_POINT('',(1.8,1.27885631932384,-3.25799424715967));
#55353=CARTESIAN_POINT('',(3.5,1.15602808444076,-3.17616105825637));
#55354=CARTESIAN_POINT('',(3.5,1.33163308640436,-3.29315628587427));
#55355=CARTESIAN_POINT('',(0.3,1.15602808444076,-3.17616105825637));
#55356=CARTESIAN_POINT('',(0.3,1.15602808444076,-3.17616105825637));
#55357=CARTESIAN_POINT('',(0.3,1.33163308640436,-3.29315628587427));
#55358=CARTESIAN_POINT('Origin',(0.3,1.18509979662344,-3.25603493102317));
#55359=CARTESIAN_POINT('',(0.3,1.11453755753863,-3.31780138538096));
#55360=CARTESIAN_POINT('Origin',(0.3,0.,0.));
#55361=CARTESIAN_POINT('',(0.3,1.15602808444076,-3.17616105825637));
#55362=CARTESIAN_POINT('Origin',(0.3,1.15602808444076,-3.17616105825637));
#55363=CARTESIAN_POINT('',(3.5,1.11453755753863,-3.31780138538096));
#55364=CARTESIAN_POINT('',(1.8,1.11453755753863,-3.31780138538096));
#55365=CARTESIAN_POINT('',(3.5,1.15602808444076,-3.17616105825637));
#55366=CARTESIAN_POINT('Origin',(3.5,1.18509979662344,-3.25603493102317));
#55367=CARTESIAN_POINT('Origin',(3.5,0.,0.));
#55368=CARTESIAN_POINT('Origin',(0.3,0.739551999844127,-3.47436150098497));
#55369=CARTESIAN_POINT('',(3.5,0.693682854390159,-3.43056906322043));
#55370=CARTESIAN_POINT('',(0.3,0.693682854390159,-3.43056906322043));
#55371=CARTESIAN_POINT('',(1.8,0.693682854390159,-3.43056906322043));
#55372=CARTESIAN_POINT('',(3.5,0.586930840514223,-3.32865020518126));
#55373=CARTESIAN_POINT('',(3.5,0.739551999844127,-3.47436150098497));
#55374=CARTESIAN_POINT('',(0.3,0.586930840514223,-3.32865020518126));
#55375=CARTESIAN_POINT('',(0.3,0.586930840514223,-3.32865020518126));
#55376=CARTESIAN_POINT('',(0.3,0.739551999844127,-3.47436150098497));
#55377=CARTESIAN_POINT('Origin',(0.3,0.601690935615912,-3.4123588641873));
#55378=CARTESIAN_POINT('',(0.3,0.521475063255118,-3.46093394308575));
#55379=CARTESIAN_POINT('Origin',(0.3,0.,0.));
#55380=CARTESIAN_POINT('',(0.3,0.586930840514223,-3.32865020518126));
#55381=CARTESIAN_POINT('Origin',(0.3,0.586930840514223,-3.32865020518126));
#55382=CARTESIAN_POINT('',(3.5,0.521475063255118,-3.46093394308575));
#55383=CARTESIAN_POINT('',(1.8,0.521475063255118,-3.46093394308575));
#55384=CARTESIAN_POINT('',(3.5,0.586930840514223,-3.32865020518126));
#55385=CARTESIAN_POINT('Origin',(3.5,0.601690935615912,-3.4123588641873));
#55386=CARTESIAN_POINT('Origin',(3.5,0.,0.));
#55387=CARTESIAN_POINT('Origin',(0.3,0.124999999999999,-3.55));
#55388=CARTESIAN_POINT('',(3.5,0.0874321869462905,-3.49890777424696));
#55389=CARTESIAN_POINT('',(0.3,0.0874321869462905,-3.49890777424696));
#55390=CARTESIAN_POINT('',(1.8,0.0874321869462905,-3.49890777424696));
#55391=CARTESIAN_POINT('',(3.5,-6.20895927167708E-16,-3.38));
#55392=CARTESIAN_POINT('',(3.5,0.124999999999999,-3.55));
#55393=CARTESIAN_POINT('',(0.3,-6.20895927167708E-16,-3.38));
#55394=CARTESIAN_POINT('',(0.3,-6.20895927167708E-16,-3.38));
#55395=CARTESIAN_POINT('',(0.3,0.124999999999999,-3.55));
#55396=CARTESIAN_POINT('Origin',(0.3,-6.36510173856837E-16,-3.465));
#55397=CARTESIAN_POINT('',(0.3,-0.0874321869462918,-3.49890777424696));
#55398=CARTESIAN_POINT('Origin',(0.3,0.,0.));
#55399=CARTESIAN_POINT('',(0.3,-6.20895927167708E-16,-3.38));
#55400=CARTESIAN_POINT('Origin',(0.3,-6.20895927167708E-16,-3.38));
#55401=CARTESIAN_POINT('',(3.5,-0.0874321869462918,-3.49890777424696));
#55402=CARTESIAN_POINT('',(1.8,-0.0874321869462921,-3.49890777424696));
#55403=CARTESIAN_POINT('',(3.5,-6.20895927167708E-16,-3.38));
#55404=CARTESIAN_POINT('Origin',(3.5,-6.36510173856837E-16,-3.465));
#55405=CARTESIAN_POINT('Origin',(3.5,0.,0.));
#55406=CARTESIAN_POINT('Origin',(0.3,-0.493350061591077,-3.51777354540171));
#55407=CARTESIAN_POINT('',(3.5,-0.521475063255118,-3.46093394308575));
#55408=CARTESIAN_POINT('',(0.3,-0.521475063255118,-3.46093394308575));
#55409=CARTESIAN_POINT('',(1.8,-0.521475063255118,-3.46093394308575));
#55410=CARTESIAN_POINT('',(3.5,-0.586930840514225,-3.32865020518126));
#55411=CARTESIAN_POINT('',(3.5,-0.493350061591077,-3.51777354540171));
#55412=CARTESIAN_POINT('',(0.3,-0.586930840514225,-3.32865020518126));
#55413=CARTESIAN_POINT('',(0.3,-0.586930840514225,-3.32865020518126));
#55414=CARTESIAN_POINT('',(0.3,-0.493350061591077,-3.51777354540171));
#55415=CARTESIAN_POINT('Origin',(0.3,-0.601690935615914,-3.4123588641873));
#55416=CARTESIAN_POINT('',(0.3,-0.693682854390159,-3.43056906322043));
#55417=CARTESIAN_POINT('Origin',(0.3,0.,0.));
#55418=CARTESIAN_POINT('',(0.3,-0.586930840514225,-3.32865020518126));
#55419=CARTESIAN_POINT('Origin',(0.3,-0.586930840514225,-3.32865020518126));
#55420=CARTESIAN_POINT('',(3.5,-0.693682854390159,-3.43056906322043));
#55421=CARTESIAN_POINT('',(1.8,-0.69368285439016,-3.43056906322043));
#55422=CARTESIAN_POINT('',(3.5,-0.586930840514225,-3.32865020518126));
#55423=CARTESIAN_POINT('Origin',(3.5,-0.601690935615914,-3.4123588641873));
#55424=CARTESIAN_POINT('Origin',(3.5,0.,0.));
#55425=CARTESIAN_POINT('Origin',(0.3,-1.09670993120789,-3.37866132170568));
#55426=CARTESIAN_POINT('',(3.5,-1.11453755753864,-3.31780138538096));
#55427=CARTESIAN_POINT('',(0.3,-1.11453755753864,-3.31780138538096));
#55428=CARTESIAN_POINT('',(1.8,-1.11453755753864,-3.31780138538096));
#55429=CARTESIAN_POINT('',(3.5,-1.15602808444076,-3.17616105825637));
#55430=CARTESIAN_POINT('',(3.5,-1.09670993120789,-3.37866132170568));
#55431=CARTESIAN_POINT('',(0.3,-1.15602808444076,-3.17616105825637));
#55432=CARTESIAN_POINT('',(0.3,-1.15602808444076,-3.17616105825637));
#55433=CARTESIAN_POINT('',(0.3,-1.09670993120789,-3.37866132170568));
#55434=CARTESIAN_POINT('Origin',(0.3,-1.18509979662344,-3.25603493102317));
#55435=CARTESIAN_POINT('',(0.3,-1.27885631932385,-3.25799424715966));
#55436=CARTESIAN_POINT('Origin',(0.3,0.,0.));
#55437=CARTESIAN_POINT('',(0.3,-1.15602808444076,-3.17616105825637));
#55438=CARTESIAN_POINT('Origin',(0.3,-1.15602808444076,-3.17616105825637));
#55439=CARTESIAN_POINT('',(3.5,-1.27885631932385,-3.25799424715966));
#55440=CARTESIAN_POINT('',(1.8,-1.27885631932385,-3.25799424715966));
#55441=CARTESIAN_POINT('',(3.5,-1.15602808444076,-3.17616105825637));
#55442=CARTESIAN_POINT('Origin',(3.5,-1.18509979662344,-3.25603493102317));
#55443=CARTESIAN_POINT('Origin',(3.5,0.,0.));
#55444=CARTESIAN_POINT('Origin',(0.3,-1.66674682452695,-3.13689018343476));
#55445=CARTESIAN_POINT('',(3.5,-1.67373539211956,-3.07385911146988));
#55446=CARTESIAN_POINT('',(0.3,-1.67373539211956,-3.07385911146988));
#55447=CARTESIAN_POINT('',(1.8,-1.67373539211956,-3.07385911146988));
#55448=CARTESIAN_POINT('',(3.5,-1.69,-2.9271658647914));
#55449=CARTESIAN_POINT('',(3.5,-1.66674682452695,-3.13689018343476));
#55450=CARTESIAN_POINT('',(0.3,-1.69,-2.9271658647914));
#55451=CARTESIAN_POINT('',(0.3,-1.69,-2.9271658647914));
#55452=CARTESIAN_POINT('',(0.3,-1.66674682452695,-3.13689018343476));
#55453=CARTESIAN_POINT('Origin',(0.3,-1.7325,-3.00077802411308));
#55454=CARTESIAN_POINT('',(0.3,-1.8251723821274,-2.98642692452359));
#55455=CARTESIAN_POINT('Origin',(0.3,0.,0.));
#55456=CARTESIAN_POINT('',(0.3,-1.69,-2.9271658647914));
#55457=CARTESIAN_POINT('Origin',(0.3,-1.69,-2.9271658647914));
#55458=CARTESIAN_POINT('',(3.5,-1.8251723821274,-2.98642692452359));
#55459=CARTESIAN_POINT('',(1.8,-1.8251723821274,-2.98642692452358));
#55460=CARTESIAN_POINT('',(3.5,-1.69,-2.9271658647914));
#55461=CARTESIAN_POINT('Origin',(3.5,-1.7325,-3.00077802411308));
#55462=CARTESIAN_POINT('Origin',(3.5,0.,0.));
#55463=CARTESIAN_POINT('Origin',(0.3,-2.18614045899734,-2.79980622428319));
#55464=CARTESIAN_POINT('',(3.5,-2.1820776237619,-2.73651918390454));
#55465=CARTESIAN_POINT('',(0.3,-2.1820776237619,-2.73651918390454));
#55466=CARTESIAN_POINT('',(1.8,-2.1820776237619,-2.73651918390454));
#55467=CARTESIAN_POINT('',(3.5,-2.1726221207405,-2.58923021774214));
#55468=CARTESIAN_POINT('',(3.5,-2.18614045899734,-2.79980622428319));
#55469=CARTESIAN_POINT('',(0.3,-2.1726221207405,-2.58923021774214));
#55470=CARTESIAN_POINT('',(0.3,-2.1726221207405,-2.58923021774214));
#55471=CARTESIAN_POINT('',(0.3,-2.18614045899734,-2.79980622428319));
#55472=CARTESIAN_POINT('Origin',(0.3,-2.22725906756386,-2.65434399540726));
#55473=CARTESIAN_POINT('',(0.3,-2.3160315056818,-2.6241185309908));
#55474=CARTESIAN_POINT('Origin',(0.3,0.,0.));
#55475=CARTESIAN_POINT('',(0.3,-2.1726221207405,-2.58923021774214));
#55476=CARTESIAN_POINT('Origin',(0.3,-2.1726221207405,-2.58923021774214));
#55477=CARTESIAN_POINT('',(3.5,-2.3160315056818,-2.6241185309908));
#55478=CARTESIAN_POINT('',(1.8,-2.3160315056818,-2.6241185309908));
#55479=CARTESIAN_POINT('',(3.5,-2.1726221207405,-2.58923021774214));
#55480=CARTESIAN_POINT('Origin',(3.5,-2.22725906756386,-2.65434399540726));
#55481=CARTESIAN_POINT('Origin',(3.5,0.,0.));
#55482=CARTESIAN_POINT('Origin',(0.3,-2.63910932186155,-2.37765156977709));
#55483=CARTESIAN_POINT('',(3.5,-2.6241185309908,-2.3160315056818));
#55484=CARTESIAN_POINT('',(0.3,-2.6241185309908,-2.3160315056818));
#55485=CARTESIAN_POINT('',(1.8,-2.6241185309908,-2.3160315056818));
#55486=CARTESIAN_POINT('',(3.5,-2.58923021774215,-2.1726221207405));
#55487=CARTESIAN_POINT('',(3.5,-2.63910932186155,-2.37765156977709));
#55488=CARTESIAN_POINT('',(0.3,-2.58923021774215,-2.1726221207405));
#55489=CARTESIAN_POINT('',(0.3,-2.58923021774215,-2.1726221207405));
#55490=CARTESIAN_POINT('',(0.3,-2.63910932186155,-2.37765156977709));
#55491=CARTESIAN_POINT('Origin',(0.3,-2.65434399540726,-2.22725906756386));
#55492=CARTESIAN_POINT('',(0.3,-2.73651918390455,-2.1820776237619));
#55493=CARTESIAN_POINT('Origin',(0.3,0.,0.));
#55494=CARTESIAN_POINT('',(0.3,-2.58923021774215,-2.1726221207405));
#55495=CARTESIAN_POINT('Origin',(0.3,-2.58923021774215,-2.1726221207405));
#55496=CARTESIAN_POINT('',(3.5,-2.73651918390455,-2.1820776237619));
#55497=CARTESIAN_POINT('',(1.8,-2.73651918390455,-2.1820776237619));
#55498=CARTESIAN_POINT('',(3.5,-2.58923021774215,-2.1726221207405));
#55499=CARTESIAN_POINT('Origin',(3.5,-2.65434399540726,-2.22725906756386));
#55500=CARTESIAN_POINT('Origin',(3.5,0.,0.));
#55501=CARTESIAN_POINT('Origin',(0.3,-3.01189018343476,-1.88325317547305));
#55502=CARTESIAN_POINT('',(3.5,-2.98642692452359,-1.8251723821274));
#55503=CARTESIAN_POINT('',(0.3,-2.98642692452359,-1.8251723821274));
#55504=CARTESIAN_POINT('',(1.8,-2.98642692452359,-1.8251723821274));
#55505=CARTESIAN_POINT('',(3.5,-2.9271658647914,-1.69));
#55506=CARTESIAN_POINT('',(3.5,-3.01189018343476,-1.88325317547305));
#55507=CARTESIAN_POINT('',(0.3,-2.9271658647914,-1.69));
#55508=CARTESIAN_POINT('',(0.3,-2.9271658647914,-1.69));
#55509=CARTESIAN_POINT('',(0.3,-3.01189018343476,-1.88325317547305));
#55510=CARTESIAN_POINT('Origin',(0.3,-3.00077802411308,-1.7325));
#55511=CARTESIAN_POINT('',(0.3,-3.07385911146988,-1.67373539211956));
#55512=CARTESIAN_POINT('Origin',(0.3,0.,0.));
#55513=CARTESIAN_POINT('',(0.3,-2.9271658647914,-1.69));
#55514=CARTESIAN_POINT('Origin',(0.3,-2.9271658647914,-1.69));
#55515=CARTESIAN_POINT('',(3.5,-3.07385911146988,-1.67373539211956));
#55516=CARTESIAN_POINT('',(1.8,-3.07385911146988,-1.67373539211956));
#55517=CARTESIAN_POINT('',(3.5,-2.9271658647914,-1.69));
#55518=CARTESIAN_POINT('Origin',(3.5,-3.00077802411308,-1.7325));
#55519=CARTESIAN_POINT('Origin',(3.5,0.,0.));
#55520=CARTESIAN_POINT('Origin',(0.3,-3.29315628587427,-1.33163308640436));
#55521=CARTESIAN_POINT('',(3.5,-3.25799424715966,-1.27885631932384));
#55522=CARTESIAN_POINT('',(0.3,-3.25799424715966,-1.27885631932384));
#55523=CARTESIAN_POINT('',(1.8,-3.25799424715966,-1.27885631932384));
#55524=CARTESIAN_POINT('',(3.5,-3.17616105825637,-1.15602808444076));
#55525=CARTESIAN_POINT('',(3.5,-3.29315628587427,-1.33163308640436));
#55526=CARTESIAN_POINT('',(0.3,-3.17616105825637,-1.15602808444076));
#55527=CARTESIAN_POINT('',(0.3,-3.17616105825637,-1.15602808444076));
#55528=CARTESIAN_POINT('',(0.3,-3.29315628587427,-1.33163308640436));
#55529=CARTESIAN_POINT('Origin',(0.3,-3.25603493102317,-1.18509979662344));
#55530=CARTESIAN_POINT('',(0.3,-3.31780138538096,-1.11453755753864));
#55531=CARTESIAN_POINT('Origin',(0.3,0.,0.));
#55532=CARTESIAN_POINT('',(0.3,-3.17616105825637,-1.15602808444076));
#55533=CARTESIAN_POINT('Origin',(0.3,-3.17616105825637,-1.15602808444076));
#55534=CARTESIAN_POINT('',(3.5,-3.31780138538096,-1.11453755753864));
#55535=CARTESIAN_POINT('',(1.8,-3.31780138538096,-1.11453755753864));
#55536=CARTESIAN_POINT('',(3.5,-3.17616105825637,-1.15602808444076));
#55537=CARTESIAN_POINT('Origin',(3.5,-3.25603493102317,-1.18509979662344));
#55538=CARTESIAN_POINT('Origin',(3.5,0.,0.));
#55539=CARTESIAN_POINT('Origin',(0.3,-3.47436150098497,-0.739551999844128));
#55540=CARTESIAN_POINT('',(3.5,-3.43056906322043,-0.693682854390159));
#55541=CARTESIAN_POINT('',(0.3,-3.43056906322043,-0.693682854390159));
#55542=CARTESIAN_POINT('',(1.8,-3.43056906322043,-0.693682854390159));
#55543=CARTESIAN_POINT('',(3.5,-3.32865020518126,-0.586930840514224));
#55544=CARTESIAN_POINT('',(3.5,-3.47436150098497,-0.739551999844128));
#55545=CARTESIAN_POINT('',(0.3,-3.32865020518126,-0.586930840514224));
#55546=CARTESIAN_POINT('',(0.3,-3.32865020518126,-0.586930840514224));
#55547=CARTESIAN_POINT('',(0.3,-3.47436150098497,-0.739551999844128));
#55548=CARTESIAN_POINT('Origin',(0.3,-3.4123588641873,-0.601690935615913));
#55549=CARTESIAN_POINT('',(0.3,-3.46093394308575,-0.521475063255118));
#55550=CARTESIAN_POINT('Origin',(0.3,0.,0.));
#55551=CARTESIAN_POINT('',(0.3,-3.32865020518126,-0.586930840514224));
#55552=CARTESIAN_POINT('Origin',(0.3,-3.32865020518126,-0.586930840514224));
#55553=CARTESIAN_POINT('',(3.5,-3.46093394308575,-0.521475063255118));
#55554=CARTESIAN_POINT('',(1.8,-3.46093394308575,-0.521475063255118));
#55555=CARTESIAN_POINT('',(3.5,-3.32865020518126,-0.586930840514224));
#55556=CARTESIAN_POINT('Origin',(3.5,-3.4123588641873,-0.601690935615913));
#55557=CARTESIAN_POINT('Origin',(3.5,0.,0.));
#55558=CARTESIAN_POINT('Origin',(0.3,-3.55,-0.125));
#55559=CARTESIAN_POINT('',(3.5,-3.49890777424696,-0.087432186946291));
#55560=CARTESIAN_POINT('',(0.3,-3.49890777424696,-0.087432186946291));
#55561=CARTESIAN_POINT('',(1.8,-3.49890777424696,-0.087432186946291));
#55562=CARTESIAN_POINT('',(3.5,-3.38,4.13930618111805E-16));
#55563=CARTESIAN_POINT('',(3.5,-3.55,-0.125));
#55564=CARTESIAN_POINT('',(0.3,-3.38,4.13930618111805E-16));
#55565=CARTESIAN_POINT('',(0.3,-3.38,4.13930618111805E-16));
#55566=CARTESIAN_POINT('',(0.3,-3.55,-0.125));
#55567=CARTESIAN_POINT('Origin',(0.3,-3.465,4.24340115904558E-16));
#55568=CARTESIAN_POINT('',(0.3,-3.5,-4.28626379701574E-16));
#55569=CARTESIAN_POINT('Origin',(0.3,0.,0.));
#55570=CARTESIAN_POINT('',(0.3,-3.49890777424696,0.0874321869462918));
#55571=CARTESIAN_POINT('',(0.3,-3.38,4.13930618111805E-16));
#55572=CARTESIAN_POINT('Origin',(0.3,0.,0.));
#55573=CARTESIAN_POINT('Origin',(0.3,-3.38,4.13930618111805E-16));
#55574=CARTESIAN_POINT('',(3.5,-3.49890777424696,0.0874321869462918));
#55575=CARTESIAN_POINT('',(1.8,-3.49890777424696,0.0874321869462913));
#55576=CARTESIAN_POINT('',(3.5,-3.38,4.13930618111805E-16));
#55577=CARTESIAN_POINT('Origin',(3.5,-3.465,4.24340115904558E-16));
#55578=CARTESIAN_POINT('',(3.5,-3.5,-4.28626379701574E-16));
#55579=CARTESIAN_POINT('Origin',(3.5,0.,0.));
#55580=CARTESIAN_POINT('Origin',(3.5,0.,0.));
#55581=CARTESIAN_POINT('Origin',(0.3,-3.5177735454017,0.493350061591078));
#55582=CARTESIAN_POINT('',(3.5,-3.46093394308575,0.52147506325512));
#55583=CARTESIAN_POINT('',(0.3,-3.46093394308575,0.52147506325512));
#55584=CARTESIAN_POINT('',(1.8,-3.46093394308575,0.52147506325512));
#55585=CARTESIAN_POINT('',(3.5,-3.32865020518126,0.586930840514226));
#55586=CARTESIAN_POINT('',(3.5,-3.5177735454017,0.493350061591078));
#55587=CARTESIAN_POINT('',(0.3,-3.32865020518126,0.586930840514226));
#55588=CARTESIAN_POINT('',(0.3,-3.32865020518126,0.586930840514226));
#55589=CARTESIAN_POINT('',(0.3,-3.5177735454017,0.493350061591078));
#55590=CARTESIAN_POINT('Origin',(0.3,-3.4123588641873,0.601690935615915));
#55591=CARTESIAN_POINT('',(0.3,-3.43056906322043,0.693682854390161));
#55592=CARTESIAN_POINT('Origin',(0.3,0.,0.));
#55593=CARTESIAN_POINT('',(0.3,-3.32865020518126,0.586930840514226));
#55594=CARTESIAN_POINT('Origin',(0.3,-3.32865020518126,0.586930840514226));
#55595=CARTESIAN_POINT('',(3.5,-3.43056906322043,0.693682854390161));
#55596=CARTESIAN_POINT('',(1.8,-3.43056906322043,0.693682854390161));
#55597=CARTESIAN_POINT('',(3.5,-3.32865020518126,0.586930840514226));
#55598=CARTESIAN_POINT('Origin',(3.5,-3.4123588641873,0.601690935615915));
#55599=CARTESIAN_POINT('Origin',(3.5,0.,0.));
#55600=CARTESIAN_POINT('Origin',(0.3,-3.37866132170568,1.09670993120789));
#55601=CARTESIAN_POINT('',(3.5,-3.31780138538096,1.11453755753864));
#55602=CARTESIAN_POINT('',(0.3,-3.31780138538096,1.11453755753864));
#55603=CARTESIAN_POINT('',(1.8,-3.31780138538096,1.11453755753864));
#55604=CARTESIAN_POINT('',(3.5,-3.17616105825637,1.15602808444076));
#55605=CARTESIAN_POINT('',(3.5,-3.37866132170568,1.09670993120789));
#55606=CARTESIAN_POINT('',(0.3,-3.17616105825637,1.15602808444076));
#55607=CARTESIAN_POINT('',(0.3,-3.17616105825637,1.15602808444076));
#55608=CARTESIAN_POINT('',(0.3,-3.37866132170568,1.09670993120789));
#55609=CARTESIAN_POINT('Origin',(0.3,-3.25603493102317,1.18509979662344));
#55610=CARTESIAN_POINT('',(0.3,-3.25799424715966,1.27885631932384));
#55611=CARTESIAN_POINT('Origin',(0.3,0.,0.));
#55612=CARTESIAN_POINT('',(0.3,-3.17616105825637,1.15602808444076));
#55613=CARTESIAN_POINT('Origin',(0.3,-3.17616105825637,1.15602808444076));
#55614=CARTESIAN_POINT('',(3.5,-3.25799424715966,1.27885631932384));
#55615=CARTESIAN_POINT('',(1.8,-3.25799424715966,1.27885631932384));
#55616=CARTESIAN_POINT('',(3.5,-3.17616105825637,1.15602808444076));
#55617=CARTESIAN_POINT('Origin',(3.5,-3.25603493102317,1.18509979662344));
#55618=CARTESIAN_POINT('Origin',(3.5,0.,0.));
#55619=CARTESIAN_POINT('Origin',(0.3,-3.13689018343476,1.66674682452694));
#55620=CARTESIAN_POINT('',(3.5,-3.07385911146988,1.67373539211956));
#55621=CARTESIAN_POINT('',(0.3,-3.07385911146988,1.67373539211956));
#55622=CARTESIAN_POINT('',(1.8,-3.07385911146988,1.67373539211956));
#55623=CARTESIAN_POINT('',(3.5,-2.9271658647914,1.69));
#55624=CARTESIAN_POINT('',(3.5,-3.13689018343476,1.66674682452694));
#55625=CARTESIAN_POINT('',(0.3,-2.9271658647914,1.69));
#55626=CARTESIAN_POINT('',(0.3,-2.9271658647914,1.69));
#55627=CARTESIAN_POINT('',(0.3,-3.13689018343476,1.66674682452694));
#55628=CARTESIAN_POINT('Origin',(0.3,-3.00077802411308,1.7325));
#55629=CARTESIAN_POINT('',(0.3,-2.98642692452359,1.8251723821274));
#55630=CARTESIAN_POINT('Origin',(0.3,0.,0.));
#55631=CARTESIAN_POINT('',(0.3,-2.9271658647914,1.69));
#55632=CARTESIAN_POINT('Origin',(0.3,-2.9271658647914,1.69));
#55633=CARTESIAN_POINT('',(3.5,-2.98642692452359,1.8251723821274));
#55634=CARTESIAN_POINT('',(1.8,-2.98642692452359,1.8251723821274));
#55635=CARTESIAN_POINT('',(3.5,-2.9271658647914,1.69));
#55636=CARTESIAN_POINT('Origin',(3.5,-3.00077802411308,1.7325));
#55637=CARTESIAN_POINT('Origin',(3.5,0.,0.));
#55638=CARTESIAN_POINT('Origin',(0.3,-2.79980622428319,2.18614045899734));
#55639=CARTESIAN_POINT('',(3.5,-2.73651918390454,2.1820776237619));
#55640=CARTESIAN_POINT('',(0.3,-2.73651918390454,2.1820776237619));
#55641=CARTESIAN_POINT('',(1.8,-2.73651918390454,2.1820776237619));
#55642=CARTESIAN_POINT('',(3.5,-2.58923021774214,2.1726221207405));
#55643=CARTESIAN_POINT('',(3.5,-2.79980622428319,2.18614045899734));
#55644=CARTESIAN_POINT('',(0.3,-2.58923021774214,2.1726221207405));
#55645=CARTESIAN_POINT('',(0.3,-2.58923021774214,2.1726221207405));
#55646=CARTESIAN_POINT('',(0.3,-2.79980622428319,2.18614045899734));
#55647=CARTESIAN_POINT('Origin',(0.3,-2.65434399540726,2.22725906756386));
#55648=CARTESIAN_POINT('',(0.3,-2.6241185309908,2.3160315056818));
#55649=CARTESIAN_POINT('Origin',(0.3,0.,0.));
#55650=CARTESIAN_POINT('',(0.3,-2.58923021774214,2.1726221207405));
#55651=CARTESIAN_POINT('Origin',(0.3,-2.58923021774214,2.1726221207405));
#55652=CARTESIAN_POINT('',(3.5,-2.6241185309908,2.3160315056818));
#55653=CARTESIAN_POINT('',(1.8,-2.6241185309908,2.3160315056818));
#55654=CARTESIAN_POINT('',(3.5,-2.58923021774214,2.1726221207405));
#55655=CARTESIAN_POINT('Origin',(3.5,-2.65434399540726,2.22725906756386));
#55656=CARTESIAN_POINT('Origin',(3.5,0.,0.));
#55657=CARTESIAN_POINT('Origin',(0.3,-2.37765156977709,2.63910932186155));
#55658=CARTESIAN_POINT('',(3.5,-2.3160315056818,2.6241185309908));
#55659=CARTESIAN_POINT('',(0.3,-2.3160315056818,2.6241185309908));
#55660=CARTESIAN_POINT('',(1.8,-2.3160315056818,2.6241185309908));
#55661=CARTESIAN_POINT('',(3.5,-2.1726221207405,2.58923021774215));
#55662=CARTESIAN_POINT('',(3.5,-2.37765156977709,2.63910932186155));
#55663=CARTESIAN_POINT('',(0.3,-2.1726221207405,2.58923021774215));
#55664=CARTESIAN_POINT('',(0.3,-2.1726221207405,2.58923021774215));
#55665=CARTESIAN_POINT('',(0.3,-2.37765156977709,2.63910932186155));
#55666=CARTESIAN_POINT('Origin',(0.3,-2.22725906756386,2.65434399540726));
#55667=CARTESIAN_POINT('',(0.3,-2.1820776237619,2.73651918390455));
#55668=CARTESIAN_POINT('Origin',(0.3,0.,0.));
#55669=CARTESIAN_POINT('',(0.3,-2.1726221207405,2.58923021774215));
#55670=CARTESIAN_POINT('Origin',(0.3,-2.1726221207405,2.58923021774215));
#55671=CARTESIAN_POINT('',(3.5,-2.1820776237619,2.73651918390455));
#55672=CARTESIAN_POINT('',(1.8,-2.1820776237619,2.73651918390455));
#55673=CARTESIAN_POINT('',(3.5,-2.1726221207405,2.58923021774215));
#55674=CARTESIAN_POINT('Origin',(3.5,-2.22725906756386,2.65434399540726));
#55675=CARTESIAN_POINT('Origin',(3.5,0.,0.));
#55676=CARTESIAN_POINT('Origin',(0.3,-1.88325317547305,3.01189018343476));
#55677=CARTESIAN_POINT('',(3.5,-1.8251723821274,2.98642692452359));
#55678=CARTESIAN_POINT('',(0.3,-1.8251723821274,2.98642692452359));
#55679=CARTESIAN_POINT('',(1.8,-1.8251723821274,2.98642692452359));
#55680=CARTESIAN_POINT('',(3.5,-1.69,2.9271658647914));
#55681=CARTESIAN_POINT('',(3.5,-1.88325317547305,3.01189018343476));
#55682=CARTESIAN_POINT('',(0.3,-1.69,2.9271658647914));
#55683=CARTESIAN_POINT('',(0.3,-1.69,2.9271658647914));
#55684=CARTESIAN_POINT('',(0.3,-1.88325317547305,3.01189018343476));
#55685=CARTESIAN_POINT('Origin',(0.3,-1.7325,3.00077802411308));
#55686=CARTESIAN_POINT('',(0.3,-1.67373539211956,3.07385911146988));
#55687=CARTESIAN_POINT('Origin',(0.3,0.,0.));
#55688=CARTESIAN_POINT('',(0.3,-1.69,2.9271658647914));
#55689=CARTESIAN_POINT('Origin',(0.3,-1.69,2.9271658647914));
#55690=CARTESIAN_POINT('',(3.5,-1.67373539211956,3.07385911146988));
#55691=CARTESIAN_POINT('',(1.8,-1.67373539211956,3.07385911146988));
#55692=CARTESIAN_POINT('',(3.5,-1.69,2.9271658647914));
#55693=CARTESIAN_POINT('Origin',(3.5,-1.7325,3.00077802411308));
#55694=CARTESIAN_POINT('Origin',(3.5,0.,0.));
#55695=CARTESIAN_POINT('Origin',(0.3,-1.33163308640436,3.29315628587427));
#55696=CARTESIAN_POINT('',(3.5,-1.27885631932384,3.25799424715966));
#55697=CARTESIAN_POINT('',(0.3,-1.27885631932384,3.25799424715966));
#55698=CARTESIAN_POINT('',(1.8,-1.27885631932384,3.25799424715966));
#55699=CARTESIAN_POINT('',(3.5,-1.15602808444076,3.17616105825637));
#55700=CARTESIAN_POINT('',(3.5,-1.33163308640436,3.29315628587427));
#55701=CARTESIAN_POINT('',(0.3,-1.15602808444076,3.17616105825637));
#55702=CARTESIAN_POINT('',(0.3,-1.15602808444076,3.17616105825637));
#55703=CARTESIAN_POINT('',(0.3,-1.33163308640436,3.29315628587427));
#55704=CARTESIAN_POINT('Origin',(0.3,-1.18509979662344,3.25603493102317));
#55705=CARTESIAN_POINT('',(0.3,-1.11453755753864,3.31780138538096));
#55706=CARTESIAN_POINT('Origin',(0.3,0.,0.));
#55707=CARTESIAN_POINT('',(0.3,-1.15602808444076,3.17616105825637));
#55708=CARTESIAN_POINT('Origin',(0.3,-1.15602808444076,3.17616105825637));
#55709=CARTESIAN_POINT('',(3.5,-1.11453755753864,3.31780138538096));
#55710=CARTESIAN_POINT('',(1.8,-1.11453755753864,3.31780138538096));
#55711=CARTESIAN_POINT('',(3.5,-1.15602808444076,3.17616105825637));
#55712=CARTESIAN_POINT('Origin',(3.5,-1.18509979662344,3.25603493102317));
#55713=CARTESIAN_POINT('Origin',(3.5,0.,0.));
#55714=CARTESIAN_POINT('Origin',(0.3,-0.739551999844129,3.47436150098497));
#55715=CARTESIAN_POINT('',(3.5,-0.69368285439016,3.43056906322043));
#55716=CARTESIAN_POINT('',(0.3,-0.69368285439016,3.43056906322043));
#55717=CARTESIAN_POINT('',(1.8,-0.69368285439016,3.43056906322043));
#55718=CARTESIAN_POINT('',(3.5,-0.586930840514225,3.32865020518126));
#55719=CARTESIAN_POINT('',(3.5,-0.739551999844129,3.47436150098497));
#55720=CARTESIAN_POINT('',(0.3,-0.586930840514225,3.32865020518126));
#55721=CARTESIAN_POINT('',(0.3,-0.586930840514225,3.32865020518126));
#55722=CARTESIAN_POINT('',(0.3,-0.739551999844129,3.47436150098497));
#55723=CARTESIAN_POINT('Origin',(0.3,-0.601690935615914,3.4123588641873));
#55724=CARTESIAN_POINT('',(0.3,-0.521475063255119,3.46093394308575));
#55725=CARTESIAN_POINT('Origin',(0.3,0.,0.));
#55726=CARTESIAN_POINT('',(0.3,-0.586930840514225,3.32865020518126));
#55727=CARTESIAN_POINT('Origin',(0.3,-0.586930840514225,3.32865020518126));
#55728=CARTESIAN_POINT('',(3.5,-0.521475063255119,3.46093394308575));
#55729=CARTESIAN_POINT('',(1.8,-0.521475063255119,3.46093394308575));
#55730=CARTESIAN_POINT('',(3.5,-0.586930840514225,3.32865020518126));
#55731=CARTESIAN_POINT('Origin',(3.5,-0.601690935615914,3.4123588641873));
#55732=CARTESIAN_POINT('Origin',(3.5,0.,0.));
#55733=CARTESIAN_POINT('Origin',(0.3,-0.125,3.55));
#55734=CARTESIAN_POINT('',(3.5,-0.0874321869462913,3.49890777424696));
#55735=CARTESIAN_POINT('',(0.3,-0.0874321869462913,3.49890777424696));
#55736=CARTESIAN_POINT('',(1.8,-0.0874321869462916,3.49890777424696));
#55737=CARTESIAN_POINT('',(3.5,2.06965309055903E-16,3.38));
#55738=CARTESIAN_POINT('',(3.5,-0.125,3.55));
#55739=CARTESIAN_POINT('',(0.3,2.06965309055903E-16,3.38));
#55740=CARTESIAN_POINT('',(0.3,2.06965309055903E-16,3.38));
#55741=CARTESIAN_POINT('',(0.3,-0.125,3.55));
#55742=CARTESIAN_POINT('Origin',(0.3,2.12170057952279E-16,3.465));
#55743=CARTESIAN_POINT('',(0.3,0.0874321869462921,3.49890777424696));
#55744=CARTESIAN_POINT('Origin',(0.3,0.,0.));
#55745=CARTESIAN_POINT('',(0.3,2.06965309055903E-16,3.38));
#55746=CARTESIAN_POINT('Origin',(0.3,2.06965309055903E-16,3.38));
#55747=CARTESIAN_POINT('',(3.5,0.0874321869462921,3.49890777424696));
#55748=CARTESIAN_POINT('',(1.8,0.0874321869462918,3.49890777424696));
#55749=CARTESIAN_POINT('',(3.5,2.06965309055903E-16,3.38));
#55750=CARTESIAN_POINT('Origin',(3.5,2.12170057952279E-16,3.465));
#55751=CARTESIAN_POINT('Origin',(3.5,0.,0.));
#55752=CARTESIAN_POINT('Origin',(0.3,0.493350061591077,3.51777354540171));
#55753=CARTESIAN_POINT('',(3.5,0.521475063255119,3.46093394308575));
#55754=CARTESIAN_POINT('',(0.3,0.521475063255119,3.46093394308575));
#55755=CARTESIAN_POINT('',(1.8,0.521475063255119,3.46093394308575));
#55756=CARTESIAN_POINT('',(3.5,0.586930840514225,3.32865020518126));
#55757=CARTESIAN_POINT('',(3.5,0.493350061591077,3.51777354540171));
#55758=CARTESIAN_POINT('',(0.3,0.586930840514225,3.32865020518126));
#55759=CARTESIAN_POINT('',(0.3,0.586930840514225,3.32865020518126));
#55760=CARTESIAN_POINT('',(0.3,0.493350061591077,3.51777354540171));
#55761=CARTESIAN_POINT('Origin',(0.3,0.601690935615914,3.4123588641873));
#55762=CARTESIAN_POINT('',(0.3,0.693682854390159,3.43056906322043));
#55763=CARTESIAN_POINT('Origin',(0.3,0.,0.));
#55764=CARTESIAN_POINT('',(0.3,0.586930840514225,3.32865020518126));
#55765=CARTESIAN_POINT('Origin',(0.3,0.586930840514225,3.32865020518126));
#55766=CARTESIAN_POINT('',(3.5,0.693682854390159,3.43056906322043));
#55767=CARTESIAN_POINT('',(1.8,0.693682854390159,3.43056906322043));
#55768=CARTESIAN_POINT('',(3.5,0.586930840514225,3.32865020518126));
#55769=CARTESIAN_POINT('Origin',(3.5,0.601690935615914,3.4123588641873));
#55770=CARTESIAN_POINT('Origin',(3.5,0.,0.));
#55771=CARTESIAN_POINT('Origin',(0.3,1.09670993120789,3.37866132170568));
#55772=CARTESIAN_POINT('',(3.5,1.11453755753864,3.31780138538096));
#55773=CARTESIAN_POINT('',(0.3,1.11453755753864,3.31780138538096));
#55774=CARTESIAN_POINT('',(1.8,1.11453755753864,3.31780138538096));
#55775=CARTESIAN_POINT('',(3.5,1.15602808444076,3.17616105825637));
#55776=CARTESIAN_POINT('',(3.5,1.09670993120789,3.37866132170568));
#55777=CARTESIAN_POINT('',(0.3,1.15602808444076,3.17616105825637));
#55778=CARTESIAN_POINT('',(0.3,1.15602808444076,3.17616105825637));
#55779=CARTESIAN_POINT('',(0.3,1.09670993120789,3.37866132170568));
#55780=CARTESIAN_POINT('Origin',(0.3,1.18509979662344,3.25603493102317));
#55781=CARTESIAN_POINT('',(0.3,1.27885631932384,3.25799424715966));
#55782=CARTESIAN_POINT('Origin',(0.3,0.,0.));
#55783=CARTESIAN_POINT('',(0.3,1.15602808444076,3.17616105825637));
#55784=CARTESIAN_POINT('Origin',(0.3,1.15602808444076,3.17616105825637));
#55785=CARTESIAN_POINT('',(3.5,1.27885631932384,3.25799424715966));
#55786=CARTESIAN_POINT('',(1.8,1.27885631932384,3.25799424715966));
#55787=CARTESIAN_POINT('',(3.5,1.15602808444076,3.17616105825637));
#55788=CARTESIAN_POINT('Origin',(3.5,1.18509979662344,3.25603493102317));
#55789=CARTESIAN_POINT('Origin',(3.5,0.,0.));
#55790=CARTESIAN_POINT('Origin',(0.3,1.66674682452695,3.13689018343476));
#55791=CARTESIAN_POINT('',(3.5,1.67373539211956,3.07385911146988));
#55792=CARTESIAN_POINT('',(0.3,1.67373539211956,3.07385911146988));
#55793=CARTESIAN_POINT('',(1.8,1.67373539211956,3.07385911146988));
#55794=CARTESIAN_POINT('',(3.5,1.69,2.9271658647914));
#55795=CARTESIAN_POINT('',(3.5,1.66674682452695,3.13689018343476));
#55796=CARTESIAN_POINT('',(0.3,1.69,2.9271658647914));
#55797=CARTESIAN_POINT('',(0.3,1.69,2.9271658647914));
#55798=CARTESIAN_POINT('',(0.3,1.66674682452695,3.13689018343476));
#55799=CARTESIAN_POINT('Origin',(0.3,1.7325,3.00077802411308));
#55800=CARTESIAN_POINT('',(0.3,1.8251723821274,2.98642692452359));
#55801=CARTESIAN_POINT('Origin',(0.3,0.,0.));
#55802=CARTESIAN_POINT('',(0.3,1.69,2.9271658647914));
#55803=CARTESIAN_POINT('Origin',(0.3,1.69,2.9271658647914));
#55804=CARTESIAN_POINT('',(3.5,1.8251723821274,2.98642692452359));
#55805=CARTESIAN_POINT('',(1.8,1.8251723821274,2.98642692452359));
#55806=CARTESIAN_POINT('',(3.5,1.69,2.9271658647914));
#55807=CARTESIAN_POINT('Origin',(3.5,1.7325,3.00077802411308));
#55808=CARTESIAN_POINT('Origin',(3.5,0.,0.));
#55809=CARTESIAN_POINT('Origin',(0.3,2.18614045899734,2.79980622428319));
#55810=CARTESIAN_POINT('',(3.5,2.1820776237619,2.73651918390455));
#55811=CARTESIAN_POINT('',(0.3,2.1820776237619,2.73651918390455));
#55812=CARTESIAN_POINT('',(1.8,2.1820776237619,2.73651918390455));
#55813=CARTESIAN_POINT('',(3.5,2.1726221207405,2.58923021774215));
#55814=CARTESIAN_POINT('',(3.5,2.18614045899734,2.79980622428319));
#55815=CARTESIAN_POINT('',(0.3,2.1726221207405,2.58923021774215));
#55816=CARTESIAN_POINT('',(0.3,2.1726221207405,2.58923021774215));
#55817=CARTESIAN_POINT('',(0.3,2.18614045899734,2.79980622428319));
#55818=CARTESIAN_POINT('Origin',(0.3,2.22725906756386,2.65434399540726));
#55819=CARTESIAN_POINT('',(0.3,2.3160315056818,2.6241185309908));
#55820=CARTESIAN_POINT('Origin',(0.3,0.,0.));
#55821=CARTESIAN_POINT('',(0.3,2.1726221207405,2.58923021774215));
#55822=CARTESIAN_POINT('Origin',(0.3,2.1726221207405,2.58923021774215));
#55823=CARTESIAN_POINT('',(3.5,2.3160315056818,2.6241185309908));
#55824=CARTESIAN_POINT('',(1.8,2.3160315056818,2.6241185309908));
#55825=CARTESIAN_POINT('',(3.5,2.1726221207405,2.58923021774215));
#55826=CARTESIAN_POINT('Origin',(3.5,2.22725906756386,2.65434399540726));
#55827=CARTESIAN_POINT('Origin',(3.5,0.,0.));
#55828=CARTESIAN_POINT('Origin',(0.3,2.63910932186155,2.37765156977709));
#55829=CARTESIAN_POINT('',(3.5,2.6241185309908,2.3160315056818));
#55830=CARTESIAN_POINT('',(0.3,2.6241185309908,2.3160315056818));
#55831=CARTESIAN_POINT('',(1.8,2.6241185309908,2.3160315056818));
#55832=CARTESIAN_POINT('',(3.5,2.58923021774215,2.1726221207405));
#55833=CARTESIAN_POINT('',(3.5,2.63910932186155,2.37765156977709));
#55834=CARTESIAN_POINT('',(0.3,2.58923021774215,2.1726221207405));
#55835=CARTESIAN_POINT('',(0.3,2.58923021774215,2.1726221207405));
#55836=CARTESIAN_POINT('',(0.3,2.63910932186155,2.37765156977709));
#55837=CARTESIAN_POINT('Origin',(0.3,2.65434399540726,2.22725906756386));
#55838=CARTESIAN_POINT('',(0.3,2.73651918390455,2.1820776237619));
#55839=CARTESIAN_POINT('Origin',(0.3,0.,0.));
#55840=CARTESIAN_POINT('',(0.3,2.58923021774215,2.1726221207405));
#55841=CARTESIAN_POINT('Origin',(0.3,2.58923021774215,2.1726221207405));
#55842=CARTESIAN_POINT('',(3.5,2.73651918390455,2.1820776237619));
#55843=CARTESIAN_POINT('',(1.8,2.73651918390455,2.1820776237619));
#55844=CARTESIAN_POINT('',(3.5,2.58923021774215,2.1726221207405));
#55845=CARTESIAN_POINT('Origin',(3.5,2.65434399540726,2.22725906756386));
#55846=CARTESIAN_POINT('Origin',(3.5,0.,0.));
#55847=CARTESIAN_POINT('Origin',(0.3,3.01189018343476,1.88325317547305));
#55848=CARTESIAN_POINT('',(3.5,2.98642692452359,1.8251723821274));
#55849=CARTESIAN_POINT('',(0.3,2.98642692452359,1.8251723821274));
#55850=CARTESIAN_POINT('',(1.8,2.98642692452359,1.8251723821274));
#55851=CARTESIAN_POINT('',(3.5,2.9271658647914,1.69));
#55852=CARTESIAN_POINT('',(3.5,3.01189018343476,1.88325317547305));
#55853=CARTESIAN_POINT('',(0.3,2.9271658647914,1.69));
#55854=CARTESIAN_POINT('',(0.3,2.9271658647914,1.69));
#55855=CARTESIAN_POINT('',(0.3,3.01189018343476,1.88325317547305));
#55856=CARTESIAN_POINT('Origin',(0.3,3.00077802411308,1.7325));
#55857=CARTESIAN_POINT('',(0.3,3.07385911146988,1.67373539211956));
#55858=CARTESIAN_POINT('Origin',(0.3,0.,0.));
#55859=CARTESIAN_POINT('',(0.3,2.9271658647914,1.69));
#55860=CARTESIAN_POINT('Origin',(0.3,2.9271658647914,1.69));
#55861=CARTESIAN_POINT('',(3.5,3.07385911146988,1.67373539211956));
#55862=CARTESIAN_POINT('',(1.8,3.07385911146988,1.67373539211956));
#55863=CARTESIAN_POINT('',(3.5,2.9271658647914,1.69));
#55864=CARTESIAN_POINT('Origin',(3.5,3.00077802411308,1.7325));
#55865=CARTESIAN_POINT('Origin',(3.5,0.,0.));
#55866=CARTESIAN_POINT('Origin',(0.3,3.29315628587427,1.33163308640436));
#55867=CARTESIAN_POINT('',(3.5,3.25799424715966,1.27885631932384));
#55868=CARTESIAN_POINT('',(0.3,3.25799424715966,1.27885631932384));
#55869=CARTESIAN_POINT('',(1.8,3.25799424715966,1.27885631932384));
#55870=CARTESIAN_POINT('',(3.5,3.17616105825637,1.15602808444076));
#55871=CARTESIAN_POINT('',(3.5,3.29315628587427,1.33163308640436));
#55872=CARTESIAN_POINT('',(0.3,3.17616105825637,1.15602808444076));
#55873=CARTESIAN_POINT('',(0.3,3.17616105825637,1.15602808444076));
#55874=CARTESIAN_POINT('',(0.3,3.29315628587427,1.33163308640436));
#55875=CARTESIAN_POINT('Origin',(0.3,3.25603493102317,1.18509979662344));
#55876=CARTESIAN_POINT('',(0.3,3.31780138538096,1.11453755753864));
#55877=CARTESIAN_POINT('Origin',(0.3,0.,0.));
#55878=CARTESIAN_POINT('',(0.3,3.17616105825637,1.15602808444076));
#55879=CARTESIAN_POINT('Origin',(0.3,3.17616105825637,1.15602808444076));
#55880=CARTESIAN_POINT('',(3.5,3.31780138538096,1.11453755753864));
#55881=CARTESIAN_POINT('',(1.8,3.31780138538096,1.11453755753864));
#55882=CARTESIAN_POINT('',(3.5,3.17616105825637,1.15602808444076));
#55883=CARTESIAN_POINT('Origin',(3.5,3.25603493102317,1.18509979662344));
#55884=CARTESIAN_POINT('Origin',(3.5,0.,0.));
#55885=CARTESIAN_POINT('Origin',(0.3,3.47436150098497,0.739551999844129));
#55886=CARTESIAN_POINT('',(3.5,3.43056906322043,0.69368285439016));
#55887=CARTESIAN_POINT('',(0.3,3.43056906322043,0.69368285439016));
#55888=CARTESIAN_POINT('',(1.8,3.43056906322043,0.69368285439016));
#55889=CARTESIAN_POINT('',(3.5,3.32865020518126,0.586930840514225));
#55890=CARTESIAN_POINT('',(3.5,3.47436150098497,0.739551999844129));
#55891=CARTESIAN_POINT('',(0.3,3.32865020518126,0.586930840514225));
#55892=CARTESIAN_POINT('',(0.3,3.32865020518126,0.586930840514225));
#55893=CARTESIAN_POINT('',(0.3,3.47436150098497,0.739551999844129));
#55894=CARTESIAN_POINT('Origin',(0.3,3.4123588641873,0.601690935615914));
#55895=CARTESIAN_POINT('',(0.3,3.46093394308575,0.521475063255119));
#55896=CARTESIAN_POINT('Origin',(0.3,0.,0.));
#55897=CARTESIAN_POINT('',(0.3,3.32865020518126,0.586930840514225));
#55898=CARTESIAN_POINT('Origin',(0.3,3.32865020518126,0.586930840514225));
#55899=CARTESIAN_POINT('',(3.5,3.46093394308575,0.521475063255119));
#55900=CARTESIAN_POINT('',(1.8,3.46093394308575,0.521475063255119));
#55901=CARTESIAN_POINT('',(3.5,3.32865020518126,0.586930840514225));
#55902=CARTESIAN_POINT('Origin',(3.5,3.4123588641873,0.601690935615914));
#55903=CARTESIAN_POINT('Origin',(3.5,0.,0.));
#55904=CARTESIAN_POINT('Origin',(0.3,3.55,0.125));
#55905=CARTESIAN_POINT('',(3.5,3.49890777424696,0.0874321869462918));
#55906=CARTESIAN_POINT('',(0.3,3.49890777424696,0.0874321869462918));
#55907=CARTESIAN_POINT('',(1.8,3.49890777424696,0.0874321869462916));
#55908=CARTESIAN_POINT('',(3.5,3.38,0.));
#55909=CARTESIAN_POINT('',(3.5,3.55,0.125));
#55910=CARTESIAN_POINT('',(0.3,3.38,0.));
#55911=CARTESIAN_POINT('',(0.3,3.38,0.));
#55912=CARTESIAN_POINT('',(0.3,3.55,0.125));
#55913=CARTESIAN_POINT('Origin',(0.3,3.465,0.));
#55914=CARTESIAN_POINT('',(0.3,3.49890777424696,-0.0874321869462918));
#55915=CARTESIAN_POINT('Origin',(0.3,0.,0.));
#55916=CARTESIAN_POINT('',(0.3,3.38,0.));
#55917=CARTESIAN_POINT('Origin',(0.3,3.38,0.));
#55918=CARTESIAN_POINT('',(3.5,3.49890777424696,-0.0874321869462918));
#55919=CARTESIAN_POINT('',(1.8,3.49890777424696,-0.0874321869462916));
#55920=CARTESIAN_POINT('',(3.5,3.38,0.));
#55921=CARTESIAN_POINT('Origin',(3.5,3.465,0.));
#55922=CARTESIAN_POINT('Origin',(3.5,0.,0.));
#55923=CARTESIAN_POINT('Origin',(1.55435453572933,0.,0.));
#55924=CARTESIAN_POINT('',(1.09870907145866,0.,0.));
#55925=CARTESIAN_POINT('',(2.,-1.483539833954,1.81681230905937E-16));
#55926=CARTESIAN_POINT('',(1.55435453572933,-0.75,-9.18485099360515E-17));
#55927=CARTESIAN_POINT('Origin',(2.,0.,0.));
#55928=CARTESIAN_POINT('Origin',(4.,0.,1.73205080756888));
#55929=CARTESIAN_POINT('',(4.,1.06057523872491E-16,1.73205080756888));
#55930=CARTESIAN_POINT('',(4.,1.5,0.866025403784439));
#55931=CARTESIAN_POINT('',(4.,0.375,1.51554445662277));
#55932=CARTESIAN_POINT('',(2.,0.,1.73205080756888));
#55933=CARTESIAN_POINT('',(4.,1.06057523872491E-16,1.73205080756888));
#55934=CARTESIAN_POINT('',(2.,1.5,0.866025403784439));
#55935=CARTESIAN_POINT('',(2.,1.5,0.866025403784439));
#55936=CARTESIAN_POINT('',(4.,1.5,0.866025403784439));
#55937=CARTESIAN_POINT('Origin',(4.,-1.5,0.866025403784439));
#55938=CARTESIAN_POINT('',(4.,-1.5,0.866025403784439));
#55939=CARTESIAN_POINT('',(4.,-1.125,1.08253175473055));
#55940=CARTESIAN_POINT('',(2.,-1.5,0.866025403784439));
#55941=CARTESIAN_POINT('',(4.,-1.5,0.866025403784439));
#55942=CARTESIAN_POINT('',(2.,1.06057523872491E-16,1.73205080756888));
#55943=CARTESIAN_POINT('Origin',(4.,-1.5,-0.866025403784439));
#55944=CARTESIAN_POINT('',(4.,-1.5,-0.866025403784439));
#55945=CARTESIAN_POINT('',(4.,-1.5,-0.43301270189222));
#55946=CARTESIAN_POINT('',(2.,-1.5,-0.866025403784439));
#55947=CARTESIAN_POINT('',(4.,-1.5,-0.866025403784439));
#55948=CARTESIAN_POINT('',(2.,-1.5,0.866025403784439));
#55949=CARTESIAN_POINT('Origin',(4.,-2.77555756156289E-16,-1.73205080756888));
#55950=CARTESIAN_POINT('',(4.,-3.18172571617472E-16,-1.73205080756888));
#55951=CARTESIAN_POINT('',(4.,-0.375,-1.51554445662277));
#55952=CARTESIAN_POINT('',(2.,-2.77555756156289E-16,-1.73205080756888));
#55953=CARTESIAN_POINT('',(4.,-3.18172571617472E-16,-1.73205080756888));
#55954=CARTESIAN_POINT('',(2.,-1.5,-0.866025403784439));
#55955=CARTESIAN_POINT('Origin',(4.,1.5,-0.866025403784439));
#55956=CARTESIAN_POINT('',(4.,1.5,-0.866025403784439));
#55957=CARTESIAN_POINT('',(4.,1.125,-1.08253175473055));
#55958=CARTESIAN_POINT('',(2.,1.5,-0.866025403784439));
#55959=CARTESIAN_POINT('',(4.,1.5,-0.866025403784439));
#55960=CARTESIAN_POINT('',(2.,-3.18172571617472E-16,-1.73205080756888));
#55961=CARTESIAN_POINT('Origin',(4.,1.5,0.866025403784439));
#55962=CARTESIAN_POINT('',(4.,1.5,0.433012701892219));
#55963=CARTESIAN_POINT('',(2.,1.5,-0.866025403784439));
#55964=CARTESIAN_POINT('Origin',(2.,0.,0.));
#55965=CARTESIAN_POINT('Origin',(-30.,1.6,0.));
#55966=CARTESIAN_POINT('',(-30.,-1.6,-1.95943487863576E-16));
#55967=CARTESIAN_POINT('Origin',(-30.,0.,0.));
#55968=CARTESIAN_POINT('Origin',(-29.8,0.,0.));
#55969=CARTESIAN_POINT('',(-29.8,-1.8,-2.20436423846524E-16));
#55970=CARTESIAN_POINT('Origin',(1.8,0.,0.));
#55971=CARTESIAN_POINT('',(3.6,-3.5,-4.28626379701574E-16));
#55972=CARTESIAN_POINT('Origin',(3.6,0.,0.));
#55973=CARTESIAN_POINT('',(1.8,-3.5,-4.28626379701574E-16));
#55974=CARTESIAN_POINT('',(1.8,-3.5,-4.28626379701574E-16));
#55975=CARTESIAN_POINT('Origin',(3.8,0.,0.));
#55976=CARTESIAN_POINT('',(4.,-3.1,-3.79640507735679E-16));
#55977=CARTESIAN_POINT('Origin',(4.,0.,0.));
#55978=CARTESIAN_POINT('',(3.8,-3.3,-4.04133443718627E-16));
#55979=CARTESIAN_POINT('Origin',(4.,0.,0.));
#82355=UNCERTAINTY_MEASURE_WITH_UNIT(LENGTH_MEASURE(0.01),#82385,
'DISTANCE_ACCURACY_VALUE',
'Maximum model space distance between geometric entities at asserted c
onnectivities');
#82363=UNCERTAINTY_MEASURE_WITH_UNIT(LENGTH_MEASURE(0.01),#82385,
'DISTANCE_ACCURACY_VALUE',
'Maximum model space distance between geometric entities at asserted c
onnectivities');
#82376=(
GEOMETRIC_REPRESENTATION_CONTEXT(3)
GLOBAL_UNCERTAINTY_ASSIGNED_CONTEXT((#82355))
GLOBAL_UNIT_ASSIGNED_CONTEXT((#82385,#82387,#82388))
REPRESENTATION_CONTEXT('','3D')
);
#82384=(
GEOMETRIC_REPRESENTATION_CONTEXT(3)
GLOBAL_UNCERTAINTY_ASSIGNED_CONTEXT((#82363))
GLOBAL_UNIT_ASSIGNED_CONTEXT((#82385,#82387,#82388))
REPRESENTATION_CONTEXT('','3D')
);
#82385=(
LENGTH_UNIT()
NAMED_UNIT(*)
SI_UNIT(.MILLI.,.METRE.)
);
#82387=(
NAMED_UNIT(*)
PLANE_ANGLE_UNIT()
SI_UNIT($,.RADIAN.)
);
#82388=(
NAMED_UNIT(*)
SI_UNIT($,.STERADIAN.)
SOLID_ANGLE_UNIT()
);
#82401=SHAPE_DEFINITION_REPRESENTATION(#82421,#82477);
#82421=PRODUCT_DEFINITION_SHAPE('',$,#82498);
#82477=SHAPE_REPRESENTATION('',(#32107),#82376);
#82485=PRODUCT_DEFINITION_CONTEXT('part definition',#82547,'design');
#82498=PRODUCT_DEFINITION('2026-10-20-12-38-25-351','14_ISO_4762_M4x30',
#82518,#82485);
#82518=PRODUCT_DEFINITION_FORMATION('',$,#82561);
#82547=APPLICATION_CONTEXT(
'Core Data for Automotive Mechanical Design Process');
#82548=PRODUCT_CONTEXT('part definition',#82547,'mechanical');
#82561=PRODUCT('2026-10-20-12-38-25-351','14_ISO_4762_M4x30',$,(#82548));
#82632=COLOUR_RGB('Black',0.12,0.14,0.17);
#82633=FILL_AREA_STYLE_COLOUR('',#82632);
#82634=FILL_AREA_STYLE('',(#82633));
#82635=SURFACE_STYLE_FILL_AREA(#82634);
#82636=SURFACE_SIDE_STYLE('',(#82635));
#82637=SURFACE_STYLE_USAGE(.BOTH.,#82636);
#82638=PRESENTATION_STYLE_ASSIGNMENT((#82637));
ENDSEC;
END-ISO-10303-21;
